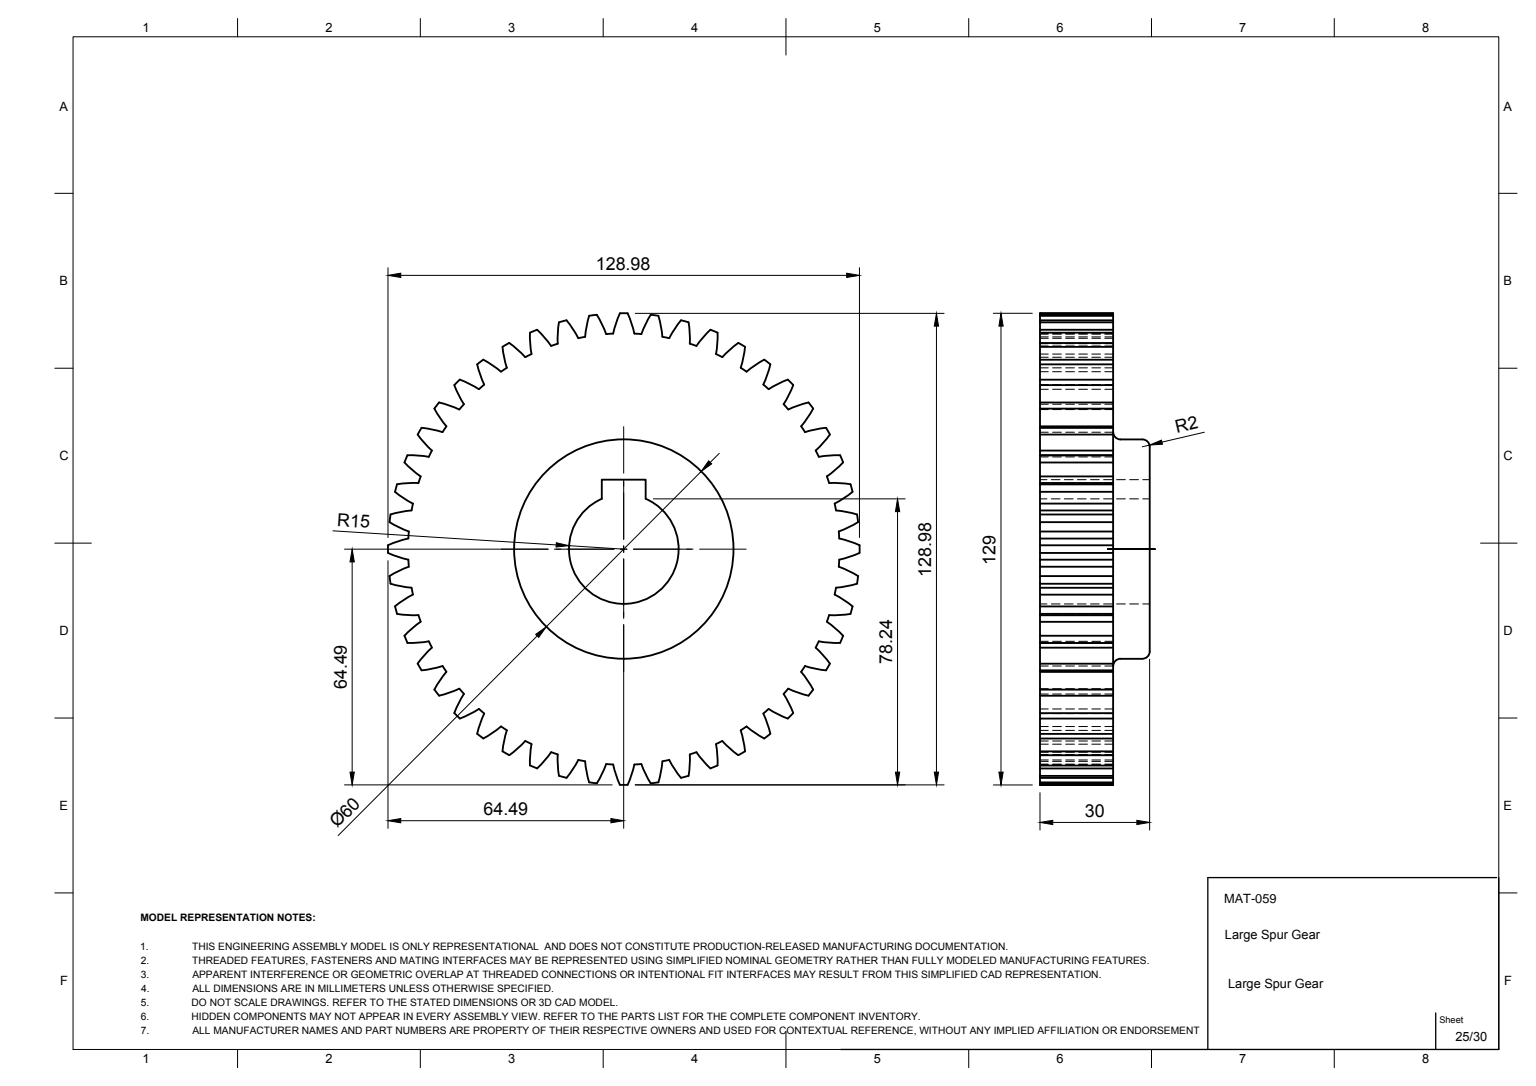
ISO-10303-21;
HEADER;
/* Generated by software containing ST-Developer
 * from STEP Tools, Inc. (www.steptools.com) 
 */

FILE_DESCRIPTION(
/* description */ ('', 'CAx-IF Rec.Pracs.---Representation and Presentation of Product Manufa
cturing Information (PMI)---4.0---2014-10-13'),
/* implementation_level */ '2;1');

FILE_NAME(
/* name */ 'Large Spur Gear.step',
/* time_stamp */ '2026-10-28T23:00:48+01:00',
/* author */ (''),
/* organization */ (''),
/* preprocessor_version */ 'ST-DEVELOPER v20.2',
/* originating_system */ 'Autodesk Translation Framework v15.17.0.0',
/* authorisation */ '');

FILE_SCHEMA (('AP242_MANAGED_MODEL_BASED_3D_ENGINEERING_MIM_LF { 1 0 10303 442 2 1 4 }'));
ENDSEC;

DATA;
#10=MECHANICAL_DESIGN_GEOMETRIC_PRESENTATION_REPRESENTATION('',(#996),#61811);
#906=TOROIDAL_SURFACE('',#36149,28.,2.);
#907=TOROIDAL_SURFACE('',#36158,32.,2.);
#932=SHAPE_REPRESENTATION_RELATIONSHIP('SRR','None',#61993,#957);
#957=ADVANCED_BREP_SHAPE_REPRESENTATION('',(#1035),#61806);
#996=STYLED_ITEM('',(#62149),#1035);
#1035=MANIFOLD_SOLID_BREP('Body1',#33826);
#1395=CYLINDRICAL_SURFACE('',#36154,30.);
#1396=CYLINDRICAL_SURFACE('',#36356,15.);
#1397=CYLINDRICAL_SURFACE('',#36359,59.00430282);
#1398=CYLINDRICAL_SURFACE('',#36361,28.3018268963564);
#1399=CYLINDRICAL_SURFACE('',#36363,28.3018268963564);
#1400=CYLINDRICAL_SURFACE('',#36365,59.00430282);
#1401=CYLINDRICAL_SURFACE('',#36367,28.3018268963564);
#1402=CYLINDRICAL_SURFACE('',#36369,28.3018268963564);
#1403=CYLINDRICAL_SURFACE('',#36371,59.00430282);
#1404=CYLINDRICAL_SURFACE('',#36373,28.3018268963564);
#1405=CYLINDRICAL_SURFACE('',#36375,28.3018268963564);
#1406=CYLINDRICAL_SURFACE('',#36377,59.00430282);
#1407=CYLINDRICAL_SURFACE('',#36379,28.3018268963564);
#1408=CYLINDRICAL_SURFACE('',#36381,28.3018268963564);
#1409=CYLINDRICAL_SURFACE('',#36383,59.00430282);
#1410=CYLINDRICAL_SURFACE('',#36385,28.3018268963564);
#1411=CYLINDRICAL_SURFACE('',#36387,28.3018268963564);
#1412=CYLINDRICAL_SURFACE('',#36389,59.00430282);
#1413=CYLINDRICAL_SURFACE('',#36391,28.3018268963564);
#1414=CYLINDRICAL_SURFACE('',#36393,28.3018268963564);
#1415=CYLINDRICAL_SURFACE('',#36395,59.00430282);
#1416=CYLINDRICAL_SURFACE('',#36397,28.3018268963564);
#1417=CYLINDRICAL_SURFACE('',#36399,28.3018268963564);
#1418=CYLINDRICAL_SURFACE('',#36401,59.00430282);
#1419=CYLINDRICAL_SURFACE('',#36403,28.3018268963564);
#1420=CYLINDRICAL_SURFACE('',#36405,28.3018268963564);
#1421=CYLINDRICAL_SURFACE('',#36407,59.00430282);
#1422=CYLINDRICAL_SURFACE('',#36409,28.3018268963564);
#1423=CYLINDRICAL_SURFACE('',#36411,28.3018268963564);
#1424=CYLINDRICAL_SURFACE('',#36413,59.00430282);
#1425=CYLINDRICAL_SURFACE('',#36415,28.3018268963564);
#1426=CYLINDRICAL_SURFACE('',#36417,28.3018268963564);
#1427=CYLINDRICAL_SURFACE('',#36419,59.00430282);
#1428=CYLINDRICAL_SURFACE('',#36421,28.3018268963564);
#1429=CYLINDRICAL_SURFACE('',#36423,28.3018268963564);
#1430=CYLINDRICAL_SURFACE('',#36425,59.00430282);
#1431=CYLINDRICAL_SURFACE('',#36427,28.3018268963564);
#1432=CYLINDRICAL_SURFACE('',#36429,28.3018268963564);
#1433=CYLINDRICAL_SURFACE('',#36431,59.00430282);
#1434=CYLINDRICAL_SURFACE('',#36433,28.3018268963564);
#1435=CYLINDRICAL_SURFACE('',#36435,28.3018268963564);
#1436=CYLINDRICAL_SURFACE('',#36437,59.00430282);
#1437=CYLINDRICAL_SURFACE('',#36439,28.3018268963564);
#1438=CYLINDRICAL_SURFACE('',#36441,28.3018268963564);
#1439=CYLINDRICAL_SURFACE('',#36443,59.00430282);
#1440=CYLINDRICAL_SURFACE('',#36445,28.3018268963564);
#1441=CYLINDRICAL_SURFACE('',#36447,28.3018268963564);
#1442=CYLINDRICAL_SURFACE('',#36449,59.00430282);
#1443=CYLINDRICAL_SURFACE('',#36451,28.3018268963564);
#1444=CYLINDRICAL_SURFACE('',#36453,28.3018268963564);
#1445=CYLINDRICAL_SURFACE('',#36455,59.00430282);
#1446=CYLINDRICAL_SURFACE('',#36457,28.3018268963564);
#1447=CYLINDRICAL_SURFACE('',#36459,28.3018268963564);
#1448=CYLINDRICAL_SURFACE('',#36461,59.00430282);
#1449=CYLINDRICAL_SURFACE('',#36463,28.3018268963564);
#1450=CYLINDRICAL_SURFACE('',#36465,28.3018268963564);
#1451=CYLINDRICAL_SURFACE('',#36467,59.00430282);
#1452=CYLINDRICAL_SURFACE('',#36469,28.3018268963564);
#1453=CYLINDRICAL_SURFACE('',#36471,28.3018268963564);
#1454=CYLINDRICAL_SURFACE('',#36473,59.00430282);
#1455=CYLINDRICAL_SURFACE('',#36475,28.3018268963564);
#1456=CYLINDRICAL_SURFACE('',#36477,28.3018268963564);
#1457=CYLINDRICAL_SURFACE('',#36479,59.00430282);
#1458=CYLINDRICAL_SURFACE('',#36481,28.3018268963564);
#1459=CYLINDRICAL_SURFACE('',#36483,28.3018268963564);
#1460=CYLINDRICAL_SURFACE('',#36485,59.00430282);
#1461=CYLINDRICAL_SURFACE('',#36487,28.3018268963564);
#1462=CYLINDRICAL_SURFACE('',#36489,28.3018268963564);
#1463=CYLINDRICAL_SURFACE('',#36491,59.00430282);
#1464=CYLINDRICAL_SURFACE('',#36493,28.3018268963564);
#1465=CYLINDRICAL_SURFACE('',#36495,28.3018268963564);
#1466=CYLINDRICAL_SURFACE('',#36497,59.00430282);
#1467=CYLINDRICAL_SURFACE('',#36499,28.3018268963564);
#1468=CYLINDRICAL_SURFACE('',#36501,28.3018268963564);
#1469=CYLINDRICAL_SURFACE('',#36503,59.00430282);
#1470=CYLINDRICAL_SURFACE('',#36505,28.3018268963564);
#1471=CYLINDRICAL_SURFACE('',#36507,28.3018268963564);
#1472=CYLINDRICAL_SURFACE('',#36509,59.00430282);
#1473=CYLINDRICAL_SURFACE('',#36511,28.3018268963564);
#1474=CYLINDRICAL_SURFACE('',#36513,28.3018268963564);
#1475=CYLINDRICAL_SURFACE('',#36515,59.00430282);
#1476=CYLINDRICAL_SURFACE('',#36517,28.3018268963564);
#1477=CYLINDRICAL_SURFACE('',#36519,28.3018268963564);
#1478=CYLINDRICAL_SURFACE('',#36521,59.00430282);
#1479=CYLINDRICAL_SURFACE('',#36523,28.3018268963564);
#1480=CYLINDRICAL_SURFACE('',#36525,28.3018268963564);
#1481=CYLINDRICAL_SURFACE('',#36527,59.00430282);
#1482=CYLINDRICAL_SURFACE('',#36529,28.3018268963564);
#1483=CYLINDRICAL_SURFACE('',#36531,28.3018268963564);
#1484=CYLINDRICAL_SURFACE('',#36533,59.00430282);
#1485=CYLINDRICAL_SURFACE('',#36535,28.3018268963564);
#1486=CYLINDRICAL_SURFACE('',#36537,28.3018268963564);
#1487=CYLINDRICAL_SURFACE('',#36539,59.00430282);
#1488=CYLINDRICAL_SURFACE('',#36541,28.3018268963564);
#1489=CYLINDRICAL_SURFACE('',#36543,28.3018268963564);
#1490=CYLINDRICAL_SURFACE('',#36545,59.00430282);
#1491=CYLINDRICAL_SURFACE('',#36547,28.3018268963564);
#1492=CYLINDRICAL_SURFACE('',#36549,28.3018268963564);
#1493=CYLINDRICAL_SURFACE('',#36551,59.00430282);
#1494=CYLINDRICAL_SURFACE('',#36553,28.3018268963564);
#1495=CYLINDRICAL_SURFACE('',#36555,28.3018268963564);
#1496=CYLINDRICAL_SURFACE('',#36557,59.00430282);
#1497=CYLINDRICAL_SURFACE('',#36559,28.3018268963564);
#1498=CYLINDRICAL_SURFACE('',#36561,28.3018268963564);
#1499=CYLINDRICAL_SURFACE('',#36563,59.00430282);
#1500=CYLINDRICAL_SURFACE('',#36565,28.3018268963564);
#1501=CYLINDRICAL_SURFACE('',#36567,28.3018268963564);
#1502=CYLINDRICAL_SURFACE('',#36569,59.00430282);
#1503=CYLINDRICAL_SURFACE('',#36571,28.3018268963564);
#1504=CYLINDRICAL_SURFACE('',#36573,28.3018268963564);
#1505=CYLINDRICAL_SURFACE('',#36575,59.00430282);
#1506=CYLINDRICAL_SURFACE('',#36577,28.3018268963564);
#1507=CYLINDRICAL_SURFACE('',#36579,28.3018268963564);
#1508=CYLINDRICAL_SURFACE('',#36581,59.00430282);
#1509=CYLINDRICAL_SURFACE('',#36583,28.3018268963564);
#1510=CYLINDRICAL_SURFACE('',#36585,28.3018268963564);
#1511=CYLINDRICAL_SURFACE('',#36587,59.00430282);
#1512=CYLINDRICAL_SURFACE('',#36589,28.3018268963564);
#1513=CYLINDRICAL_SURFACE('',#36591,28.3018268963564);
#1514=CYLINDRICAL_SURFACE('',#36593,59.00430282);
#1515=CYLINDRICAL_SURFACE('',#36595,28.3018268963564);
#1516=CYLINDRICAL_SURFACE('',#36597,28.3018268963564);
#1517=CYLINDRICAL_SURFACE('',#36599,59.00430282);
#1518=CYLINDRICAL_SURFACE('',#36601,28.3018268963564);
#1519=CYLINDRICAL_SURFACE('',#36603,28.3018268963564);
#1520=CYLINDRICAL_SURFACE('',#36605,59.00430282);
#1521=CYLINDRICAL_SURFACE('',#36607,28.3018268963564);
#1522=CYLINDRICAL_SURFACE('',#36609,28.3018268963564);
#1523=CYLINDRICAL_SURFACE('',#36611,59.00430282);
#1524=CYLINDRICAL_SURFACE('',#36613,28.3018268963564);
#1525=CYLINDRICAL_SURFACE('',#36615,28.3018268963564);
#1526=CYLINDRICAL_SURFACE('',#36617,59.00430282);
#1527=CYLINDRICAL_SURFACE('',#36619,28.3018268963564);
#1528=CYLINDRICAL_SURFACE('',#36621,28.3018268963564);
#1529=CYLINDRICAL_SURFACE('',#36623,59.00430282);
#1530=CYLINDRICAL_SURFACE('',#36625,28.3018268963564);
#1531=CYLINDRICAL_SURFACE('',#36627,28.3018268963564);
#1532=CYLINDRICAL_SURFACE('',#36629,59.00430282);
#1533=CYLINDRICAL_SURFACE('',#36631,28.3018268963564);
#1534=CYLINDRICAL_SURFACE('',#36633,28.3018268963564);
#1535=CYLINDRICAL_SURFACE('',#36635,59.00430282);
#1536=CYLINDRICAL_SURFACE('',#36637,28.3018268963564);
#1537=CYLINDRICAL_SURFACE('',#36639,28.3018268963564);
#1538=CYLINDRICAL_SURFACE('',#36641,64.5);
#1539=CYLINDRICAL_SURFACE('',#36643,64.5);
#1540=CYLINDRICAL_SURFACE('',#36645,64.5);
#1541=CYLINDRICAL_SURFACE('',#36647,64.5);
#1542=CYLINDRICAL_SURFACE('',#36649,64.5);
#1543=CYLINDRICAL_SURFACE('',#36651,64.5);
#1544=CYLINDRICAL_SURFACE('',#36653,64.5);
#1545=CYLINDRICAL_SURFACE('',#36655,64.5);
#1546=CYLINDRICAL_SURFACE('',#36657,64.5);
#1547=CYLINDRICAL_SURFACE('',#36659,64.5);
#1548=CYLINDRICAL_SURFACE('',#36661,64.5);
#1549=CYLINDRICAL_SURFACE('',#36663,64.5);
#1550=CYLINDRICAL_SURFACE('',#36665,64.5);
#1551=CYLINDRICAL_SURFACE('',#36667,64.5);
#1552=CYLINDRICAL_SURFACE('',#36669,64.5);
#1553=CYLINDRICAL_SURFACE('',#36671,64.5);
#1554=CYLINDRICAL_SURFACE('',#36673,64.5);
#1555=CYLINDRICAL_SURFACE('',#36675,64.5);
#1556=CYLINDRICAL_SURFACE('',#36677,64.5);
#1557=CYLINDRICAL_SURFACE('',#36679,64.5);
#1558=CYLINDRICAL_SURFACE('',#36681,64.5);
#1559=CYLINDRICAL_SURFACE('',#36683,64.5);
#1560=CYLINDRICAL_SURFACE('',#36685,64.5);
#1561=CYLINDRICAL_SURFACE('',#36687,64.5);
#1562=CYLINDRICAL_SURFACE('',#36689,64.5);
#1563=CYLINDRICAL_SURFACE('',#36691,64.5);
#1564=CYLINDRICAL_SURFACE('',#36693,64.5);
#1565=CYLINDRICAL_SURFACE('',#36695,64.5);
#1566=CYLINDRICAL_SURFACE('',#36697,64.5);
#1567=CYLINDRICAL_SURFACE('',#36699,64.5);
#1568=CYLINDRICAL_SURFACE('',#36701,64.5);
#1569=CYLINDRICAL_SURFACE('',#36703,64.5);
#1570=CYLINDRICAL_SURFACE('',#36705,64.5);
#1571=CYLINDRICAL_SURFACE('',#36707,64.5);
#1572=CYLINDRICAL_SURFACE('',#36709,64.5);
#1573=CYLINDRICAL_SURFACE('',#36711,64.5);
#1574=CYLINDRICAL_SURFACE('',#36713,64.5);
#1575=CYLINDRICAL_SURFACE('',#36715,64.5);
#1576=CYLINDRICAL_SURFACE('',#36717,64.5);
#1577=CYLINDRICAL_SURFACE('',#36719,64.5);
#1578=CYLINDRICAL_SURFACE('',#36721,64.5);
#1579=CYLINDRICAL_SURFACE('',#36723,64.5);
#1580=CYLINDRICAL_SURFACE('',#36725,64.5);
#1581=CYLINDRICAL_SURFACE('',#36727,64.5);
#1582=CYLINDRICAL_SURFACE('',#36729,64.5);
#1583=CYLINDRICAL_SURFACE('',#36731,64.5);
#1584=CYLINDRICAL_SURFACE('',#36733,64.5);
#1585=CYLINDRICAL_SURFACE('',#36735,59.00430282);
#1586=CYLINDRICAL_SURFACE('',#36737,28.3018268963564);
#1587=CYLINDRICAL_SURFACE('',#36739,28.3018268963564);
#1588=CYLINDRICAL_SURFACE('',#36741,64.5);
#2131=FACE_BOUND('',#7406,.T.);
#2132=FACE_BOUND('',#7409,.T.);
#2133=FACE_BOUND('',#7607,.T.);
#3125=CIRCLE('',#36150,28.);
#3126=CIRCLE('',#36151,2.);
#3127=CIRCLE('',#36152,30.);
#3128=CIRCLE('',#36153,30.);
#3129=CIRCLE('',#36155,30.);
#3130=CIRCLE('',#36157,15.);
#3131=CIRCLE('',#36159,32.);
#3132=CIRCLE('',#36160,2.);
#3133=CIRCLE('',#36162,28.3018268963564);
#3134=CIRCLE('',#36163,59.00430282);
#3135=CIRCLE('',#36164,28.3018268963564);
#3136=CIRCLE('',#36165,64.5);
#3137=CIRCLE('',#36166,28.3018268963564);
#3138=CIRCLE('',#36167,59.00430282);
#3139=CIRCLE('',#36168,28.3018268963564);
#3140=CIRCLE('',#36169,64.5);
#3141=CIRCLE('',#36170,28.3018268963564);
#3142=CIRCLE('',#36171,59.00430282);
#3143=CIRCLE('',#36172,28.3018268963564);
#3144=CIRCLE('',#36173,64.5);
#3145=CIRCLE('',#36174,28.3018268963564);
#3146=CIRCLE('',#36175,59.00430282);
#3147=CIRCLE('',#36176,28.3018268963564);
#3148=CIRCLE('',#36177,64.5);
#3149=CIRCLE('',#36178,28.3018268963564);
#3150=CIRCLE('',#36179,59.00430282);
#3151=CIRCLE('',#36180,28.3018268963564);
#3152=CIRCLE('',#36181,64.5);
#3153=CIRCLE('',#36182,28.3018268963564);
#3154=CIRCLE('',#36183,59.00430282);
#3155=CIRCLE('',#36184,28.3018268963564);
#3156=CIRCLE('',#36185,64.5);
#3157=CIRCLE('',#36186,28.3018268963564);
#3158=CIRCLE('',#36187,59.00430282);
#3159=CIRCLE('',#36188,28.3018268963564);
#3160=CIRCLE('',#36189,64.5);
#3161=CIRCLE('',#36190,28.3018268963564);
#3162=CIRCLE('',#36191,59.00430282);
#3163=CIRCLE('',#36192,28.3018268963564);
#3164=CIRCLE('',#36193,64.5);
#3165=CIRCLE('',#36194,28.3018268963564);
#3166=CIRCLE('',#36195,59.00430282);
#3167=CIRCLE('',#36196,28.3018268963564);
#3168=CIRCLE('',#36197,64.5);
#3169=CIRCLE('',#36198,28.3018268963564);
#3170=CIRCLE('',#36199,59.00430282);
#3171=CIRCLE('',#36200,28.3018268963564);
#3172=CIRCLE('',#36201,64.5);
#3173=CIRCLE('',#36202,28.3018268963564);
#3174=CIRCLE('',#36203,59.00430282);
#3175=CIRCLE('',#36204,28.3018268963564);
#3176=CIRCLE('',#36205,64.5);
#3177=CIRCLE('',#36206,28.3018268963564);
#3178=CIRCLE('',#36207,59.00430282);
#3179=CIRCLE('',#36208,28.3018268963564);
#3180=CIRCLE('',#36209,64.5);
#3181=CIRCLE('',#36210,28.3018268963564);
#3182=CIRCLE('',#36211,59.00430282);
#3183=CIRCLE('',#36212,28.3018268963564);
#3184=CIRCLE('',#36213,64.5);
#3185=CIRCLE('',#36214,28.3018268963564);
#3186=CIRCLE('',#36215,59.00430282);
#3187=CIRCLE('',#36216,28.3018268963564);
#3188=CIRCLE('',#36217,64.5);
#3189=CIRCLE('',#36218,28.3018268963564);
#3190=CIRCLE('',#36219,59.00430282);
#3191=CIRCLE('',#36220,28.3018268963564);
#3192=CIRCLE('',#36221,64.5);
#3193=CIRCLE('',#36222,28.3018268963564);
#3194=CIRCLE('',#36223,59.00430282);
#3195=CIRCLE('',#36224,28.3018268963564);
#3196=CIRCLE('',#36225,64.5);
#3197=CIRCLE('',#36226,28.3018268963564);
#3198=CIRCLE('',#36227,59.00430282);
#3199=CIRCLE('',#36228,28.3018268963564);
#3200=CIRCLE('',#36229,64.5);
#3201=CIRCLE('',#36230,28.3018268963564);
#3202=CIRCLE('',#36231,59.00430282);
#3203=CIRCLE('',#36232,28.3018268963564);
#3204=CIRCLE('',#36233,64.5);
#3205=CIRCLE('',#36234,28.3018268963564);
#3206=CIRCLE('',#36235,59.00430282);
#3207=CIRCLE('',#36236,28.3018268963564);
#3208=CIRCLE('',#36237,64.5);
#3209=CIRCLE('',#36238,28.3018268963564);
#3210=CIRCLE('',#36239,59.00430282);
#3211=CIRCLE('',#36240,28.3018268963564);
#3212=CIRCLE('',#36241,64.5);
#3213=CIRCLE('',#36242,28.3018268963564);
#3214=CIRCLE('',#36243,59.00430282);
#3215=CIRCLE('',#36244,28.3018268963564);
#3216=CIRCLE('',#36245,64.5);
#3217=CIRCLE('',#36246,28.3018268963564);
#3218=CIRCLE('',#36247,59.00430282);
#3219=CIRCLE('',#36248,28.3018268963564);
#3220=CIRCLE('',#36249,64.5);
#3221=CIRCLE('',#36250,28.3018268963564);
#3222=CIRCLE('',#36251,59.00430282);
#3223=CIRCLE('',#36252,28.3018268963564);
#3224=CIRCLE('',#36253,64.5);
#3225=CIRCLE('',#36254,28.3018268963564);
#3226=CIRCLE('',#36255,59.00430282);
#3227=CIRCLE('',#36256,28.3018268963564);
#3228=CIRCLE('',#36257,64.5);
#3229=CIRCLE('',#36258,28.3018268963564);
#3230=CIRCLE('',#36259,59.00430282);
#3231=CIRCLE('',#36260,28.3018268963564);
#3232=CIRCLE('',#36261,64.5);
#3233=CIRCLE('',#36262,28.3018268963564);
#3234=CIRCLE('',#36263,59.00430282);
#3235=CIRCLE('',#36264,28.3018268963564);
#3236=CIRCLE('',#36265,64.5);
#3237=CIRCLE('',#36266,28.3018268963564);
#3238=CIRCLE('',#36267,59.00430282);
#3239=CIRCLE('',#36268,28.3018268963564);
#3240=CIRCLE('',#36269,64.5);
#3241=CIRCLE('',#36270,28.3018268963564);
#3242=CIRCLE('',#36271,59.00430282);
#3243=CIRCLE('',#36272,28.3018268963564);
#3244=CIRCLE('',#36273,64.5);
#3245=CIRCLE('',#36274,28.3018268963564);
#3246=CIRCLE('',#36275,59.00430282);
#3247=CIRCLE('',#36276,28.3018268963564);
#3248=CIRCLE('',#36277,64.5);
#3249=CIRCLE('',#36278,28.3018268963564);
#3250=CIRCLE('',#36279,59.00430282);
#3251=CIRCLE('',#36280,28.3018268963564);
#3252=CIRCLE('',#36281,64.5);
#3253=CIRCLE('',#36282,28.3018268963564);
#3254=CIRCLE('',#36283,59.00430282);
#3255=CIRCLE('',#36284,28.3018268963564);
#3256=CIRCLE('',#36285,64.5);
#3257=CIRCLE('',#36286,28.3018268963564);
#3258=CIRCLE('',#36287,59.00430282);
#3259=CIRCLE('',#36288,28.3018268963564);
#3260=CIRCLE('',#36289,64.5);
#3261=CIRCLE('',#36290,28.3018268963564);
#3262=CIRCLE('',#36291,59.00430282);
#3263=CIRCLE('',#36292,28.3018268963564);
#3264=CIRCLE('',#36293,64.5);
#3265=CIRCLE('',#36294,28.3018268963564);
#3266=CIRCLE('',#36295,59.00430282);
#3267=CIRCLE('',#36296,28.3018268963564);
#3268=CIRCLE('',#36297,64.5);
#3269=CIRCLE('',#36298,28.3018268963564);
#3270=CIRCLE('',#36299,59.00430282);
#3271=CIRCLE('',#36300,28.3018268963564);
#3272=CIRCLE('',#36301,64.5);
#3273=CIRCLE('',#36302,28.3018268963564);
#3274=CIRCLE('',#36303,59.00430282);
#3275=CIRCLE('',#36304,28.3018268963564);
#3276=CIRCLE('',#36305,64.5);
#3277=CIRCLE('',#36306,28.3018268963564);
#3278=CIRCLE('',#36307,59.00430282);
#3279=CIRCLE('',#36308,28.3018268963564);
#3280=CIRCLE('',#36309,64.5);
#3281=CIRCLE('',#36310,28.3018268963564);
#3282=CIRCLE('',#36311,59.00430282);
#3283=CIRCLE('',#36312,28.3018268963564);
#3284=CIRCLE('',#36313,64.5);
#3285=CIRCLE('',#36314,28.3018268963564);
#3286=CIRCLE('',#36315,59.00430282);
#3287=CIRCLE('',#36316,28.3018268963564);
#3288=CIRCLE('',#36317,64.5);
#3289=CIRCLE('',#36318,28.3018268963564);
#3290=CIRCLE('',#36319,59.00430282);
#3291=CIRCLE('',#36320,28.3018268963564);
#3292=CIRCLE('',#36321,64.5);
#3293=CIRCLE('',#36322,28.3018268963564);
#3294=CIRCLE('',#36323,59.00430282);
#3295=CIRCLE('',#36324,28.3018268963564);
#3296=CIRCLE('',#36325,64.5);
#3297=CIRCLE('',#36326,28.3018268963564);
#3298=CIRCLE('',#36327,59.00430282);
#3299=CIRCLE('',#36328,28.3018268963564);
#3300=CIRCLE('',#36329,64.5);
#3301=CIRCLE('',#36330,28.3018268963564);
#3302=CIRCLE('',#36331,59.00430282);
#3303=CIRCLE('',#36332,28.3018268963564);
#3304=CIRCLE('',#36333,64.5);
#3305=CIRCLE('',#36334,28.3018268963564);
#3306=CIRCLE('',#36335,59.00430282);
#3307=CIRCLE('',#36336,28.3018268963564);
#3308=CIRCLE('',#36337,64.5);
#3309=CIRCLE('',#36338,28.3018268963564);
#3310=CIRCLE('',#36339,59.00430282);
#3311=CIRCLE('',#36340,28.3018268963564);
#3312=CIRCLE('',#36341,64.5);
#3313=CIRCLE('',#36342,28.3018268963564);
#3314=CIRCLE('',#36343,59.00430282);
#3315=CIRCLE('',#36344,28.3018268963564);
#3316=CIRCLE('',#36345,64.5);
#3317=CIRCLE('',#36346,28.3018268963564);
#3318=CIRCLE('',#36347,59.00430282);
#3319=CIRCLE('',#36348,28.3018268963564);
#3320=CIRCLE('',#36349,64.5);
#3321=CIRCLE('',#36350,28.3018268963564);
#3322=CIRCLE('',#36351,59.00430282);
#3323=CIRCLE('',#36352,28.3018268963564);
#3324=CIRCLE('',#36353,64.5);
#3325=CIRCLE('',#36357,15.);
#3326=CIRCLE('',#36360,59.00430282);
#3327=CIRCLE('',#36362,28.3018268963564);
#3328=CIRCLE('',#36364,28.3018268963564);
#3329=CIRCLE('',#36366,59.00430282);
#3330=CIRCLE('',#36368,28.3018268963564);
#3331=CIRCLE('',#36370,28.3018268963564);
#3332=CIRCLE('',#36372,59.00430282);
#3333=CIRCLE('',#36374,28.3018268963564);
#3334=CIRCLE('',#36376,28.3018268963564);
#3335=CIRCLE('',#36378,59.00430282);
#3336=CIRCLE('',#36380,28.3018268963564);
#3337=CIRCLE('',#36382,28.3018268963564);
#3338=CIRCLE('',#36384,59.00430282);
#3339=CIRCLE('',#36386,28.3018268963564);
#3340=CIRCLE('',#36388,28.3018268963564);
#3341=CIRCLE('',#36390,59.00430282);
#3342=CIRCLE('',#36392,28.3018268963564);
#3343=CIRCLE('',#36394,28.3018268963564);
#3344=CIRCLE('',#36396,59.00430282);
#3345=CIRCLE('',#36398,28.3018268963564);
#3346=CIRCLE('',#36400,28.3018268963564);
#3347=CIRCLE('',#36402,59.00430282);
#3348=CIRCLE('',#36404,28.3018268963564);
#3349=CIRCLE('',#36406,28.3018268963564);
#3350=CIRCLE('',#36408,59.00430282);
#3351=CIRCLE('',#36410,28.3018268963564);
#3352=CIRCLE('',#36412,28.3018268963564);
#3353=CIRCLE('',#36414,59.00430282);
#3354=CIRCLE('',#36416,28.3018268963564);
#3355=CIRCLE('',#36418,28.3018268963564);
#3356=CIRCLE('',#36420,59.00430282);
#3357=CIRCLE('',#36422,28.3018268963564);
#3358=CIRCLE('',#36424,28.3018268963564);
#3359=CIRCLE('',#36426,59.00430282);
#3360=CIRCLE('',#36428,28.3018268963564);
#3361=CIRCLE('',#36430,28.3018268963564);
#3362=CIRCLE('',#36432,59.00430282);
#3363=CIRCLE('',#36434,28.3018268963564);
#3364=CIRCLE('',#36436,28.3018268963564);
#3365=CIRCLE('',#36438,59.00430282);
#3366=CIRCLE('',#36440,28.3018268963564);
#3367=CIRCLE('',#36442,28.3018268963564);
#3368=CIRCLE('',#36444,59.00430282);
#3369=CIRCLE('',#36446,28.3018268963564);
#3370=CIRCLE('',#36448,28.3018268963564);
#3371=CIRCLE('',#36450,59.00430282);
#3372=CIRCLE('',#36452,28.3018268963564);
#3373=CIRCLE('',#36454,28.3018268963564);
#3374=CIRCLE('',#36456,59.00430282);
#3375=CIRCLE('',#36458,28.3018268963564);
#3376=CIRCLE('',#36460,28.3018268963564);
#3377=CIRCLE('',#36462,59.00430282);
#3378=CIRCLE('',#36464,28.3018268963564);
#3379=CIRCLE('',#36466,28.3018268963564);
#3380=CIRCLE('',#36468,59.00430282);
#3381=CIRCLE('',#36470,28.3018268963564);
#3382=CIRCLE('',#36472,28.3018268963564);
#3383=CIRCLE('',#36474,59.00430282);
#3384=CIRCLE('',#36476,28.3018268963564);
#3385=CIRCLE('',#36478,28.3018268963564);
#3386=CIRCLE('',#36480,59.00430282);
#3387=CIRCLE('',#36482,28.3018268963564);
#3388=CIRCLE('',#36484,28.3018268963564);
#3389=CIRCLE('',#36486,59.00430282);
#3390=CIRCLE('',#36488,28.3018268963564);
#3391=CIRCLE('',#36490,28.3018268963564);
#3392=CIRCLE('',#36492,59.00430282);
#3393=CIRCLE('',#36494,28.3018268963564);
#3394=CIRCLE('',#36496,28.3018268963564);
#3395=CIRCLE('',#36498,59.00430282);
#3396=CIRCLE('',#36500,28.3018268963564);
#3397=CIRCLE('',#36502,28.3018268963564);
#3398=CIRCLE('',#36504,59.00430282);
#3399=CIRCLE('',#36506,28.3018268963564);
#3400=CIRCLE('',#36508,28.3018268963564);
#3401=CIRCLE('',#36510,59.00430282);
#3402=CIRCLE('',#36512,28.3018268963564);
#3403=CIRCLE('',#36514,28.3018268963564);
#3404=CIRCLE('',#36516,59.00430282);
#3405=CIRCLE('',#36518,28.3018268963564);
#3406=CIRCLE('',#36520,28.3018268963564);
#3407=CIRCLE('',#36522,59.00430282);
#3408=CIRCLE('',#36524,28.3018268963564);
#3409=CIRCLE('',#36526,28.3018268963564);
#3410=CIRCLE('',#36528,59.00430282);
#3411=CIRCLE('',#36530,28.3018268963564);
#3412=CIRCLE('',#36532,28.3018268963564);
#3413=CIRCLE('',#36534,59.00430282);
#3414=CIRCLE('',#36536,28.3018268963564);
#3415=CIRCLE('',#36538,28.3018268963564);
#3416=CIRCLE('',#36540,59.00430282);
#3417=CIRCLE('',#36542,28.3018268963564);
#3418=CIRCLE('',#36544,28.3018268963564);
#3419=CIRCLE('',#36546,59.00430282);
#3420=CIRCLE('',#36548,28.3018268963564);
#3421=CIRCLE('',#36550,28.3018268963564);
#3422=CIRCLE('',#36552,59.00430282);
#3423=CIRCLE('',#36554,28.3018268963564);
#3424=CIRCLE('',#36556,28.3018268963564);
#3425=CIRCLE('',#36558,59.00430282);
#3426=CIRCLE('',#36560,28.3018268963564);
#3427=CIRCLE('',#36562,28.3018268963564);
#3428=CIRCLE('',#36564,59.00430282);
#3429=CIRCLE('',#36566,28.3018268963564);
#3430=CIRCLE('',#36568,28.3018268963564);
#3431=CIRCLE('',#36570,59.00430282);
#3432=CIRCLE('',#36572,28.3018268963564);
#3433=CIRCLE('',#36574,28.3018268963564);
#3434=CIRCLE('',#36576,59.00430282);
#3435=CIRCLE('',#36578,28.3018268963564);
#3436=CIRCLE('',#36580,28.3018268963564);
#3437=CIRCLE('',#36582,59.00430282);
#3438=CIRCLE('',#36584,28.3018268963564);
#3439=CIRCLE('',#36586,28.3018268963564);
#3440=CIRCLE('',#36588,59.00430282);
#3441=CIRCLE('',#36590,28.3018268963564);
#3442=CIRCLE('',#36592,28.3018268963564);
#3443=CIRCLE('',#36594,59.00430282);
#3444=CIRCLE('',#36596,28.3018268963564);
#3445=CIRCLE('',#36598,28.3018268963564);
#3446=CIRCLE('',#36600,59.00430282);
#3447=CIRCLE('',#36602,28.3018268963564);
#3448=CIRCLE('',#36604,28.3018268963564);
#3449=CIRCLE('',#36606,59.00430282);
#3450=CIRCLE('',#36608,28.3018268963564);
#3451=CIRCLE('',#36610,28.3018268963564);
#3452=CIRCLE('',#36612,59.00430282);
#3453=CIRCLE('',#36614,28.3018268963564);
#3454=CIRCLE('',#36616,28.3018268963564);
#3455=CIRCLE('',#36618,59.00430282);
#3456=CIRCLE('',#36620,28.3018268963564);
#3457=CIRCLE('',#36622,28.3018268963564);
#3458=CIRCLE('',#36624,59.00430282);
#3459=CIRCLE('',#36626,28.3018268963564);
#3460=CIRCLE('',#36628,28.3018268963564);
#3461=CIRCLE('',#36630,59.00430282);
#3462=CIRCLE('',#36632,28.3018268963564);
#3463=CIRCLE('',#36634,28.3018268963564);
#3464=CIRCLE('',#36636,59.00430282);
#3465=CIRCLE('',#36638,28.3018268963564);
#3466=CIRCLE('',#36640,28.3018268963564);
#3467=CIRCLE('',#36642,64.5);
#3468=CIRCLE('',#36644,64.5);
#3469=CIRCLE('',#36646,64.5);
#3470=CIRCLE('',#36648,64.5);
#3471=CIRCLE('',#36650,64.5);
#3472=CIRCLE('',#36652,64.5);
#3473=CIRCLE('',#36654,64.5);
#3474=CIRCLE('',#36656,64.5);
#3475=CIRCLE('',#36658,64.5);
#3476=CIRCLE('',#36660,64.5);
#3477=CIRCLE('',#36662,64.5);
#3478=CIRCLE('',#36664,64.5);
#3479=CIRCLE('',#36666,64.5);
#3480=CIRCLE('',#36668,64.5);
#3481=CIRCLE('',#36670,64.5);
#3482=CIRCLE('',#36672,64.5);
#3483=CIRCLE('',#36674,64.5);
#3484=CIRCLE('',#36676,64.5);
#3485=CIRCLE('',#36678,64.5);
#3486=CIRCLE('',#36680,64.5);
#3487=CIRCLE('',#36682,64.5);
#3488=CIRCLE('',#36684,64.5);
#3489=CIRCLE('',#36686,64.5);
#3490=CIRCLE('',#36688,64.5);
#3491=CIRCLE('',#36690,64.5);
#3492=CIRCLE('',#36692,64.5);
#3493=CIRCLE('',#36694,64.5);
#3494=CIRCLE('',#36696,64.5);
#3495=CIRCLE('',#36698,64.5);
#3496=CIRCLE('',#36700,64.5);
#3497=CIRCLE('',#36702,64.5);
#3498=CIRCLE('',#36704,64.5);
#3499=CIRCLE('',#36706,64.5);
#3500=CIRCLE('',#36708,64.5);
#3501=CIRCLE('',#36710,64.5);
#3502=CIRCLE('',#36712,64.5);
#3503=CIRCLE('',#36714,64.5);
#3504=CIRCLE('',#36716,64.5);
#3505=CIRCLE('',#36718,64.5);
#3506=CIRCLE('',#36720,64.5);
#3507=CIRCLE('',#36722,64.5);
#3508=CIRCLE('',#36724,64.5);
#3509=CIRCLE('',#36726,64.5);
#3510=CIRCLE('',#36728,64.5);
#3511=CIRCLE('',#36730,64.5);
#3512=CIRCLE('',#36732,64.5);
#3513=CIRCLE('',#36734,64.5);
#3514=CIRCLE('',#36736,59.00430282);
#3515=CIRCLE('',#36738,28.3018268963564);
#3516=CIRCLE('',#36740,28.3018268963564);
#3517=CIRCLE('',#36742,64.5);
#5272=FACE_OUTER_BOUND('',#7403,.T.);
#5273=FACE_OUTER_BOUND('',#7404,.T.);
#5274=FACE_OUTER_BOUND('',#7405,.T.);
#5275=FACE_OUTER_BOUND('',#7407,.T.);
#5276=FACE_OUTER_BOUND('',#7408,.T.);
#5277=FACE_OUTER_BOUND('',#7410,.T.);
#5278=FACE_OUTER_BOUND('',#7411,.T.);
#5279=FACE_OUTER_BOUND('',#7412,.T.);
#5280=FACE_OUTER_BOUND('',#7413,.T.);
#5281=FACE_OUTER_BOUND('',#7414,.T.);
#5282=FACE_OUTER_BOUND('',#7415,.T.);
#5283=FACE_OUTER_BOUND('',#7416,.T.);
#5284=FACE_OUTER_BOUND('',#7417,.T.);
#5285=FACE_OUTER_BOUND('',#7418,.T.);
#5286=FACE_OUTER_BOUND('',#7419,.T.);
#5287=FACE_OUTER_BOUND('',#7420,.T.);
#5288=FACE_OUTER_BOUND('',#7421,.T.);
#5289=FACE_OUTER_BOUND('',#7422,.T.);
#5290=FACE_OUTER_BOUND('',#7423,.T.);
#5291=FACE_OUTER_BOUND('',#7424,.T.);
#5292=FACE_OUTER_BOUND('',#7425,.T.);
#5293=FACE_OUTER_BOUND('',#7426,.T.);
#5294=FACE_OUTER_BOUND('',#7427,.T.);
#5295=FACE_OUTER_BOUND('',#7428,.T.);
#5296=FACE_OUTER_BOUND('',#7429,.T.);
#5297=FACE_OUTER_BOUND('',#7430,.T.);
#5298=FACE_OUTER_BOUND('',#7431,.T.);
#5299=FACE_OUTER_BOUND('',#7432,.T.);
#5300=FACE_OUTER_BOUND('',#7433,.T.);
#5301=FACE_OUTER_BOUND('',#7434,.T.);
#5302=FACE_OUTER_BOUND('',#7435,.T.);
#5303=FACE_OUTER_BOUND('',#7436,.T.);
#5304=FACE_OUTER_BOUND('',#7437,.T.);
#5305=FACE_OUTER_BOUND('',#7438,.T.);
#5306=FACE_OUTER_BOUND('',#7439,.T.);
#5307=FACE_OUTER_BOUND('',#7440,.T.);
#5308=FACE_OUTER_BOUND('',#7441,.T.);
#5309=FACE_OUTER_BOUND('',#7442,.T.);
#5310=FACE_OUTER_BOUND('',#7443,.T.);
#5311=FACE_OUTER_BOUND('',#7444,.T.);
#5312=FACE_OUTER_BOUND('',#7445,.T.);
#5313=FACE_OUTER_BOUND('',#7446,.T.);
#5314=FACE_OUTER_BOUND('',#7447,.T.);
#5315=FACE_OUTER_BOUND('',#7448,.T.);
#5316=FACE_OUTER_BOUND('',#7449,.T.);
#5317=FACE_OUTER_BOUND('',#7450,.T.);
#5318=FACE_OUTER_BOUND('',#7451,.T.);
#5319=FACE_OUTER_BOUND('',#7452,.T.);
#5320=FACE_OUTER_BOUND('',#7453,.T.);
#5321=FACE_OUTER_BOUND('',#7454,.T.);
#5322=FACE_OUTER_BOUND('',#7455,.T.);
#5323=FACE_OUTER_BOUND('',#7456,.T.);
#5324=FACE_OUTER_BOUND('',#7457,.T.);
#5325=FACE_OUTER_BOUND('',#7458,.T.);
#5326=FACE_OUTER_BOUND('',#7459,.T.);
#5327=FACE_OUTER_BOUND('',#7460,.T.);
#5328=FACE_OUTER_BOUND('',#7461,.T.);
#5329=FACE_OUTER_BOUND('',#7462,.T.);
#5330=FACE_OUTER_BOUND('',#7463,.T.);
#5331=FACE_OUTER_BOUND('',#7464,.T.);
#5332=FACE_OUTER_BOUND('',#7465,.T.);
#5333=FACE_OUTER_BOUND('',#7466,.T.);
#5334=FACE_OUTER_BOUND('',#7467,.T.);
#5335=FACE_OUTER_BOUND('',#7468,.T.);
#5336=FACE_OUTER_BOUND('',#7469,.T.);
#5337=FACE_OUTER_BOUND('',#7470,.T.);
#5338=FACE_OUTER_BOUND('',#7471,.T.);
#5339=FACE_OUTER_BOUND('',#7472,.T.);
#5340=FACE_OUTER_BOUND('',#7473,.T.);
#5341=FACE_OUTER_BOUND('',#7474,.T.);
#5342=FACE_OUTER_BOUND('',#7475,.T.);
#5343=FACE_OUTER_BOUND('',#7476,.T.);
#5344=FACE_OUTER_BOUND('',#7477,.T.);
#5345=FACE_OUTER_BOUND('',#7478,.T.);
#5346=FACE_OUTER_BOUND('',#7479,.T.);
#5347=FACE_OUTER_BOUND('',#7480,.T.);
#5348=FACE_OUTER_BOUND('',#7481,.T.);
#5349=FACE_OUTER_BOUND('',#7482,.T.);
#5350=FACE_OUTER_BOUND('',#7483,.T.);
#5351=FACE_OUTER_BOUND('',#7484,.T.);
#5352=FACE_OUTER_BOUND('',#7485,.T.);
#5353=FACE_OUTER_BOUND('',#7486,.T.);
#5354=FACE_OUTER_BOUND('',#7487,.T.);
#5355=FACE_OUTER_BOUND('',#7488,.T.);
#5356=FACE_OUTER_BOUND('',#7489,.T.);
#5357=FACE_OUTER_BOUND('',#7490,.T.);
#5358=FACE_OUTER_BOUND('',#7491,.T.);
#5359=FACE_OUTER_BOUND('',#7492,.T.);
#5360=FACE_OUTER_BOUND('',#7493,.T.);
#5361=FACE_OUTER_BOUND('',#7494,.T.);
#5362=FACE_OUTER_BOUND('',#7495,.T.);
#5363=FACE_OUTER_BOUND('',#7496,.T.);
#5364=FACE_OUTER_BOUND('',#7497,.T.);
#5365=FACE_OUTER_BOUND('',#7498,.T.);
#5366=FACE_OUTER_BOUND('',#7499,.T.);
#5367=FACE_OUTER_BOUND('',#7500,.T.);
#5368=FACE_OUTER_BOUND('',#7501,.T.);
#5369=FACE_OUTER_BOUND('',#7502,.T.);
#5370=FACE_OUTER_BOUND('',#7503,.T.);
#5371=FACE_OUTER_BOUND('',#7504,.T.);
#5372=FACE_OUTER_BOUND('',#7505,.T.);
#5373=FACE_OUTER_BOUND('',#7506,.T.);
#5374=FACE_OUTER_BOUND('',#7507,.T.);
#5375=FACE_OUTER_BOUND('',#7508,.T.);
#5376=FACE_OUTER_BOUND('',#7509,.T.);
#5377=FACE_OUTER_BOUND('',#7510,.T.);
#5378=FACE_OUTER_BOUND('',#7511,.T.);
#5379=FACE_OUTER_BOUND('',#7512,.T.);
#5380=FACE_OUTER_BOUND('',#7513,.T.);
#5381=FACE_OUTER_BOUND('',#7514,.T.);
#5382=FACE_OUTER_BOUND('',#7515,.T.);
#5383=FACE_OUTER_BOUND('',#7516,.T.);
#5384=FACE_OUTER_BOUND('',#7517,.T.);
#5385=FACE_OUTER_BOUND('',#7518,.T.);
#5386=FACE_OUTER_BOUND('',#7519,.T.);
#5387=FACE_OUTER_BOUND('',#7520,.T.);
#5388=FACE_OUTER_BOUND('',#7521,.T.);
#5389=FACE_OUTER_BOUND('',#7522,.T.);
#5390=FACE_OUTER_BOUND('',#7523,.T.);
#5391=FACE_OUTER_BOUND('',#7524,.T.);
#5392=FACE_OUTER_BOUND('',#7525,.T.);
#5393=FACE_OUTER_BOUND('',#7526,.T.);
#5394=FACE_OUTER_BOUND('',#7527,.T.);
#5395=FACE_OUTER_BOUND('',#7528,.T.);
#5396=FACE_OUTER_BOUND('',#7529,.T.);
#5397=FACE_OUTER_BOUND('',#7530,.T.);
#5398=FACE_OUTER_BOUND('',#7531,.T.);
#5399=FACE_OUTER_BOUND('',#7532,.T.);
#5400=FACE_OUTER_BOUND('',#7533,.T.);
#5401=FACE_OUTER_BOUND('',#7534,.T.);
#5402=FACE_OUTER_BOUND('',#7535,.T.);
#5403=FACE_OUTER_BOUND('',#7536,.T.);
#5404=FACE_OUTER_BOUND('',#7537,.T.);
#5405=FACE_OUTER_BOUND('',#7538,.T.);
#5406=FACE_OUTER_BOUND('',#7539,.T.);
#5407=FACE_OUTER_BOUND('',#7540,.T.);
#5408=FACE_OUTER_BOUND('',#7541,.T.);
#5409=FACE_OUTER_BOUND('',#7542,.T.);
#5410=FACE_OUTER_BOUND('',#7543,.T.);
#5411=FACE_OUTER_BOUND('',#7544,.T.);
#5412=FACE_OUTER_BOUND('',#7545,.T.);
#5413=FACE_OUTER_BOUND('',#7546,.T.);
#5414=FACE_OUTER_BOUND('',#7547,.T.);
#5415=FACE_OUTER_BOUND('',#7548,.T.);
#5416=FACE_OUTER_BOUND('',#7549,.T.);
#5417=FACE_OUTER_BOUND('',#7550,.T.);
#5418=FACE_OUTER_BOUND('',#7551,.T.);
#5419=FACE_OUTER_BOUND('',#7552,.T.);
#5420=FACE_OUTER_BOUND('',#7553,.T.);
#5421=FACE_OUTER_BOUND('',#7554,.T.);
#5422=FACE_OUTER_BOUND('',#7555,.T.);
#5423=FACE_OUTER_BOUND('',#7556,.T.);
#5424=FACE_OUTER_BOUND('',#7557,.T.);
#5425=FACE_OUTER_BOUND('',#7558,.T.);
#5426=FACE_OUTER_BOUND('',#7559,.T.);
#5427=FACE_OUTER_BOUND('',#7560,.T.);
#5428=FACE_OUTER_BOUND('',#7561,.T.);
#5429=FACE_OUTER_BOUND('',#7562,.T.);
#5430=FACE_OUTER_BOUND('',#7563,.T.);
#5431=FACE_OUTER_BOUND('',#7564,.T.);
#5432=FACE_OUTER_BOUND('',#7565,.T.);
#5433=FACE_OUTER_BOUND('',#7566,.T.);
#5434=FACE_OUTER_BOUND('',#7567,.T.);
#5435=FACE_OUTER_BOUND('',#7568,.T.);
#5436=FACE_OUTER_BOUND('',#7569,.T.);
#5437=FACE_OUTER_BOUND('',#7570,.T.);
#5438=FACE_OUTER_BOUND('',#7571,.T.);
#5439=FACE_OUTER_BOUND('',#7572,.T.);
#5440=FACE_OUTER_BOUND('',#7573,.T.);
#5441=FACE_OUTER_BOUND('',#7574,.T.);
#5442=FACE_OUTER_BOUND('',#7575,.T.);
#5443=FACE_OUTER_BOUND('',#7576,.T.);
#5444=FACE_OUTER_BOUND('',#7577,.T.);
#5445=FACE_OUTER_BOUND('',#7578,.T.);
#5446=FACE_OUTER_BOUND('',#7579,.T.);
#5447=FACE_OUTER_BOUND('',#7580,.T.);
#5448=FACE_OUTER_BOUND('',#7581,.T.);
#5449=FACE_OUTER_BOUND('',#7582,.T.);
#5450=FACE_OUTER_BOUND('',#7583,.T.);
#5451=FACE_OUTER_BOUND('',#7584,.T.);
#5452=FACE_OUTER_BOUND('',#7585,.T.);
#5453=FACE_OUTER_BOUND('',#7586,.T.);
#5454=FACE_OUTER_BOUND('',#7587,.T.);
#5455=FACE_OUTER_BOUND('',#7588,.T.);
#5456=FACE_OUTER_BOUND('',#7589,.T.);
#5457=FACE_OUTER_BOUND('',#7590,.T.);
#5458=FACE_OUTER_BOUND('',#7591,.T.);
#5459=FACE_OUTER_BOUND('',#7592,.T.);
#5460=FACE_OUTER_BOUND('',#7593,.T.);
#5461=FACE_OUTER_BOUND('',#7594,.T.);
#5462=FACE_OUTER_BOUND('',#7595,.T.);
#5463=FACE_OUTER_BOUND('',#7596,.T.);
#5464=FACE_OUTER_BOUND('',#7597,.T.);
#5465=FACE_OUTER_BOUND('',#7598,.T.);
#5466=FACE_OUTER_BOUND('',#7599,.T.);
#5467=FACE_OUTER_BOUND('',#7600,.T.);
#5468=FACE_OUTER_BOUND('',#7601,.T.);
#5469=FACE_OUTER_BOUND('',#7602,.T.);
#5470=FACE_OUTER_BOUND('',#7603,.T.);
#5471=FACE_OUTER_BOUND('',#7604,.T.);
#5472=FACE_OUTER_BOUND('',#7605,.T.);
#5473=FACE_OUTER_BOUND('',#7606,.T.);
#7403=EDGE_LOOP('',(#26578,#26579,#26580,#26581,#26582));
#7404=EDGE_LOOP('',(#26583,#26584,#26585,#26586,#26587));
#7405=EDGE_LOOP('',(#26588));
#7406=EDGE_LOOP('',(#26589,#26590,#26591,#26592));
#7407=EDGE_LOOP('',(#26593,#26594,#26595,#26596));
#7408=EDGE_LOOP('',(#26597,#26598,#26599,#26600,#26601,#26602,#26603,#26604,
#26605,#26606,#26607,#26608,#26609,#26610,#26611,#26612,#26613,#26614,#26615,
#26616,#26617,#26618,#26619,#26620,#26621,#26622,#26623,#26624,#26625,#26626,
#26627,#26628,#26629,#26630,#26631,#26632,#26633,#26634,#26635,#26636,#26637,
#26638,#26639,#26640,#26641,#26642,#26643,#26644,#26645,#26646,#26647,#26648,
#26649,#26650,#26651,#26652,#26653,#26654,#26655,#26656,#26657,#26658,#26659,
#26660,#26661,#26662,#26663,#26664,#26665,#26666,#26667,#26668,#26669,#26670,
#26671,#26672,#26673,#26674,#26675,#26676,#26677,#26678,#26679,#26680,#26681,
#26682,#26683,#26684,#26685,#26686,#26687,#26688,#26689,#26690,#26691,#26692,
#26693,#26694,#26695,#26696,#26697,#26698,#26699,#26700,#26701,#26702,#26703,
#26704,#26705,#26706,#26707,#26708,#26709,#26710,#26711,#26712,#26713,#26714,
#26715,#26716,#26717,#26718,#26719,#26720,#26721,#26722,#26723,#26724,#26725,
#26726,#26727,#26728,#26729,#26730,#26731,#26732,#26733,#26734,#26735,#26736,
#26737,#26738,#26739,#26740,#26741,#26742,#26743,#26744,#26745,#26746,#26747,
#26748,#26749,#26750,#26751,#26752,#26753,#26754,#26755,#26756,#26757,#26758,
#26759,#26760,#26761,#26762,#26763,#26764,#26765,#26766,#26767,#26768,#26769,
#26770,#26771,#26772,#26773,#26774,#26775,#26776,#26777,#26778,#26779,#26780,
#26781,#26782,#26783,#26784,#26785,#26786,#26787,#26788));
#7409=EDGE_LOOP('',(#26789));
#7410=EDGE_LOOP('',(#26790,#26791,#26792,#26793));
#7411=EDGE_LOOP('',(#26794,#26795,#26796,#26797));
#7412=EDGE_LOOP('',(#26798,#26799,#26800,#26801));
#7413=EDGE_LOOP('',(#26802,#26803,#26804,#26805));
#7414=EDGE_LOOP('',(#26806,#26807,#26808,#26809));
#7415=EDGE_LOOP('',(#26810,#26811,#26812,#26813));
#7416=EDGE_LOOP('',(#26814,#26815,#26816,#26817));
#7417=EDGE_LOOP('',(#26818,#26819,#26820,#26821));
#7418=EDGE_LOOP('',(#26822,#26823,#26824,#26825));
#7419=EDGE_LOOP('',(#26826,#26827,#26828,#26829));
#7420=EDGE_LOOP('',(#26830,#26831,#26832,#26833));
#7421=EDGE_LOOP('',(#26834,#26835,#26836,#26837));
#7422=EDGE_LOOP('',(#26838,#26839,#26840,#26841));
#7423=EDGE_LOOP('',(#26842,#26843,#26844,#26845));
#7424=EDGE_LOOP('',(#26846,#26847,#26848,#26849));
#7425=EDGE_LOOP('',(#26850,#26851,#26852,#26853));
#7426=EDGE_LOOP('',(#26854,#26855,#26856,#26857));
#7427=EDGE_LOOP('',(#26858,#26859,#26860,#26861));
#7428=EDGE_LOOP('',(#26862,#26863,#26864,#26865));
#7429=EDGE_LOOP('',(#26866,#26867,#26868,#26869));
#7430=EDGE_LOOP('',(#26870,#26871,#26872,#26873));
#7431=EDGE_LOOP('',(#26874,#26875,#26876,#26877));
#7432=EDGE_LOOP('',(#26878,#26879,#26880,#26881));
#7433=EDGE_LOOP('',(#26882,#26883,#26884,#26885));
#7434=EDGE_LOOP('',(#26886,#26887,#26888,#26889));
#7435=EDGE_LOOP('',(#26890,#26891,#26892,#26893));
#7436=EDGE_LOOP('',(#26894,#26895,#26896,#26897));
#7437=EDGE_LOOP('',(#26898,#26899,#26900,#26901));
#7438=EDGE_LOOP('',(#26902,#26903,#26904,#26905));
#7439=EDGE_LOOP('',(#26906,#26907,#26908,#26909));
#7440=EDGE_LOOP('',(#26910,#26911,#26912,#26913));
#7441=EDGE_LOOP('',(#26914,#26915,#26916,#26917));
#7442=EDGE_LOOP('',(#26918,#26919,#26920,#26921));
#7443=EDGE_LOOP('',(#26922,#26923,#26924,#26925));
#7444=EDGE_LOOP('',(#26926,#26927,#26928,#26929));
#7445=EDGE_LOOP('',(#26930,#26931,#26932,#26933));
#7446=EDGE_LOOP('',(#26934,#26935,#26936,#26937));
#7447=EDGE_LOOP('',(#26938,#26939,#26940,#26941));
#7448=EDGE_LOOP('',(#26942,#26943,#26944,#26945));
#7449=EDGE_LOOP('',(#26946,#26947,#26948,#26949));
#7450=EDGE_LOOP('',(#26950,#26951,#26952,#26953));
#7451=EDGE_LOOP('',(#26954,#26955,#26956,#26957));
#7452=EDGE_LOOP('',(#26958,#26959,#26960,#26961));
#7453=EDGE_LOOP('',(#26962,#26963,#26964,#26965));
#7454=EDGE_LOOP('',(#26966,#26967,#26968,#26969));
#7455=EDGE_LOOP('',(#26970,#26971,#26972,#26973));
#7456=EDGE_LOOP('',(#26974,#26975,#26976,#26977));
#7457=EDGE_LOOP('',(#26978,#26979,#26980,#26981));
#7458=EDGE_LOOP('',(#26982,#26983,#26984,#26985));
#7459=EDGE_LOOP('',(#26986,#26987,#26988,#26989));
#7460=EDGE_LOOP('',(#26990,#26991,#26992,#26993));
#7461=EDGE_LOOP('',(#26994,#26995,#26996,#26997));
#7462=EDGE_LOOP('',(#26998,#26999,#27000,#27001));
#7463=EDGE_LOOP('',(#27002,#27003,#27004,#27005));
#7464=EDGE_LOOP('',(#27006,#27007,#27008,#27009));
#7465=EDGE_LOOP('',(#27010,#27011,#27012,#27013));
#7466=EDGE_LOOP('',(#27014,#27015,#27016,#27017));
#7467=EDGE_LOOP('',(#27018,#27019,#27020,#27021));
#7468=EDGE_LOOP('',(#27022,#27023,#27024,#27025));
#7469=EDGE_LOOP('',(#27026,#27027,#27028,#27029));
#7470=EDGE_LOOP('',(#27030,#27031,#27032,#27033));
#7471=EDGE_LOOP('',(#27034,#27035,#27036,#27037));
#7472=EDGE_LOOP('',(#27038,#27039,#27040,#27041));
#7473=EDGE_LOOP('',(#27042,#27043,#27044,#27045));
#7474=EDGE_LOOP('',(#27046,#27047,#27048,#27049));
#7475=EDGE_LOOP('',(#27050,#27051,#27052,#27053));
#7476=EDGE_LOOP('',(#27054,#27055,#27056,#27057));
#7477=EDGE_LOOP('',(#27058,#27059,#27060,#27061));
#7478=EDGE_LOOP('',(#27062,#27063,#27064,#27065));
#7479=EDGE_LOOP('',(#27066,#27067,#27068,#27069));
#7480=EDGE_LOOP('',(#27070,#27071,#27072,#27073));
#7481=EDGE_LOOP('',(#27074,#27075,#27076,#27077));
#7482=EDGE_LOOP('',(#27078,#27079,#27080,#27081));
#7483=EDGE_LOOP('',(#27082,#27083,#27084,#27085));
#7484=EDGE_LOOP('',(#27086,#27087,#27088,#27089));
#7485=EDGE_LOOP('',(#27090,#27091,#27092,#27093));
#7486=EDGE_LOOP('',(#27094,#27095,#27096,#27097));
#7487=EDGE_LOOP('',(#27098,#27099,#27100,#27101));
#7488=EDGE_LOOP('',(#27102,#27103,#27104,#27105));
#7489=EDGE_LOOP('',(#27106,#27107,#27108,#27109));
#7490=EDGE_LOOP('',(#27110,#27111,#27112,#27113));
#7491=EDGE_LOOP('',(#27114,#27115,#27116,#27117));
#7492=EDGE_LOOP('',(#27118,#27119,#27120,#27121));
#7493=EDGE_LOOP('',(#27122,#27123,#27124,#27125));
#7494=EDGE_LOOP('',(#27126,#27127,#27128,#27129));
#7495=EDGE_LOOP('',(#27130,#27131,#27132,#27133));
#7496=EDGE_LOOP('',(#27134,#27135,#27136,#27137));
#7497=EDGE_LOOP('',(#27138,#27139,#27140,#27141));
#7498=EDGE_LOOP('',(#27142,#27143,#27144,#27145));
#7499=EDGE_LOOP('',(#27146,#27147,#27148,#27149));
#7500=EDGE_LOOP('',(#27150,#27151,#27152,#27153));
#7501=EDGE_LOOP('',(#27154,#27155,#27156,#27157));
#7502=EDGE_LOOP('',(#27158,#27159,#27160,#27161));
#7503=EDGE_LOOP('',(#27162,#27163,#27164,#27165));
#7504=EDGE_LOOP('',(#27166,#27167,#27168,#27169));
#7505=EDGE_LOOP('',(#27170,#27171,#27172,#27173));
#7506=EDGE_LOOP('',(#27174,#27175,#27176,#27177));
#7507=EDGE_LOOP('',(#27178,#27179,#27180,#27181));
#7508=EDGE_LOOP('',(#27182,#27183,#27184,#27185));
#7509=EDGE_LOOP('',(#27186,#27187,#27188,#27189));
#7510=EDGE_LOOP('',(#27190,#27191,#27192,#27193));
#7511=EDGE_LOOP('',(#27194,#27195,#27196,#27197));
#7512=EDGE_LOOP('',(#27198,#27199,#27200,#27201));
#7513=EDGE_LOOP('',(#27202,#27203,#27204,#27205));
#7514=EDGE_LOOP('',(#27206,#27207,#27208,#27209));
#7515=EDGE_LOOP('',(#27210,#27211,#27212,#27213));
#7516=EDGE_LOOP('',(#27214,#27215,#27216,#27217));
#7517=EDGE_LOOP('',(#27218,#27219,#27220,#27221));
#7518=EDGE_LOOP('',(#27222,#27223,#27224,#27225));
#7519=EDGE_LOOP('',(#27226,#27227,#27228,#27229));
#7520=EDGE_LOOP('',(#27230,#27231,#27232,#27233));
#7521=EDGE_LOOP('',(#27234,#27235,#27236,#27237));
#7522=EDGE_LOOP('',(#27238,#27239,#27240,#27241));
#7523=EDGE_LOOP('',(#27242,#27243,#27244,#27245));
#7524=EDGE_LOOP('',(#27246,#27247,#27248,#27249));
#7525=EDGE_LOOP('',(#27250,#27251,#27252,#27253));
#7526=EDGE_LOOP('',(#27254,#27255,#27256,#27257));
#7527=EDGE_LOOP('',(#27258,#27259,#27260,#27261));
#7528=EDGE_LOOP('',(#27262,#27263,#27264,#27265));
#7529=EDGE_LOOP('',(#27266,#27267,#27268,#27269));
#7530=EDGE_LOOP('',(#27270,#27271,#27272,#27273));
#7531=EDGE_LOOP('',(#27274,#27275,#27276,#27277));
#7532=EDGE_LOOP('',(#27278,#27279,#27280,#27281));
#7533=EDGE_LOOP('',(#27282,#27283,#27284,#27285));
#7534=EDGE_LOOP('',(#27286,#27287,#27288,#27289));
#7535=EDGE_LOOP('',(#27290,#27291,#27292,#27293));
#7536=EDGE_LOOP('',(#27294,#27295,#27296,#27297));
#7537=EDGE_LOOP('',(#27298,#27299,#27300,#27301));
#7538=EDGE_LOOP('',(#27302,#27303,#27304,#27305));
#7539=EDGE_LOOP('',(#27306,#27307,#27308,#27309));
#7540=EDGE_LOOP('',(#27310,#27311,#27312,#27313));
#7541=EDGE_LOOP('',(#27314,#27315,#27316,#27317));
#7542=EDGE_LOOP('',(#27318,#27319,#27320,#27321));
#7543=EDGE_LOOP('',(#27322,#27323,#27324,#27325));
#7544=EDGE_LOOP('',(#27326,#27327,#27328,#27329));
#7545=EDGE_LOOP('',(#27330,#27331,#27332,#27333));
#7546=EDGE_LOOP('',(#27334,#27335,#27336,#27337));
#7547=EDGE_LOOP('',(#27338,#27339,#27340,#27341));
#7548=EDGE_LOOP('',(#27342,#27343,#27344,#27345));
#7549=EDGE_LOOP('',(#27346,#27347,#27348,#27349));
#7550=EDGE_LOOP('',(#27350,#27351,#27352,#27353));
#7551=EDGE_LOOP('',(#27354,#27355,#27356,#27357));
#7552=EDGE_LOOP('',(#27358,#27359,#27360,#27361));
#7553=EDGE_LOOP('',(#27362,#27363,#27364,#27365));
#7554=EDGE_LOOP('',(#27366,#27367,#27368,#27369));
#7555=EDGE_LOOP('',(#27370,#27371,#27372,#27373));
#7556=EDGE_LOOP('',(#27374,#27375,#27376,#27377));
#7557=EDGE_LOOP('',(#27378,#27379,#27380,#27381));
#7558=EDGE_LOOP('',(#27382,#27383,#27384,#27385));
#7559=EDGE_LOOP('',(#27386,#27387,#27388,#27389));
#7560=EDGE_LOOP('',(#27390,#27391,#27392,#27393));
#7561=EDGE_LOOP('',(#27394,#27395,#27396,#27397));
#7562=EDGE_LOOP('',(#27398,#27399,#27400,#27401));
#7563=EDGE_LOOP('',(#27402,#27403,#27404,#27405));
#7564=EDGE_LOOP('',(#27406,#27407,#27408,#27409));
#7565=EDGE_LOOP('',(#27410,#27411,#27412,#27413));
#7566=EDGE_LOOP('',(#27414,#27415,#27416,#27417));
#7567=EDGE_LOOP('',(#27418,#27419,#27420,#27421));
#7568=EDGE_LOOP('',(#27422,#27423,#27424,#27425));
#7569=EDGE_LOOP('',(#27426,#27427,#27428,#27429));
#7570=EDGE_LOOP('',(#27430,#27431,#27432,#27433));
#7571=EDGE_LOOP('',(#27434,#27435,#27436,#27437));
#7572=EDGE_LOOP('',(#27438,#27439,#27440,#27441));
#7573=EDGE_LOOP('',(#27442,#27443,#27444,#27445));
#7574=EDGE_LOOP('',(#27446,#27447,#27448,#27449));
#7575=EDGE_LOOP('',(#27450,#27451,#27452,#27453));
#7576=EDGE_LOOP('',(#27454,#27455,#27456,#27457));
#7577=EDGE_LOOP('',(#27458,#27459,#27460,#27461));
#7578=EDGE_LOOP('',(#27462,#27463,#27464,#27465));
#7579=EDGE_LOOP('',(#27466,#27467,#27468,#27469));
#7580=EDGE_LOOP('',(#27470,#27471,#27472,#27473));
#7581=EDGE_LOOP('',(#27474,#27475,#27476,#27477));
#7582=EDGE_LOOP('',(#27478,#27479,#27480,#27481));
#7583=EDGE_LOOP('',(#27482,#27483,#27484,#27485));
#7584=EDGE_LOOP('',(#27486,#27487,#27488,#27489));
#7585=EDGE_LOOP('',(#27490,#27491,#27492,#27493));
#7586=EDGE_LOOP('',(#27494,#27495,#27496,#27497));
#7587=EDGE_LOOP('',(#27498,#27499,#27500,#27501));
#7588=EDGE_LOOP('',(#27502,#27503,#27504,#27505));
#7589=EDGE_LOOP('',(#27506,#27507,#27508,#27509));
#7590=EDGE_LOOP('',(#27510,#27511,#27512,#27513));
#7591=EDGE_LOOP('',(#27514,#27515,#27516,#27517));
#7592=EDGE_LOOP('',(#27518,#27519,#27520,#27521));
#7593=EDGE_LOOP('',(#27522,#27523,#27524,#27525));
#7594=EDGE_LOOP('',(#27526,#27527,#27528,#27529));
#7595=EDGE_LOOP('',(#27530,#27531,#27532,#27533));
#7596=EDGE_LOOP('',(#27534,#27535,#27536,#27537));
#7597=EDGE_LOOP('',(#27538,#27539,#27540,#27541));
#7598=EDGE_LOOP('',(#27542,#27543,#27544,#27545));
#7599=EDGE_LOOP('',(#27546,#27547,#27548,#27549));
#7600=EDGE_LOOP('',(#27550,#27551,#27552,#27553));
#7601=EDGE_LOOP('',(#27554,#27555,#27556,#27557));
#7602=EDGE_LOOP('',(#27558,#27559,#27560,#27561));
#7603=EDGE_LOOP('',(#27562,#27563,#27564,#27565));
#7604=EDGE_LOOP('',(#27566,#27567,#27568,#27569));
#7605=EDGE_LOOP('',(#27570,#27571,#27572,#27573));
#7606=EDGE_LOOP('',(#27574,#27575,#27576,#27577,#27578,#27579,#27580,#27581,
#27582,#27583,#27584,#27585,#27586,#27587,#27588,#27589,#27590,#27591,#27592,
#27593,#27594,#27595,#27596,#27597,#27598,#27599,#27600,#27601,#27602,#27603,
#27604,#27605,#27606,#27607,#27608,#27609,#27610,#27611,#27612,#27613,#27614,
#27615,#27616,#27617,#27618,#27619,#27620,#27621,#27622,#27623,#27624,#27625,
#27626,#27627,#27628,#27629,#27630,#27631,#27632,#27633,#27634,#27635,#27636,
#27637,#27638,#27639,#27640,#27641,#27642,#27643,#27644,#27645,#27646,#27647,
#27648,#27649,#27650,#27651,#27652,#27653,#27654,#27655,#27656,#27657,#27658,
#27659,#27660,#27661,#27662,#27663,#27664,#27665,#27666,#27667,#27668,#27669,
#27670,#27671,#27672,#27673,#27674,#27675,#27676,#27677,#27678,#27679,#27680,
#27681,#27682,#27683,#27684,#27685,#27686,#27687,#27688,#27689,#27690,#27691,
#27692,#27693,#27694,#27695,#27696,#27697,#27698,#27699,#27700,#27701,#27702,
#27703,#27704,#27705,#27706,#27707,#27708,#27709,#27710,#27711,#27712,#27713,
#27714,#27715,#27716,#27717,#27718,#27719,#27720,#27721,#27722,#27723,#27724,
#27725,#27726,#27727,#27728,#27729,#27730,#27731,#27732,#27733,#27734,#27735,
#27736,#27737,#27738,#27739,#27740,#27741,#27742,#27743,#27744,#27745,#27746,
#27747,#27748,#27749,#27750,#27751,#27752,#27753,#27754,#27755,#27756,#27757,
#27758,#27759,#27760,#27761,#27762,#27763,#27764,#27765));
#7607=EDGE_LOOP('',(#27766,#27767,#27768,#27769));
#9826=LINE('',#56415,#12373);
#9827=LINE('',#56420,#12374);
#9828=LINE('',#56422,#12375);
#9829=LINE('',#56424,#12376);
#9830=LINE('',#56818,#12377);
#9831=LINE('',#56819,#12378);
#9832=LINE('',#56820,#12379);
#9833=LINE('',#56823,#12380);
#9834=LINE('',#56824,#12381);
#9835=LINE('',#56828,#12382);
#9836=LINE('',#56830,#12383);
#9837=LINE('',#56833,#12384);
#9838=LINE('',#56836,#12385);
#9839=LINE('',#56840,#12386);
#9840=LINE('',#56843,#12387);
#9841=LINE('',#56847,#12388);
#9842=LINE('',#56850,#12389);
#9843=LINE('',#56854,#12390);
#9844=LINE('',#56857,#12391);
#9845=LINE('',#56861,#12392);
#9846=LINE('',#56864,#12393);
#9847=LINE('',#56868,#12394);
#9848=LINE('',#56871,#12395);
#9849=LINE('',#56875,#12396);
#9850=LINE('',#56878,#12397);
#9851=LINE('',#56882,#12398);
#9852=LINE('',#56885,#12399);
#9853=LINE('',#56889,#12400);
#9854=LINE('',#56892,#12401);
#9855=LINE('',#56896,#12402);
#9856=LINE('',#56899,#12403);
#9857=LINE('',#56903,#12404);
#9858=LINE('',#56906,#12405);
#9859=LINE('',#56910,#12406);
#9860=LINE('',#56913,#12407);
#9861=LINE('',#56917,#12408);
#9862=LINE('',#56920,#12409);
#9863=LINE('',#56924,#12410);
#9864=LINE('',#56927,#12411);
#9865=LINE('',#56931,#12412);
#9866=LINE('',#56934,#12413);
#9867=LINE('',#56938,#12414);
#9868=LINE('',#56941,#12415);
#9869=LINE('',#56945,#12416);
#9870=LINE('',#56948,#12417);
#9871=LINE('',#56952,#12418);
#9872=LINE('',#56955,#12419);
#9873=LINE('',#56959,#12420);
#9874=LINE('',#56962,#12421);
#9875=LINE('',#56966,#12422);
#9876=LINE('',#56969,#12423);
#9877=LINE('',#56973,#12424);
#9878=LINE('',#56976,#12425);
#9879=LINE('',#56980,#12426);
#9880=LINE('',#56983,#12427);
#9881=LINE('',#56987,#12428);
#9882=LINE('',#56990,#12429);
#9883=LINE('',#56994,#12430);
#9884=LINE('',#56997,#12431);
#9885=LINE('',#57001,#12432);
#9886=LINE('',#57004,#12433);
#9887=LINE('',#57008,#12434);
#9888=LINE('',#57011,#12435);
#9889=LINE('',#57015,#12436);
#9890=LINE('',#57018,#12437);
#9891=LINE('',#57022,#12438);
#9892=LINE('',#57025,#12439);
#9893=LINE('',#57029,#12440);
#9894=LINE('',#57032,#12441);
#9895=LINE('',#57036,#12442);
#9896=LINE('',#57039,#12443);
#9897=LINE('',#57043,#12444);
#9898=LINE('',#57046,#12445);
#9899=LINE('',#57050,#12446);
#9900=LINE('',#57053,#12447);
#9901=LINE('',#57057,#12448);
#9902=LINE('',#57060,#12449);
#9903=LINE('',#57064,#12450);
#9904=LINE('',#57067,#12451);
#9905=LINE('',#57071,#12452);
#9906=LINE('',#57074,#12453);
#9907=LINE('',#57078,#12454);
#9908=LINE('',#57081,#12455);
#9909=LINE('',#57085,#12456);
#9910=LINE('',#57088,#12457);
#9911=LINE('',#57092,#12458);
#9912=LINE('',#57095,#12459);
#9913=LINE('',#57099,#12460);
#9914=LINE('',#57102,#12461);
#9915=LINE('',#57106,#12462);
#9916=LINE('',#57109,#12463);
#9917=LINE('',#57113,#12464);
#9918=LINE('',#57116,#12465);
#9919=LINE('',#57120,#12466);
#9920=LINE('',#57123,#12467);
#9921=LINE('',#57127,#12468);
#9922=LINE('',#57130,#12469);
#9923=LINE('',#57134,#12470);
#9924=LINE('',#57137,#12471);
#9925=LINE('',#57141,#12472);
#9926=LINE('',#57144,#12473);
#9927=LINE('',#57148,#12474);
#9928=LINE('',#57151,#12475);
#9929=LINE('',#57155,#12476);
#9930=LINE('',#57158,#12477);
#9931=LINE('',#57162,#12478);
#9932=LINE('',#57165,#12479);
#9933=LINE('',#57169,#12480);
#9934=LINE('',#57172,#12481);
#9935=LINE('',#57176,#12482);
#9936=LINE('',#57179,#12483);
#9937=LINE('',#57183,#12484);
#9938=LINE('',#57186,#12485);
#9939=LINE('',#57190,#12486);
#9940=LINE('',#57193,#12487);
#9941=LINE('',#57197,#12488);
#9942=LINE('',#57200,#12489);
#9943=LINE('',#57204,#12490);
#9944=LINE('',#57207,#12491);
#9945=LINE('',#57211,#12492);
#9946=LINE('',#57214,#12493);
#9947=LINE('',#57218,#12494);
#9948=LINE('',#57221,#12495);
#9949=LINE('',#57225,#12496);
#9950=LINE('',#57228,#12497);
#9951=LINE('',#57232,#12498);
#9952=LINE('',#57235,#12499);
#9953=LINE('',#57239,#12500);
#9954=LINE('',#57242,#12501);
#9955=LINE('',#57246,#12502);
#9956=LINE('',#57249,#12503);
#9957=LINE('',#57253,#12504);
#9958=LINE('',#57256,#12505);
#9959=LINE('',#57260,#12506);
#9960=LINE('',#57263,#12507);
#9961=LINE('',#57267,#12508);
#9962=LINE('',#57270,#12509);
#9963=LINE('',#57274,#12510);
#9964=LINE('',#57277,#12511);
#9965=LINE('',#57281,#12512);
#9966=LINE('',#57284,#12513);
#9967=LINE('',#57288,#12514);
#9968=LINE('',#57291,#12515);
#9969=LINE('',#57295,#12516);
#9970=LINE('',#57298,#12517);
#9971=LINE('',#57302,#12518);
#9972=LINE('',#57305,#12519);
#9973=LINE('',#57309,#12520);
#9974=LINE('',#57312,#12521);
#9975=LINE('',#57316,#12522);
#9976=LINE('',#57319,#12523);
#9977=LINE('',#57323,#12524);
#9978=LINE('',#57326,#12525);
#9979=LINE('',#57330,#12526);
#9980=LINE('',#57333,#12527);
#9981=LINE('',#57337,#12528);
#9982=LINE('',#57340,#12529);
#9983=LINE('',#57344,#12530);
#9984=LINE('',#57347,#12531);
#9985=LINE('',#57351,#12532);
#9986=LINE('',#57354,#12533);
#9987=LINE('',#57358,#12534);
#9988=LINE('',#57361,#12535);
#9989=LINE('',#57365,#12536);
#9990=LINE('',#57368,#12537);
#9991=LINE('',#57372,#12538);
#9992=LINE('',#57375,#12539);
#9993=LINE('',#57379,#12540);
#9994=LINE('',#57382,#12541);
#9995=LINE('',#57386,#12542);
#9996=LINE('',#57389,#12543);
#9997=LINE('',#57393,#12544);
#9998=LINE('',#57396,#12545);
#9999=LINE('',#57400,#12546);
#10000=LINE('',#57403,#12547);
#10001=LINE('',#57407,#12548);
#10002=LINE('',#57410,#12549);
#10003=LINE('',#57414,#12550);
#10004=LINE('',#57417,#12551);
#10005=LINE('',#57421,#12552);
#10006=LINE('',#57424,#12553);
#10007=LINE('',#57428,#12554);
#10008=LINE('',#57431,#12555);
#10009=LINE('',#57435,#12556);
#10010=LINE('',#57438,#12557);
#10011=LINE('',#57442,#12558);
#10012=LINE('',#57445,#12559);
#10013=LINE('',#57449,#12560);
#10014=LINE('',#57452,#12561);
#10015=LINE('',#57456,#12562);
#10016=LINE('',#57459,#12563);
#10017=LINE('',#57463,#12564);
#10018=LINE('',#57466,#12565);
#10019=LINE('',#57470,#12566);
#10020=LINE('',#57473,#12567);
#10021=LINE('',#57477,#12568);
#10022=LINE('',#57480,#12569);
#10023=LINE('',#57484,#12570);
#10024=LINE('',#57487,#12571);
#10025=LINE('',#57492,#12572);
#10026=LINE('',#57587,#12573);
#10027=LINE('',#57590,#12574);
#10028=LINE('',#57594,#12575);
#12373=VECTOR('',#43732,30.);
#12374=VECTOR('',#43737,10.);
#12375=VECTOR('',#43738,10.);
#12376=VECTOR('',#43739,10.);
#12377=VECTOR('',#44136,10.);
#12378=VECTOR('',#44137,10.);
#12379=VECTOR('',#44138,10.);
#12380=VECTOR('',#44141,10.);
#12381=VECTOR('',#44142,10.);
#12382=VECTOR('',#44147,10.);
#12383=VECTOR('',#44150,10.);
#12384=VECTOR('',#44153,10.);
#12385=VECTOR('',#44156,10.);
#12386=VECTOR('',#44161,10.);
#12387=VECTOR('',#44164,10.);
#12388=VECTOR('',#44169,10.);
#12389=VECTOR('',#44172,10.);
#12390=VECTOR('',#44177,10.);
#12391=VECTOR('',#44180,10.);
#12392=VECTOR('',#44185,10.);
#12393=VECTOR('',#44188,10.);
#12394=VECTOR('',#44193,10.);
#12395=VECTOR('',#44196,10.);
#12396=VECTOR('',#44201,10.);
#12397=VECTOR('',#44204,10.);
#12398=VECTOR('',#44209,10.);
#12399=VECTOR('',#44212,10.);
#12400=VECTOR('',#44217,10.);
#12401=VECTOR('',#44220,10.);
#12402=VECTOR('',#44225,10.);
#12403=VECTOR('',#44228,10.);
#12404=VECTOR('',#44233,10.);
#12405=VECTOR('',#44236,10.);
#12406=VECTOR('',#44241,10.);
#12407=VECTOR('',#44244,10.);
#12408=VECTOR('',#44249,10.);
#12409=VECTOR('',#44252,10.);
#12410=VECTOR('',#44257,10.);
#12411=VECTOR('',#44260,10.);
#12412=VECTOR('',#44265,10.);
#12413=VECTOR('',#44268,10.);
#12414=VECTOR('',#44273,10.);
#12415=VECTOR('',#44276,10.);
#12416=VECTOR('',#44281,10.);
#12417=VECTOR('',#44284,10.);
#12418=VECTOR('',#44289,10.);
#12419=VECTOR('',#44292,10.);
#12420=VECTOR('',#44297,10.);
#12421=VECTOR('',#44300,10.);
#12422=VECTOR('',#44305,10.);
#12423=VECTOR('',#44308,10.);
#12424=VECTOR('',#44313,10.);
#12425=VECTOR('',#44316,10.);
#12426=VECTOR('',#44321,10.);
#12427=VECTOR('',#44324,10.);
#12428=VECTOR('',#44329,10.);
#12429=VECTOR('',#44332,10.);
#12430=VECTOR('',#44337,10.);
#12431=VECTOR('',#44340,10.);
#12432=VECTOR('',#44345,10.);
#12433=VECTOR('',#44348,10.);
#12434=VECTOR('',#44353,10.);
#12435=VECTOR('',#44356,10.);
#12436=VECTOR('',#44361,10.);
#12437=VECTOR('',#44364,10.);
#12438=VECTOR('',#44369,10.);
#12439=VECTOR('',#44372,10.);
#12440=VECTOR('',#44377,10.);
#12441=VECTOR('',#44380,10.);
#12442=VECTOR('',#44385,10.);
#12443=VECTOR('',#44388,10.);
#12444=VECTOR('',#44393,10.);
#12445=VECTOR('',#44396,10.);
#12446=VECTOR('',#44401,10.);
#12447=VECTOR('',#44404,10.);
#12448=VECTOR('',#44409,10.);
#12449=VECTOR('',#44412,10.);
#12450=VECTOR('',#44417,10.);
#12451=VECTOR('',#44420,10.);
#12452=VECTOR('',#44425,10.);
#12453=VECTOR('',#44428,10.);
#12454=VECTOR('',#44433,10.);
#12455=VECTOR('',#44436,10.);
#12456=VECTOR('',#44441,10.);
#12457=VECTOR('',#44444,10.);
#12458=VECTOR('',#44449,10.);
#12459=VECTOR('',#44452,10.);
#12460=VECTOR('',#44457,10.);
#12461=VECTOR('',#44460,10.);
#12462=VECTOR('',#44465,10.);
#12463=VECTOR('',#44468,10.);
#12464=VECTOR('',#44473,10.);
#12465=VECTOR('',#44476,10.);
#12466=VECTOR('',#44481,10.);
#12467=VECTOR('',#44484,10.);
#12468=VECTOR('',#44489,10.);
#12469=VECTOR('',#44492,10.);
#12470=VECTOR('',#44497,10.);
#12471=VECTOR('',#44500,10.);
#12472=VECTOR('',#44505,10.);
#12473=VECTOR('',#44508,10.);
#12474=VECTOR('',#44513,10.);
#12475=VECTOR('',#44516,10.);
#12476=VECTOR('',#44521,10.);
#12477=VECTOR('',#44524,10.);
#12478=VECTOR('',#44529,10.);
#12479=VECTOR('',#44532,10.);
#12480=VECTOR('',#44537,10.);
#12481=VECTOR('',#44540,10.);
#12482=VECTOR('',#44545,10.);
#12483=VECTOR('',#44548,10.);
#12484=VECTOR('',#44553,10.);
#12485=VECTOR('',#44556,10.);
#12486=VECTOR('',#44561,10.);
#12487=VECTOR('',#44564,10.);
#12488=VECTOR('',#44569,10.);
#12489=VECTOR('',#44572,10.);
#12490=VECTOR('',#44577,10.);
#12491=VECTOR('',#44580,10.);
#12492=VECTOR('',#44585,10.);
#12493=VECTOR('',#44588,10.);
#12494=VECTOR('',#44593,10.);
#12495=VECTOR('',#44596,10.);
#12496=VECTOR('',#44601,10.);
#12497=VECTOR('',#44604,10.);
#12498=VECTOR('',#44609,10.);
#12499=VECTOR('',#44612,10.);
#12500=VECTOR('',#44617,10.);
#12501=VECTOR('',#44620,10.);
#12502=VECTOR('',#44625,10.);
#12503=VECTOR('',#44628,10.);
#12504=VECTOR('',#44633,10.);
#12505=VECTOR('',#44636,10.);
#12506=VECTOR('',#44641,10.);
#12507=VECTOR('',#44644,10.);
#12508=VECTOR('',#44649,10.);
#12509=VECTOR('',#44652,10.);
#12510=VECTOR('',#44657,10.);
#12511=VECTOR('',#44660,10.);
#12512=VECTOR('',#44665,10.);
#12513=VECTOR('',#44668,10.);
#12514=VECTOR('',#44673,10.);
#12515=VECTOR('',#44676,10.);
#12516=VECTOR('',#44681,10.);
#12517=VECTOR('',#44684,10.);
#12518=VECTOR('',#44689,10.);
#12519=VECTOR('',#44692,10.);
#12520=VECTOR('',#44697,10.);
#12521=VECTOR('',#44700,10.);
#12522=VECTOR('',#44705,10.);
#12523=VECTOR('',#44708,10.);
#12524=VECTOR('',#44713,10.);
#12525=VECTOR('',#44716,10.);
#12526=VECTOR('',#44721,10.);
#12527=VECTOR('',#44724,10.);
#12528=VECTOR('',#44729,10.);
#12529=VECTOR('',#44732,10.);
#12530=VECTOR('',#44737,10.);
#12531=VECTOR('',#44740,10.);
#12532=VECTOR('',#44745,10.);
#12533=VECTOR('',#44748,10.);
#12534=VECTOR('',#44753,10.);
#12535=VECTOR('',#44756,10.);
#12536=VECTOR('',#44761,10.);
#12537=VECTOR('',#44764,10.);
#12538=VECTOR('',#44769,10.);
#12539=VECTOR('',#44772,10.);
#12540=VECTOR('',#44777,10.);
#12541=VECTOR('',#44780,10.);
#12542=VECTOR('',#44785,10.);
#12543=VECTOR('',#44788,10.);
#12544=VECTOR('',#44793,10.);
#12545=VECTOR('',#44796,10.);
#12546=VECTOR('',#44801,10.);
#12547=VECTOR('',#44804,10.);
#12548=VECTOR('',#44809,10.);
#12549=VECTOR('',#44812,10.);
#12550=VECTOR('',#44817,10.);
#12551=VECTOR('',#44820,10.);
#12552=VECTOR('',#44825,10.);
#12553=VECTOR('',#44828,10.);
#12554=VECTOR('',#44833,10.);
#12555=VECTOR('',#44836,10.);
#12556=VECTOR('',#44841,10.);
#12557=VECTOR('',#44844,10.);
#12558=VECTOR('',#44849,10.);
#12559=VECTOR('',#44852,10.);
#12560=VECTOR('',#44857,10.);
#12561=VECTOR('',#44860,10.);
#12562=VECTOR('',#44865,10.);
#12563=VECTOR('',#44868,10.);
#12564=VECTOR('',#44873,10.);
#12565=VECTOR('',#44876,10.);
#12566=VECTOR('',#44881,10.);
#12567=VECTOR('',#44884,10.);
#12568=VECTOR('',#44889,10.);
#12569=VECTOR('',#44892,10.);
#12570=VECTOR('',#44897,10.);
#12571=VECTOR('',#44900,10.);
#12572=VECTOR('',#44907,10.);
#12573=VECTOR('',#45094,10.);
#12574=VECTOR('',#45097,10.);
#12575=VECTOR('',#45102,10.);
#15111=VERTEX_POINT('',#56406);
#15112=VERTEX_POINT('',#56408);
#15113=VERTEX_POINT('',#56410);
#15114=VERTEX_POINT('',#56414);
#15115=VERTEX_POINT('',#56418);
#15116=VERTEX_POINT('',#56419);
#15117=VERTEX_POINT('',#56421);
#15118=VERTEX_POINT('',#56423);
#15119=VERTEX_POINT('',#56427);
#15120=VERTEX_POINT('',#56431);
#15121=VERTEX_POINT('',#56432);
#15122=VERTEX_POINT('',#56434);
#15123=VERTEX_POINT('',#56436);
#15124=VERTEX_POINT('',#56438);
#15125=VERTEX_POINT('',#56440);
#15126=VERTEX_POINT('',#56442);
#15127=VERTEX_POINT('',#56444);
#15128=VERTEX_POINT('',#56446);
#15129=VERTEX_POINT('',#56448);
#15130=VERTEX_POINT('',#56450);
#15131=VERTEX_POINT('',#56452);
#15132=VERTEX_POINT('',#56454);
#15133=VERTEX_POINT('',#56456);
#15134=VERTEX_POINT('',#56458);
#15135=VERTEX_POINT('',#56460);
#15136=VERTEX_POINT('',#56462);
#15137=VERTEX_POINT('',#56464);
#15138=VERTEX_POINT('',#56466);
#15139=VERTEX_POINT('',#56468);
#15140=VERTEX_POINT('',#56470);
#15141=VERTEX_POINT('',#56472);
#15142=VERTEX_POINT('',#56474);
#15143=VERTEX_POINT('',#56476);
#15144=VERTEX_POINT('',#56478);
#15145=VERTEX_POINT('',#56480);
#15146=VERTEX_POINT('',#56482);
#15147=VERTEX_POINT('',#56484);
#15148=VERTEX_POINT('',#56486);
#15149=VERTEX_POINT('',#56488);
#15150=VERTEX_POINT('',#56490);
#15151=VERTEX_POINT('',#56492);
#15152=VERTEX_POINT('',#56494);
#15153=VERTEX_POINT('',#56496);
#15154=VERTEX_POINT('',#56498);
#15155=VERTEX_POINT('',#56500);
#15156=VERTEX_POINT('',#56502);
#15157=VERTEX_POINT('',#56504);
#15158=VERTEX_POINT('',#56506);
#15159=VERTEX_POINT('',#56508);
#15160=VERTEX_POINT('',#56510);
#15161=VERTEX_POINT('',#56512);
#15162=VERTEX_POINT('',#56514);
#15163=VERTEX_POINT('',#56516);
#15164=VERTEX_POINT('',#56518);
#15165=VERTEX_POINT('',#56520);
#15166=VERTEX_POINT('',#56522);
#15167=VERTEX_POINT('',#56524);
#15168=VERTEX_POINT('',#56526);
#15169=VERTEX_POINT('',#56528);
#15170=VERTEX_POINT('',#56530);
#15171=VERTEX_POINT('',#56532);
#15172=VERTEX_POINT('',#56534);
#15173=VERTEX_POINT('',#56536);
#15174=VERTEX_POINT('',#56538);
#15175=VERTEX_POINT('',#56540);
#15176=VERTEX_POINT('',#56542);
#15177=VERTEX_POINT('',#56544);
#15178=VERTEX_POINT('',#56546);
#15179=VERTEX_POINT('',#56548);
#15180=VERTEX_POINT('',#56550);
#15181=VERTEX_POINT('',#56552);
#15182=VERTEX_POINT('',#56554);
#15183=VERTEX_POINT('',#56556);
#15184=VERTEX_POINT('',#56558);
#15185=VERTEX_POINT('',#56560);
#15186=VERTEX_POINT('',#56562);
#15187=VERTEX_POINT('',#56564);
#15188=VERTEX_POINT('',#56566);
#15189=VERTEX_POINT('',#56568);
#15190=VERTEX_POINT('',#56570);
#15191=VERTEX_POINT('',#56572);
#15192=VERTEX_POINT('',#56574);
#15193=VERTEX_POINT('',#56576);
#15194=VERTEX_POINT('',#56578);
#15195=VERTEX_POINT('',#56580);
#15196=VERTEX_POINT('',#56582);
#15197=VERTEX_POINT('',#56584);
#15198=VERTEX_POINT('',#56586);
#15199=VERTEX_POINT('',#56588);
#15200=VERTEX_POINT('',#56590);
#15201=VERTEX_POINT('',#56592);
#15202=VERTEX_POINT('',#56594);
#15203=VERTEX_POINT('',#56596);
#15204=VERTEX_POINT('',#56598);
#15205=VERTEX_POINT('',#56600);
#15206=VERTEX_POINT('',#56602);
#15207=VERTEX_POINT('',#56604);
#15208=VERTEX_POINT('',#56606);
#15209=VERTEX_POINT('',#56608);
#15210=VERTEX_POINT('',#56610);
#15211=VERTEX_POINT('',#56612);
#15212=VERTEX_POINT('',#56614);
#15213=VERTEX_POINT('',#56616);
#15214=VERTEX_POINT('',#56618);
#15215=VERTEX_POINT('',#56620);
#15216=VERTEX_POINT('',#56622);
#15217=VERTEX_POINT('',#56624);
#15218=VERTEX_POINT('',#56626);
#15219=VERTEX_POINT('',#56628);
#15220=VERTEX_POINT('',#56630);
#15221=VERTEX_POINT('',#56632);
#15222=VERTEX_POINT('',#56634);
#15223=VERTEX_POINT('',#56636);
#15224=VERTEX_POINT('',#56638);
#15225=VERTEX_POINT('',#56640);
#15226=VERTEX_POINT('',#56642);
#15227=VERTEX_POINT('',#56644);
#15228=VERTEX_POINT('',#56646);
#15229=VERTEX_POINT('',#56648);
#15230=VERTEX_POINT('',#56650);
#15231=VERTEX_POINT('',#56652);
#15232=VERTEX_POINT('',#56654);
#15233=VERTEX_POINT('',#56656);
#15234=VERTEX_POINT('',#56658);
#15235=VERTEX_POINT('',#56660);
#15236=VERTEX_POINT('',#56662);
#15237=VERTEX_POINT('',#56664);
#15238=VERTEX_POINT('',#56666);
#15239=VERTEX_POINT('',#56668);
#15240=VERTEX_POINT('',#56670);
#15241=VERTEX_POINT('',#56672);
#15242=VERTEX_POINT('',#56674);
#15243=VERTEX_POINT('',#56676);
#15244=VERTEX_POINT('',#56678);
#15245=VERTEX_POINT('',#56680);
#15246=VERTEX_POINT('',#56682);
#15247=VERTEX_POINT('',#56684);
#15248=VERTEX_POINT('',#56686);
#15249=VERTEX_POINT('',#56688);
#15250=VERTEX_POINT('',#56690);
#15251=VERTEX_POINT('',#56692);
#15252=VERTEX_POINT('',#56694);
#15253=VERTEX_POINT('',#56696);
#15254=VERTEX_POINT('',#56698);
#15255=VERTEX_POINT('',#56700);
#15256=VERTEX_POINT('',#56702);
#15257=VERTEX_POINT('',#56704);
#15258=VERTEX_POINT('',#56706);
#15259=VERTEX_POINT('',#56708);
#15260=VERTEX_POINT('',#56710);
#15261=VERTEX_POINT('',#56712);
#15262=VERTEX_POINT('',#56714);
#15263=VERTEX_POINT('',#56716);
#15264=VERTEX_POINT('',#56718);
#15265=VERTEX_POINT('',#56720);
#15266=VERTEX_POINT('',#56722);
#15267=VERTEX_POINT('',#56724);
#15268=VERTEX_POINT('',#56726);
#15269=VERTEX_POINT('',#56728);
#15270=VERTEX_POINT('',#56730);
#15271=VERTEX_POINT('',#56732);
#15272=VERTEX_POINT('',#56734);
#15273=VERTEX_POINT('',#56736);
#15274=VERTEX_POINT('',#56738);
#15275=VERTEX_POINT('',#56740);
#15276=VERTEX_POINT('',#56742);
#15277=VERTEX_POINT('',#56744);
#15278=VERTEX_POINT('',#56746);
#15279=VERTEX_POINT('',#56748);
#15280=VERTEX_POINT('',#56750);
#15281=VERTEX_POINT('',#56752);
#15282=VERTEX_POINT('',#56754);
#15283=VERTEX_POINT('',#56756);
#15284=VERTEX_POINT('',#56758);
#15285=VERTEX_POINT('',#56760);
#15286=VERTEX_POINT('',#56762);
#15287=VERTEX_POINT('',#56764);
#15288=VERTEX_POINT('',#56766);
#15289=VERTEX_POINT('',#56768);
#15290=VERTEX_POINT('',#56770);
#15291=VERTEX_POINT('',#56772);
#15292=VERTEX_POINT('',#56774);
#15293=VERTEX_POINT('',#56776);
#15294=VERTEX_POINT('',#56778);
#15295=VERTEX_POINT('',#56780);
#15296=VERTEX_POINT('',#56782);
#15297=VERTEX_POINT('',#56784);
#15298=VERTEX_POINT('',#56786);
#15299=VERTEX_POINT('',#56788);
#15300=VERTEX_POINT('',#56790);
#15301=VERTEX_POINT('',#56792);
#15302=VERTEX_POINT('',#56794);
#15303=VERTEX_POINT('',#56796);
#15304=VERTEX_POINT('',#56798);
#15305=VERTEX_POINT('',#56800);
#15306=VERTEX_POINT('',#56802);
#15307=VERTEX_POINT('',#56804);
#15308=VERTEX_POINT('',#56806);
#15309=VERTEX_POINT('',#56808);
#15310=VERTEX_POINT('',#56810);
#15311=VERTEX_POINT('',#56812);
#15312=VERTEX_POINT('',#56816);
#15313=VERTEX_POINT('',#56817);
#15314=VERTEX_POINT('',#56822);
#15315=VERTEX_POINT('',#56826);
#15316=VERTEX_POINT('',#56832);
#15317=VERTEX_POINT('',#56834);
#15318=VERTEX_POINT('',#56838);
#15319=VERTEX_POINT('',#56842);
#15320=VERTEX_POINT('',#56846);
#15321=VERTEX_POINT('',#56848);
#15322=VERTEX_POINT('',#56852);
#15323=VERTEX_POINT('',#56856);
#15324=VERTEX_POINT('',#56860);
#15325=VERTEX_POINT('',#56862);
#15326=VERTEX_POINT('',#56866);
#15327=VERTEX_POINT('',#56870);
#15328=VERTEX_POINT('',#56874);
#15329=VERTEX_POINT('',#56876);
#15330=VERTEX_POINT('',#56880);
#15331=VERTEX_POINT('',#56884);
#15332=VERTEX_POINT('',#56888);
#15333=VERTEX_POINT('',#56890);
#15334=VERTEX_POINT('',#56894);
#15335=VERTEX_POINT('',#56898);
#15336=VERTEX_POINT('',#56902);
#15337=VERTEX_POINT('',#56904);
#15338=VERTEX_POINT('',#56908);
#15339=VERTEX_POINT('',#56912);
#15340=VERTEX_POINT('',#56916);
#15341=VERTEX_POINT('',#56918);
#15342=VERTEX_POINT('',#56922);
#15343=VERTEX_POINT('',#56926);
#15344=VERTEX_POINT('',#56930);
#15345=VERTEX_POINT('',#56932);
#15346=VERTEX_POINT('',#56936);
#15347=VERTEX_POINT('',#56940);
#15348=VERTEX_POINT('',#56944);
#15349=VERTEX_POINT('',#56946);
#15350=VERTEX_POINT('',#56950);
#15351=VERTEX_POINT('',#56954);
#15352=VERTEX_POINT('',#56958);
#15353=VERTEX_POINT('',#56960);
#15354=VERTEX_POINT('',#56964);
#15355=VERTEX_POINT('',#56968);
#15356=VERTEX_POINT('',#56972);
#15357=VERTEX_POINT('',#56974);
#15358=VERTEX_POINT('',#56978);
#15359=VERTEX_POINT('',#56982);
#15360=VERTEX_POINT('',#56986);
#15361=VERTEX_POINT('',#56988);
#15362=VERTEX_POINT('',#56992);
#15363=VERTEX_POINT('',#56996);
#15364=VERTEX_POINT('',#57000);
#15365=VERTEX_POINT('',#57002);
#15366=VERTEX_POINT('',#57006);
#15367=VERTEX_POINT('',#57010);
#15368=VERTEX_POINT('',#57014);
#15369=VERTEX_POINT('',#57016);
#15370=VERTEX_POINT('',#57020);
#15371=VERTEX_POINT('',#57024);
#15372=VERTEX_POINT('',#57028);
#15373=VERTEX_POINT('',#57030);
#15374=VERTEX_POINT('',#57034);
#15375=VERTEX_POINT('',#57038);
#15376=VERTEX_POINT('',#57042);
#15377=VERTEX_POINT('',#57044);
#15378=VERTEX_POINT('',#57048);
#15379=VERTEX_POINT('',#57052);
#15380=VERTEX_POINT('',#57056);
#15381=VERTEX_POINT('',#57058);
#15382=VERTEX_POINT('',#57062);
#15383=VERTEX_POINT('',#57066);
#15384=VERTEX_POINT('',#57070);
#15385=VERTEX_POINT('',#57072);
#15386=VERTEX_POINT('',#57076);
#15387=VERTEX_POINT('',#57080);
#15388=VERTEX_POINT('',#57084);
#15389=VERTEX_POINT('',#57086);
#15390=VERTEX_POINT('',#57090);
#15391=VERTEX_POINT('',#57094);
#15392=VERTEX_POINT('',#57098);
#15393=VERTEX_POINT('',#57100);
#15394=VERTEX_POINT('',#57104);
#15395=VERTEX_POINT('',#57108);
#15396=VERTEX_POINT('',#57112);
#15397=VERTEX_POINT('',#57114);
#15398=VERTEX_POINT('',#57118);
#15399=VERTEX_POINT('',#57122);
#15400=VERTEX_POINT('',#57126);
#15401=VERTEX_POINT('',#57128);
#15402=VERTEX_POINT('',#57132);
#15403=VERTEX_POINT('',#57136);
#15404=VERTEX_POINT('',#57140);
#15405=VERTEX_POINT('',#57142);
#15406=VERTEX_POINT('',#57146);
#15407=VERTEX_POINT('',#57150);
#15408=VERTEX_POINT('',#57154);
#15409=VERTEX_POINT('',#57156);
#15410=VERTEX_POINT('',#57160);
#15411=VERTEX_POINT('',#57164);
#15412=VERTEX_POINT('',#57168);
#15413=VERTEX_POINT('',#57170);
#15414=VERTEX_POINT('',#57174);
#15415=VERTEX_POINT('',#57178);
#15416=VERTEX_POINT('',#57182);
#15417=VERTEX_POINT('',#57184);
#15418=VERTEX_POINT('',#57188);
#15419=VERTEX_POINT('',#57192);
#15420=VERTEX_POINT('',#57196);
#15421=VERTEX_POINT('',#57198);
#15422=VERTEX_POINT('',#57202);
#15423=VERTEX_POINT('',#57206);
#15424=VERTEX_POINT('',#57210);
#15425=VERTEX_POINT('',#57212);
#15426=VERTEX_POINT('',#57216);
#15427=VERTEX_POINT('',#57220);
#15428=VERTEX_POINT('',#57224);
#15429=VERTEX_POINT('',#57226);
#15430=VERTEX_POINT('',#57230);
#15431=VERTEX_POINT('',#57234);
#15432=VERTEX_POINT('',#57238);
#15433=VERTEX_POINT('',#57240);
#15434=VERTEX_POINT('',#57244);
#15435=VERTEX_POINT('',#57248);
#15436=VERTEX_POINT('',#57252);
#15437=VERTEX_POINT('',#57254);
#15438=VERTEX_POINT('',#57258);
#15439=VERTEX_POINT('',#57262);
#15440=VERTEX_POINT('',#57266);
#15441=VERTEX_POINT('',#57268);
#15442=VERTEX_POINT('',#57272);
#15443=VERTEX_POINT('',#57276);
#15444=VERTEX_POINT('',#57280);
#15445=VERTEX_POINT('',#57282);
#15446=VERTEX_POINT('',#57286);
#15447=VERTEX_POINT('',#57290);
#15448=VERTEX_POINT('',#57294);
#15449=VERTEX_POINT('',#57296);
#15450=VERTEX_POINT('',#57300);
#15451=VERTEX_POINT('',#57304);
#15452=VERTEX_POINT('',#57308);
#15453=VERTEX_POINT('',#57310);
#15454=VERTEX_POINT('',#57314);
#15455=VERTEX_POINT('',#57318);
#15456=VERTEX_POINT('',#57322);
#15457=VERTEX_POINT('',#57324);
#15458=VERTEX_POINT('',#57328);
#15459=VERTEX_POINT('',#57332);
#15460=VERTEX_POINT('',#57336);
#15461=VERTEX_POINT('',#57338);
#15462=VERTEX_POINT('',#57342);
#15463=VERTEX_POINT('',#57346);
#15464=VERTEX_POINT('',#57350);
#15465=VERTEX_POINT('',#57352);
#15466=VERTEX_POINT('',#57356);
#15467=VERTEX_POINT('',#57360);
#15468=VERTEX_POINT('',#57364);
#15469=VERTEX_POINT('',#57366);
#15470=VERTEX_POINT('',#57370);
#15471=VERTEX_POINT('',#57374);
#15472=VERTEX_POINT('',#57378);
#15473=VERTEX_POINT('',#57380);
#15474=VERTEX_POINT('',#57384);
#15475=VERTEX_POINT('',#57388);
#15476=VERTEX_POINT('',#57392);
#15477=VERTEX_POINT('',#57394);
#15478=VERTEX_POINT('',#57398);
#15479=VERTEX_POINT('',#57402);
#15480=VERTEX_POINT('',#57406);
#15481=VERTEX_POINT('',#57408);
#15482=VERTEX_POINT('',#57412);
#15483=VERTEX_POINT('',#57416);
#15484=VERTEX_POINT('',#57420);
#15485=VERTEX_POINT('',#57422);
#15486=VERTEX_POINT('',#57426);
#15487=VERTEX_POINT('',#57430);
#15488=VERTEX_POINT('',#57434);
#15489=VERTEX_POINT('',#57436);
#15490=VERTEX_POINT('',#57440);
#15491=VERTEX_POINT('',#57444);
#15492=VERTEX_POINT('',#57448);
#15493=VERTEX_POINT('',#57450);
#15494=VERTEX_POINT('',#57454);
#15495=VERTEX_POINT('',#57458);
#15496=VERTEX_POINT('',#57462);
#15497=VERTEX_POINT('',#57464);
#15498=VERTEX_POINT('',#57468);
#15499=VERTEX_POINT('',#57472);
#15500=VERTEX_POINT('',#57476);
#15501=VERTEX_POINT('',#57478);
#15502=VERTEX_POINT('',#57482);
#15503=VERTEX_POINT('',#57486);
#15504=VERTEX_POINT('',#57490);
#15505=VERTEX_POINT('',#57586);
#15506=VERTEX_POINT('',#57588);
#15507=VERTEX_POINT('',#57592);
#19191=EDGE_CURVE('',#15111,#15111,#3125,.T.);
#19192=EDGE_CURVE('',#15111,#15112,#3126,.T.);
#19193=EDGE_CURVE('',#15112,#15113,#3127,.T.);
#19194=EDGE_CURVE('',#15113,#15112,#3128,.T.);
#19195=EDGE_CURVE('',#15113,#15114,#9826,.T.);
#19196=EDGE_CURVE('',#15114,#15114,#3129,.T.);
#19197=EDGE_CURVE('',#15115,#15116,#9827,.T.);
#19198=EDGE_CURVE('',#15116,#15117,#9828,.T.);
#19199=EDGE_CURVE('',#15117,#15118,#9829,.T.);
#19200=EDGE_CURVE('',#15118,#15115,#3130,.T.);
#19201=EDGE_CURVE('',#15119,#15119,#3131,.T.);
#19202=EDGE_CURVE('',#15119,#15114,#3132,.T.);
#19203=EDGE_CURVE('',#15120,#15121,#3133,.T.);
#19204=EDGE_CURVE('',#15121,#15122,#3134,.T.);
#19205=EDGE_CURVE('',#15122,#15123,#3135,.T.);
#19206=EDGE_CURVE('',#15124,#15123,#3136,.T.);
#19207=EDGE_CURVE('',#15124,#15125,#3137,.T.);
#19208=EDGE_CURVE('',#15125,#15126,#3138,.T.);
#19209=EDGE_CURVE('',#15126,#15127,#3139,.T.);
#19210=EDGE_CURVE('',#15128,#15127,#3140,.T.);
#19211=EDGE_CURVE('',#15128,#15129,#3141,.T.);
#19212=EDGE_CURVE('',#15129,#15130,#3142,.T.);
#19213=EDGE_CURVE('',#15130,#15131,#3143,.T.);
#19214=EDGE_CURVE('',#15132,#15131,#3144,.T.);
#19215=EDGE_CURVE('',#15132,#15133,#3145,.T.);
#19216=EDGE_CURVE('',#15133,#15134,#3146,.T.);
#19217=EDGE_CURVE('',#15134,#15135,#3147,.T.);
#19218=EDGE_CURVE('',#15136,#15135,#3148,.T.);
#19219=EDGE_CURVE('',#15136,#15137,#3149,.T.);
#19220=EDGE_CURVE('',#15137,#15138,#3150,.T.);
#19221=EDGE_CURVE('',#15138,#15139,#3151,.T.);
#19222=EDGE_CURVE('',#15140,#15139,#3152,.T.);
#19223=EDGE_CURVE('',#15140,#15141,#3153,.T.);
#19224=EDGE_CURVE('',#15141,#15142,#3154,.T.);
#19225=EDGE_CURVE('',#15142,#15143,#3155,.T.);
#19226=EDGE_CURVE('',#15144,#15143,#3156,.T.);
#19227=EDGE_CURVE('',#15144,#15145,#3157,.T.);
#19228=EDGE_CURVE('',#15145,#15146,#3158,.T.);
#19229=EDGE_CURVE('',#15146,#15147,#3159,.T.);
#19230=EDGE_CURVE('',#15148,#15147,#3160,.T.);
#19231=EDGE_CURVE('',#15148,#15149,#3161,.T.);
#19232=EDGE_CURVE('',#15149,#15150,#3162,.T.);
#19233=EDGE_CURVE('',#15150,#15151,#3163,.T.);
#19234=EDGE_CURVE('',#15152,#15151,#3164,.T.);
#19235=EDGE_CURVE('',#15152,#15153,#3165,.T.);
#19236=EDGE_CURVE('',#15153,#15154,#3166,.T.);
#19237=EDGE_CURVE('',#15154,#15155,#3167,.T.);
#19238=EDGE_CURVE('',#15156,#15155,#3168,.T.);
#19239=EDGE_CURVE('',#15156,#15157,#3169,.T.);
#19240=EDGE_CURVE('',#15157,#15158,#3170,.T.);
#19241=EDGE_CURVE('',#15158,#15159,#3171,.T.);
#19242=EDGE_CURVE('',#15160,#15159,#3172,.T.);
#19243=EDGE_CURVE('',#15160,#15161,#3173,.T.);
#19244=EDGE_CURVE('',#15161,#15162,#3174,.T.);
#19245=EDGE_CURVE('',#15162,#15163,#3175,.T.);
#19246=EDGE_CURVE('',#15164,#15163,#3176,.T.);
#19247=EDGE_CURVE('',#15164,#15165,#3177,.T.);
#19248=EDGE_CURVE('',#15165,#15166,#3178,.T.);
#19249=EDGE_CURVE('',#15166,#15167,#3179,.T.);
#19250=EDGE_CURVE('',#15168,#15167,#3180,.T.);
#19251=EDGE_CURVE('',#15168,#15169,#3181,.T.);
#19252=EDGE_CURVE('',#15169,#15170,#3182,.T.);
#19253=EDGE_CURVE('',#15170,#15171,#3183,.T.);
#19254=EDGE_CURVE('',#15172,#15171,#3184,.T.);
#19255=EDGE_CURVE('',#15172,#15173,#3185,.T.);
#19256=EDGE_CURVE('',#15173,#15174,#3186,.T.);
#19257=EDGE_CURVE('',#15174,#15175,#3187,.T.);
#19258=EDGE_CURVE('',#15176,#15175,#3188,.T.);
#19259=EDGE_CURVE('',#15176,#15177,#3189,.T.);
#19260=EDGE_CURVE('',#15177,#15178,#3190,.T.);
#19261=EDGE_CURVE('',#15178,#15179,#3191,.T.);
#19262=EDGE_CURVE('',#15180,#15179,#3192,.T.);
#19263=EDGE_CURVE('',#15180,#15181,#3193,.T.);
#19264=EDGE_CURVE('',#15181,#15182,#3194,.T.);
#19265=EDGE_CURVE('',#15182,#15183,#3195,.T.);
#19266=EDGE_CURVE('',#15184,#15183,#3196,.T.);
#19267=EDGE_CURVE('',#15184,#15185,#3197,.T.);
#19268=EDGE_CURVE('',#15185,#15186,#3198,.T.);
#19269=EDGE_CURVE('',#15186,#15187,#3199,.T.);
#19270=EDGE_CURVE('',#15188,#15187,#3200,.T.);
#19271=EDGE_CURVE('',#15188,#15189,#3201,.T.);
#19272=EDGE_CURVE('',#15189,#15190,#3202,.T.);
#19273=EDGE_CURVE('',#15190,#15191,#3203,.T.);
#19274=EDGE_CURVE('',#15192,#15191,#3204,.T.);
#19275=EDGE_CURVE('',#15192,#15193,#3205,.T.);
#19276=EDGE_CURVE('',#15193,#15194,#3206,.T.);
#19277=EDGE_CURVE('',#15194,#15195,#3207,.T.);
#19278=EDGE_CURVE('',#15196,#15195,#3208,.T.);
#19279=EDGE_CURVE('',#15196,#15197,#3209,.T.);
#19280=EDGE_CURVE('',#15197,#15198,#3210,.T.);
#19281=EDGE_CURVE('',#15198,#15199,#3211,.T.);
#19282=EDGE_CURVE('',#15200,#15199,#3212,.T.);
#19283=EDGE_CURVE('',#15200,#15201,#3213,.T.);
#19284=EDGE_CURVE('',#15201,#15202,#3214,.T.);
#19285=EDGE_CURVE('',#15202,#15203,#3215,.T.);
#19286=EDGE_CURVE('',#15204,#15203,#3216,.T.);
#19287=EDGE_CURVE('',#15204,#15205,#3217,.T.);
#19288=EDGE_CURVE('',#15205,#15206,#3218,.T.);
#19289=EDGE_CURVE('',#15206,#15207,#3219,.T.);
#19290=EDGE_CURVE('',#15208,#15207,#3220,.T.);
#19291=EDGE_CURVE('',#15208,#15209,#3221,.T.);
#19292=EDGE_CURVE('',#15209,#15210,#3222,.T.);
#19293=EDGE_CURVE('',#15210,#15211,#3223,.T.);
#19294=EDGE_CURVE('',#15212,#15211,#3224,.T.);
#19295=EDGE_CURVE('',#15212,#15213,#3225,.T.);
#19296=EDGE_CURVE('',#15213,#15214,#3226,.T.);
#19297=EDGE_CURVE('',#15214,#15215,#3227,.T.);
#19298=EDGE_CURVE('',#15216,#15215,#3228,.T.);
#19299=EDGE_CURVE('',#15216,#15217,#3229,.T.);
#19300=EDGE_CURVE('',#15217,#15218,#3230,.T.);
#19301=EDGE_CURVE('',#15218,#15219,#3231,.T.);
#19302=EDGE_CURVE('',#15220,#15219,#3232,.T.);
#19303=EDGE_CURVE('',#15220,#15221,#3233,.T.);
#19304=EDGE_CURVE('',#15221,#15222,#3234,.T.);
#19305=EDGE_CURVE('',#15222,#15223,#3235,.T.);
#19306=EDGE_CURVE('',#15224,#15223,#3236,.T.);
#19307=EDGE_CURVE('',#15224,#15225,#3237,.T.);
#19308=EDGE_CURVE('',#15225,#15226,#3238,.T.);
#19309=EDGE_CURVE('',#15226,#15227,#3239,.T.);
#19310=EDGE_CURVE('',#15228,#15227,#3240,.T.);
#19311=EDGE_CURVE('',#15228,#15229,#3241,.T.);
#19312=EDGE_CURVE('',#15229,#15230,#3242,.T.);
#19313=EDGE_CURVE('',#15230,#15231,#3243,.T.);
#19314=EDGE_CURVE('',#15232,#15231,#3244,.T.);
#19315=EDGE_CURVE('',#15232,#15233,#3245,.T.);
#19316=EDGE_CURVE('',#15233,#15234,#3246,.T.);
#19317=EDGE_CURVE('',#15234,#15235,#3247,.T.);
#19318=EDGE_CURVE('',#15236,#15235,#3248,.T.);
#19319=EDGE_CURVE('',#15236,#15237,#3249,.T.);
#19320=EDGE_CURVE('',#15237,#15238,#3250,.T.);
#19321=EDGE_CURVE('',#15238,#15239,#3251,.T.);
#19322=EDGE_CURVE('',#15240,#15239,#3252,.T.);
#19323=EDGE_CURVE('',#15240,#15241,#3253,.T.);
#19324=EDGE_CURVE('',#15241,#15242,#3254,.T.);
#19325=EDGE_CURVE('',#15242,#15243,#3255,.T.);
#19326=EDGE_CURVE('',#15244,#15243,#3256,.T.);
#19327=EDGE_CURVE('',#15244,#15245,#3257,.T.);
#19328=EDGE_CURVE('',#15245,#15246,#3258,.T.);
#19329=EDGE_CURVE('',#15246,#15247,#3259,.T.);
#19330=EDGE_CURVE('',#15248,#15247,#3260,.T.);
#19331=EDGE_CURVE('',#15248,#15249,#3261,.T.);
#19332=EDGE_CURVE('',#15249,#15250,#3262,.T.);
#19333=EDGE_CURVE('',#15250,#15251,#3263,.T.);
#19334=EDGE_CURVE('',#15252,#15251,#3264,.T.);
#19335=EDGE_CURVE('',#15252,#15253,#3265,.T.);
#19336=EDGE_CURVE('',#15253,#15254,#3266,.T.);
#19337=EDGE_CURVE('',#15254,#15255,#3267,.T.);
#19338=EDGE_CURVE('',#15256,#15255,#3268,.T.);
#19339=EDGE_CURVE('',#15256,#15257,#3269,.T.);
#19340=EDGE_CURVE('',#15257,#15258,#3270,.T.);
#19341=EDGE_CURVE('',#15258,#15259,#3271,.T.);
#19342=EDGE_CURVE('',#15260,#15259,#3272,.T.);
#19343=EDGE_CURVE('',#15260,#15261,#3273,.T.);
#19344=EDGE_CURVE('',#15261,#15262,#3274,.T.);
#19345=EDGE_CURVE('',#15262,#15263,#3275,.T.);
#19346=EDGE_CURVE('',#15264,#15263,#3276,.T.);
#19347=EDGE_CURVE('',#15264,#15265,#3277,.T.);
#19348=EDGE_CURVE('',#15265,#15266,#3278,.T.);
#19349=EDGE_CURVE('',#15266,#15267,#3279,.T.);
#19350=EDGE_CURVE('',#15268,#15267,#3280,.T.);
#19351=EDGE_CURVE('',#15268,#15269,#3281,.T.);
#19352=EDGE_CURVE('',#15269,#15270,#3282,.T.);
#19353=EDGE_CURVE('',#15270,#15271,#3283,.T.);
#19354=EDGE_CURVE('',#15272,#15271,#3284,.T.);
#19355=EDGE_CURVE('',#15272,#15273,#3285,.T.);
#19356=EDGE_CURVE('',#15273,#15274,#3286,.T.);
#19357=EDGE_CURVE('',#15274,#15275,#3287,.T.);
#19358=EDGE_CURVE('',#15276,#15275,#3288,.T.);
#19359=EDGE_CURVE('',#15276,#15277,#3289,.T.);
#19360=EDGE_CURVE('',#15277,#15278,#3290,.T.);
#19361=EDGE_CURVE('',#15278,#15279,#3291,.T.);
#19362=EDGE_CURVE('',#15280,#15279,#3292,.T.);
#19363=EDGE_CURVE('',#15280,#15281,#3293,.T.);
#19364=EDGE_CURVE('',#15281,#15282,#3294,.T.);
#19365=EDGE_CURVE('',#15282,#15283,#3295,.T.);
#19366=EDGE_CURVE('',#15284,#15283,#3296,.T.);
#19367=EDGE_CURVE('',#15284,#15285,#3297,.T.);
#19368=EDGE_CURVE('',#15285,#15286,#3298,.T.);
#19369=EDGE_CURVE('',#15286,#15287,#3299,.T.);
#19370=EDGE_CURVE('',#15288,#15287,#3300,.T.);
#19371=EDGE_CURVE('',#15288,#15289,#3301,.T.);
#19372=EDGE_CURVE('',#15289,#15290,#3302,.T.);
#19373=EDGE_CURVE('',#15290,#15291,#3303,.T.);
#19374=EDGE_CURVE('',#15292,#15291,#3304,.T.);
#19375=EDGE_CURVE('',#15292,#15293,#3305,.T.);
#19376=EDGE_CURVE('',#15293,#15294,#3306,.T.);
#19377=EDGE_CURVE('',#15294,#15295,#3307,.T.);
#19378=EDGE_CURVE('',#15296,#15295,#3308,.T.);
#19379=EDGE_CURVE('',#15296,#15297,#3309,.T.);
#19380=EDGE_CURVE('',#15297,#15298,#3310,.T.);
#19381=EDGE_CURVE('',#15298,#15299,#3311,.T.);
#19382=EDGE_CURVE('',#15300,#15299,#3312,.T.);
#19383=EDGE_CURVE('',#15300,#15301,#3313,.T.);
#19384=EDGE_CURVE('',#15301,#15302,#3314,.T.);
#19385=EDGE_CURVE('',#15302,#15303,#3315,.T.);
#19386=EDGE_CURVE('',#15304,#15303,#3316,.T.);
#19387=EDGE_CURVE('',#15304,#15305,#3317,.T.);
#19388=EDGE_CURVE('',#15305,#15306,#3318,.T.);
#19389=EDGE_CURVE('',#15306,#15307,#3319,.T.);
#19390=EDGE_CURVE('',#15308,#15307,#3320,.T.);
#19391=EDGE_CURVE('',#15308,#15309,#3321,.T.);
#19392=EDGE_CURVE('',#15309,#15310,#3322,.T.);
#19393=EDGE_CURVE('',#15310,#15311,#3323,.T.);
#19394=EDGE_CURVE('',#15120,#15311,#3324,.T.);
#19395=EDGE_CURVE('',#15312,#15313,#9830,.T.);
#19396=EDGE_CURVE('',#15117,#15312,#9831,.T.);
#19397=EDGE_CURVE('',#15116,#15313,#9832,.T.);
#19398=EDGE_CURVE('',#15313,#15314,#9833,.T.);
#19399=EDGE_CURVE('',#15314,#15115,#9834,.T.);
#19400=EDGE_CURVE('',#15314,#15315,#3325,.T.);
#19401=EDGE_CURVE('',#15118,#15315,#9835,.T.);
#19402=EDGE_CURVE('',#15315,#15312,#9836,.T.);
#19403=EDGE_CURVE('',#15316,#15121,#9837,.T.);
#19404=EDGE_CURVE('',#15317,#15316,#3326,.T.);
#19405=EDGE_CURVE('',#15317,#15122,#9838,.T.);
#19406=EDGE_CURVE('',#15318,#15317,#3327,.T.);
#19407=EDGE_CURVE('',#15123,#15318,#9839,.T.);
#19408=EDGE_CURVE('',#15319,#15120,#9840,.T.);
#19409=EDGE_CURVE('',#15316,#15319,#3328,.T.);
#19410=EDGE_CURVE('',#15320,#15125,#9841,.T.);
#19411=EDGE_CURVE('',#15321,#15320,#3329,.T.);
#19412=EDGE_CURVE('',#15321,#15126,#9842,.T.);
#19413=EDGE_CURVE('',#15322,#15321,#3330,.T.);
#19414=EDGE_CURVE('',#15127,#15322,#9843,.T.);
#19415=EDGE_CURVE('',#15323,#15124,#9844,.T.);
#19416=EDGE_CURVE('',#15320,#15323,#3331,.T.);
#19417=EDGE_CURVE('',#15324,#15129,#9845,.T.);
#19418=EDGE_CURVE('',#15325,#15324,#3332,.T.);
#19419=EDGE_CURVE('',#15325,#15130,#9846,.T.);
#19420=EDGE_CURVE('',#15326,#15325,#3333,.T.);
#19421=EDGE_CURVE('',#15131,#15326,#9847,.T.);
#19422=EDGE_CURVE('',#15327,#15128,#9848,.T.);
#19423=EDGE_CURVE('',#15324,#15327,#3334,.T.);
#19424=EDGE_CURVE('',#15328,#15133,#9849,.T.);
#19425=EDGE_CURVE('',#15329,#15328,#3335,.T.);
#19426=EDGE_CURVE('',#15329,#15134,#9850,.T.);
#19427=EDGE_CURVE('',#15330,#15329,#3336,.T.);
#19428=EDGE_CURVE('',#15135,#15330,#9851,.T.);
#19429=EDGE_CURVE('',#15331,#15132,#9852,.T.);
#19430=EDGE_CURVE('',#15328,#15331,#3337,.T.);
#19431=EDGE_CURVE('',#15332,#15137,#9853,.T.);
#19432=EDGE_CURVE('',#15333,#15332,#3338,.T.);
#19433=EDGE_CURVE('',#15333,#15138,#9854,.T.);
#19434=EDGE_CURVE('',#15334,#15333,#3339,.T.);
#19435=EDGE_CURVE('',#15139,#15334,#9855,.T.);
#19436=EDGE_CURVE('',#15335,#15136,#9856,.T.);
#19437=EDGE_CURVE('',#15332,#15335,#3340,.T.);
#19438=EDGE_CURVE('',#15336,#15141,#9857,.T.);
#19439=EDGE_CURVE('',#15337,#15336,#3341,.T.);
#19440=EDGE_CURVE('',#15337,#15142,#9858,.T.);
#19441=EDGE_CURVE('',#15338,#15337,#3342,.T.);
#19442=EDGE_CURVE('',#15143,#15338,#9859,.T.);
#19443=EDGE_CURVE('',#15339,#15140,#9860,.T.);
#19444=EDGE_CURVE('',#15336,#15339,#3343,.T.);
#19445=EDGE_CURVE('',#15340,#15145,#9861,.T.);
#19446=EDGE_CURVE('',#15341,#15340,#3344,.T.);
#19447=EDGE_CURVE('',#15341,#15146,#9862,.T.);
#19448=EDGE_CURVE('',#15342,#15341,#3345,.T.);
#19449=EDGE_CURVE('',#15147,#15342,#9863,.T.);
#19450=EDGE_CURVE('',#15343,#15144,#9864,.T.);
#19451=EDGE_CURVE('',#15340,#15343,#3346,.T.);
#19452=EDGE_CURVE('',#15344,#15149,#9865,.T.);
#19453=EDGE_CURVE('',#15345,#15344,#3347,.T.);
#19454=EDGE_CURVE('',#15345,#15150,#9866,.T.);
#19455=EDGE_CURVE('',#15346,#15345,#3348,.T.);
#19456=EDGE_CURVE('',#15151,#15346,#9867,.T.);
#19457=EDGE_CURVE('',#15347,#15148,#9868,.T.);
#19458=EDGE_CURVE('',#15344,#15347,#3349,.T.);
#19459=EDGE_CURVE('',#15348,#15153,#9869,.T.);
#19460=EDGE_CURVE('',#15349,#15348,#3350,.T.);
#19461=EDGE_CURVE('',#15349,#15154,#9870,.T.);
#19462=EDGE_CURVE('',#15350,#15349,#3351,.T.);
#19463=EDGE_CURVE('',#15155,#15350,#9871,.T.);
#19464=EDGE_CURVE('',#15351,#15152,#9872,.T.);
#19465=EDGE_CURVE('',#15348,#15351,#3352,.T.);
#19466=EDGE_CURVE('',#15352,#15157,#9873,.T.);
#19467=EDGE_CURVE('',#15353,#15352,#3353,.T.);
#19468=EDGE_CURVE('',#15353,#15158,#9874,.T.);
#19469=EDGE_CURVE('',#15354,#15353,#3354,.T.);
#19470=EDGE_CURVE('',#15159,#15354,#9875,.T.);
#19471=EDGE_CURVE('',#15355,#15156,#9876,.T.);
#19472=EDGE_CURVE('',#15352,#15355,#3355,.T.);
#19473=EDGE_CURVE('',#15356,#15161,#9877,.T.);
#19474=EDGE_CURVE('',#15357,#15356,#3356,.T.);
#19475=EDGE_CURVE('',#15357,#15162,#9878,.T.);
#19476=EDGE_CURVE('',#15358,#15357,#3357,.T.);
#19477=EDGE_CURVE('',#15163,#15358,#9879,.T.);
#19478=EDGE_CURVE('',#15359,#15160,#9880,.T.);
#19479=EDGE_CURVE('',#15356,#15359,#3358,.T.);
#19480=EDGE_CURVE('',#15360,#15165,#9881,.T.);
#19481=EDGE_CURVE('',#15361,#15360,#3359,.T.);
#19482=EDGE_CURVE('',#15361,#15166,#9882,.T.);
#19483=EDGE_CURVE('',#15362,#15361,#3360,.T.);
#19484=EDGE_CURVE('',#15167,#15362,#9883,.T.);
#19485=EDGE_CURVE('',#15363,#15164,#9884,.T.);
#19486=EDGE_CURVE('',#15360,#15363,#3361,.T.);
#19487=EDGE_CURVE('',#15364,#15169,#9885,.T.);
#19488=EDGE_CURVE('',#15365,#15364,#3362,.T.);
#19489=EDGE_CURVE('',#15365,#15170,#9886,.T.);
#19490=EDGE_CURVE('',#15366,#15365,#3363,.T.);
#19491=EDGE_CURVE('',#15171,#15366,#9887,.T.);
#19492=EDGE_CURVE('',#15367,#15168,#9888,.T.);
#19493=EDGE_CURVE('',#15364,#15367,#3364,.T.);
#19494=EDGE_CURVE('',#15368,#15173,#9889,.T.);
#19495=EDGE_CURVE('',#15369,#15368,#3365,.T.);
#19496=EDGE_CURVE('',#15369,#15174,#9890,.T.);
#19497=EDGE_CURVE('',#15370,#15369,#3366,.T.);
#19498=EDGE_CURVE('',#15175,#15370,#9891,.T.);
#19499=EDGE_CURVE('',#15371,#15172,#9892,.T.);
#19500=EDGE_CURVE('',#15368,#15371,#3367,.T.);
#19501=EDGE_CURVE('',#15372,#15177,#9893,.T.);
#19502=EDGE_CURVE('',#15373,#15372,#3368,.T.);
#19503=EDGE_CURVE('',#15373,#15178,#9894,.T.);
#19504=EDGE_CURVE('',#15374,#15373,#3369,.T.);
#19505=EDGE_CURVE('',#15179,#15374,#9895,.T.);
#19506=EDGE_CURVE('',#15375,#15176,#9896,.T.);
#19507=EDGE_CURVE('',#15372,#15375,#3370,.T.);
#19508=EDGE_CURVE('',#15376,#15181,#9897,.T.);
#19509=EDGE_CURVE('',#15377,#15376,#3371,.T.);
#19510=EDGE_CURVE('',#15377,#15182,#9898,.T.);
#19511=EDGE_CURVE('',#15378,#15377,#3372,.T.);
#19512=EDGE_CURVE('',#15183,#15378,#9899,.T.);
#19513=EDGE_CURVE('',#15379,#15180,#9900,.T.);
#19514=EDGE_CURVE('',#15376,#15379,#3373,.T.);
#19515=EDGE_CURVE('',#15380,#15185,#9901,.T.);
#19516=EDGE_CURVE('',#15381,#15380,#3374,.T.);
#19517=EDGE_CURVE('',#15381,#15186,#9902,.T.);
#19518=EDGE_CURVE('',#15382,#15381,#3375,.T.);
#19519=EDGE_CURVE('',#15187,#15382,#9903,.T.);
#19520=EDGE_CURVE('',#15383,#15184,#9904,.T.);
#19521=EDGE_CURVE('',#15380,#15383,#3376,.T.);
#19522=EDGE_CURVE('',#15384,#15189,#9905,.T.);
#19523=EDGE_CURVE('',#15385,#15384,#3377,.T.);
#19524=EDGE_CURVE('',#15385,#15190,#9906,.T.);
#19525=EDGE_CURVE('',#15386,#15385,#3378,.T.);
#19526=EDGE_CURVE('',#15191,#15386,#9907,.T.);
#19527=EDGE_CURVE('',#15387,#15188,#9908,.T.);
#19528=EDGE_CURVE('',#15384,#15387,#3379,.T.);
#19529=EDGE_CURVE('',#15388,#15193,#9909,.T.);
#19530=EDGE_CURVE('',#15389,#15388,#3380,.T.);
#19531=EDGE_CURVE('',#15389,#15194,#9910,.T.);
#19532=EDGE_CURVE('',#15390,#15389,#3381,.T.);
#19533=EDGE_CURVE('',#15195,#15390,#9911,.T.);
#19534=EDGE_CURVE('',#15391,#15192,#9912,.T.);
#19535=EDGE_CURVE('',#15388,#15391,#3382,.T.);
#19536=EDGE_CURVE('',#15392,#15197,#9913,.T.);
#19537=EDGE_CURVE('',#15393,#15392,#3383,.T.);
#19538=EDGE_CURVE('',#15393,#15198,#9914,.T.);
#19539=EDGE_CURVE('',#15394,#15393,#3384,.T.);
#19540=EDGE_CURVE('',#15199,#15394,#9915,.T.);
#19541=EDGE_CURVE('',#15395,#15196,#9916,.T.);
#19542=EDGE_CURVE('',#15392,#15395,#3385,.T.);
#19543=EDGE_CURVE('',#15396,#15201,#9917,.T.);
#19544=EDGE_CURVE('',#15397,#15396,#3386,.T.);
#19545=EDGE_CURVE('',#15397,#15202,#9918,.T.);
#19546=EDGE_CURVE('',#15398,#15397,#3387,.T.);
#19547=EDGE_CURVE('',#15203,#15398,#9919,.T.);
#19548=EDGE_CURVE('',#15399,#15200,#9920,.T.);
#19549=EDGE_CURVE('',#15396,#15399,#3388,.T.);
#19550=EDGE_CURVE('',#15400,#15205,#9921,.T.);
#19551=EDGE_CURVE('',#15401,#15400,#3389,.T.);
#19552=EDGE_CURVE('',#15401,#15206,#9922,.T.);
#19553=EDGE_CURVE('',#15402,#15401,#3390,.T.);
#19554=EDGE_CURVE('',#15207,#15402,#9923,.T.);
#19555=EDGE_CURVE('',#15403,#15204,#9924,.T.);
#19556=EDGE_CURVE('',#15400,#15403,#3391,.T.);
#19557=EDGE_CURVE('',#15404,#15209,#9925,.T.);
#19558=EDGE_CURVE('',#15405,#15404,#3392,.T.);
#19559=EDGE_CURVE('',#15405,#15210,#9926,.T.);
#19560=EDGE_CURVE('',#15406,#15405,#3393,.T.);
#19561=EDGE_CURVE('',#15211,#15406,#9927,.T.);
#19562=EDGE_CURVE('',#15407,#15208,#9928,.T.);
#19563=EDGE_CURVE('',#15404,#15407,#3394,.T.);
#19564=EDGE_CURVE('',#15408,#15213,#9929,.T.);
#19565=EDGE_CURVE('',#15409,#15408,#3395,.T.);
#19566=EDGE_CURVE('',#15409,#15214,#9930,.T.);
#19567=EDGE_CURVE('',#15410,#15409,#3396,.T.);
#19568=EDGE_CURVE('',#15215,#15410,#9931,.T.);
#19569=EDGE_CURVE('',#15411,#15212,#9932,.T.);
#19570=EDGE_CURVE('',#15408,#15411,#3397,.T.);
#19571=EDGE_CURVE('',#15412,#15217,#9933,.T.);
#19572=EDGE_CURVE('',#15413,#15412,#3398,.T.);
#19573=EDGE_CURVE('',#15413,#15218,#9934,.T.);
#19574=EDGE_CURVE('',#15414,#15413,#3399,.T.);
#19575=EDGE_CURVE('',#15219,#15414,#9935,.T.);
#19576=EDGE_CURVE('',#15415,#15216,#9936,.T.);
#19577=EDGE_CURVE('',#15412,#15415,#3400,.T.);
#19578=EDGE_CURVE('',#15416,#15221,#9937,.T.);
#19579=EDGE_CURVE('',#15417,#15416,#3401,.T.);
#19580=EDGE_CURVE('',#15417,#15222,#9938,.T.);
#19581=EDGE_CURVE('',#15418,#15417,#3402,.T.);
#19582=EDGE_CURVE('',#15223,#15418,#9939,.T.);
#19583=EDGE_CURVE('',#15419,#15220,#9940,.T.);
#19584=EDGE_CURVE('',#15416,#15419,#3403,.T.);
#19585=EDGE_CURVE('',#15420,#15225,#9941,.T.);
#19586=EDGE_CURVE('',#15421,#15420,#3404,.T.);
#19587=EDGE_CURVE('',#15421,#15226,#9942,.T.);
#19588=EDGE_CURVE('',#15422,#15421,#3405,.T.);
#19589=EDGE_CURVE('',#15227,#15422,#9943,.T.);
#19590=EDGE_CURVE('',#15423,#15224,#9944,.T.);
#19591=EDGE_CURVE('',#15420,#15423,#3406,.T.);
#19592=EDGE_CURVE('',#15424,#15229,#9945,.T.);
#19593=EDGE_CURVE('',#15425,#15424,#3407,.T.);
#19594=EDGE_CURVE('',#15425,#15230,#9946,.T.);
#19595=EDGE_CURVE('',#15426,#15425,#3408,.T.);
#19596=EDGE_CURVE('',#15231,#15426,#9947,.T.);
#19597=EDGE_CURVE('',#15427,#15228,#9948,.T.);
#19598=EDGE_CURVE('',#15424,#15427,#3409,.T.);
#19599=EDGE_CURVE('',#15428,#15233,#9949,.T.);
#19600=EDGE_CURVE('',#15429,#15428,#3410,.T.);
#19601=EDGE_CURVE('',#15429,#15234,#9950,.T.);
#19602=EDGE_CURVE('',#15430,#15429,#3411,.T.);
#19603=EDGE_CURVE('',#15235,#15430,#9951,.T.);
#19604=EDGE_CURVE('',#15431,#15232,#9952,.T.);
#19605=EDGE_CURVE('',#15428,#15431,#3412,.T.);
#19606=EDGE_CURVE('',#15432,#15237,#9953,.T.);
#19607=EDGE_CURVE('',#15433,#15432,#3413,.T.);
#19608=EDGE_CURVE('',#15433,#15238,#9954,.T.);
#19609=EDGE_CURVE('',#15434,#15433,#3414,.T.);
#19610=EDGE_CURVE('',#15239,#15434,#9955,.T.);
#19611=EDGE_CURVE('',#15435,#15236,#9956,.T.);
#19612=EDGE_CURVE('',#15432,#15435,#3415,.T.);
#19613=EDGE_CURVE('',#15436,#15241,#9957,.T.);
#19614=EDGE_CURVE('',#15437,#15436,#3416,.T.);
#19615=EDGE_CURVE('',#15437,#15242,#9958,.T.);
#19616=EDGE_CURVE('',#15438,#15437,#3417,.T.);
#19617=EDGE_CURVE('',#15243,#15438,#9959,.T.);
#19618=EDGE_CURVE('',#15439,#15240,#9960,.T.);
#19619=EDGE_CURVE('',#15436,#15439,#3418,.T.);
#19620=EDGE_CURVE('',#15440,#15245,#9961,.T.);
#19621=EDGE_CURVE('',#15441,#15440,#3419,.T.);
#19622=EDGE_CURVE('',#15441,#15246,#9962,.T.);
#19623=EDGE_CURVE('',#15442,#15441,#3420,.T.);
#19624=EDGE_CURVE('',#15247,#15442,#9963,.T.);
#19625=EDGE_CURVE('',#15443,#15244,#9964,.T.);
#19626=EDGE_CURVE('',#15440,#15443,#3421,.T.);
#19627=EDGE_CURVE('',#15444,#15249,#9965,.T.);
#19628=EDGE_CURVE('',#15445,#15444,#3422,.T.);
#19629=EDGE_CURVE('',#15445,#15250,#9966,.T.);
#19630=EDGE_CURVE('',#15446,#15445,#3423,.T.);
#19631=EDGE_CURVE('',#15251,#15446,#9967,.T.);
#19632=EDGE_CURVE('',#15447,#15248,#9968,.T.);
#19633=EDGE_CURVE('',#15444,#15447,#3424,.T.);
#19634=EDGE_CURVE('',#15448,#15253,#9969,.T.);
#19635=EDGE_CURVE('',#15449,#15448,#3425,.T.);
#19636=EDGE_CURVE('',#15449,#15254,#9970,.T.);
#19637=EDGE_CURVE('',#15450,#15449,#3426,.T.);
#19638=EDGE_CURVE('',#15255,#15450,#9971,.T.);
#19639=EDGE_CURVE('',#15451,#15252,#9972,.T.);
#19640=EDGE_CURVE('',#15448,#15451,#3427,.T.);
#19641=EDGE_CURVE('',#15452,#15257,#9973,.T.);
#19642=EDGE_CURVE('',#15453,#15452,#3428,.T.);
#19643=EDGE_CURVE('',#15453,#15258,#9974,.T.);
#19644=EDGE_CURVE('',#15454,#15453,#3429,.T.);
#19645=EDGE_CURVE('',#15259,#15454,#9975,.T.);
#19646=EDGE_CURVE('',#15455,#15256,#9976,.T.);
#19647=EDGE_CURVE('',#15452,#15455,#3430,.T.);
#19648=EDGE_CURVE('',#15456,#15261,#9977,.T.);
#19649=EDGE_CURVE('',#15457,#15456,#3431,.T.);
#19650=EDGE_CURVE('',#15457,#15262,#9978,.T.);
#19651=EDGE_CURVE('',#15458,#15457,#3432,.T.);
#19652=EDGE_CURVE('',#15263,#15458,#9979,.T.);
#19653=EDGE_CURVE('',#15459,#15260,#9980,.T.);
#19654=EDGE_CURVE('',#15456,#15459,#3433,.T.);
#19655=EDGE_CURVE('',#15460,#15265,#9981,.T.);
#19656=EDGE_CURVE('',#15461,#15460,#3434,.T.);
#19657=EDGE_CURVE('',#15461,#15266,#9982,.T.);
#19658=EDGE_CURVE('',#15462,#15461,#3435,.T.);
#19659=EDGE_CURVE('',#15267,#15462,#9983,.T.);
#19660=EDGE_CURVE('',#15463,#15264,#9984,.T.);
#19661=EDGE_CURVE('',#15460,#15463,#3436,.T.);
#19662=EDGE_CURVE('',#15464,#15269,#9985,.T.);
#19663=EDGE_CURVE('',#15465,#15464,#3437,.T.);
#19664=EDGE_CURVE('',#15465,#15270,#9986,.T.);
#19665=EDGE_CURVE('',#15466,#15465,#3438,.T.);
#19666=EDGE_CURVE('',#15271,#15466,#9987,.T.);
#19667=EDGE_CURVE('',#15467,#15268,#9988,.T.);
#19668=EDGE_CURVE('',#15464,#15467,#3439,.T.);
#19669=EDGE_CURVE('',#15468,#15273,#9989,.T.);
#19670=EDGE_CURVE('',#15469,#15468,#3440,.T.);
#19671=EDGE_CURVE('',#15469,#15274,#9990,.T.);
#19672=EDGE_CURVE('',#15470,#15469,#3441,.T.);
#19673=EDGE_CURVE('',#15275,#15470,#9991,.T.);
#19674=EDGE_CURVE('',#15471,#15272,#9992,.T.);
#19675=EDGE_CURVE('',#15468,#15471,#3442,.T.);
#19676=EDGE_CURVE('',#15472,#15277,#9993,.T.);
#19677=EDGE_CURVE('',#15473,#15472,#3443,.T.);
#19678=EDGE_CURVE('',#15473,#15278,#9994,.T.);
#19679=EDGE_CURVE('',#15474,#15473,#3444,.T.);
#19680=EDGE_CURVE('',#15279,#15474,#9995,.T.);
#19681=EDGE_CURVE('',#15475,#15276,#9996,.T.);
#19682=EDGE_CURVE('',#15472,#15475,#3445,.T.);
#19683=EDGE_CURVE('',#15476,#15281,#9997,.T.);
#19684=EDGE_CURVE('',#15477,#15476,#3446,.T.);
#19685=EDGE_CURVE('',#15477,#15282,#9998,.T.);
#19686=EDGE_CURVE('',#15478,#15477,#3447,.T.);
#19687=EDGE_CURVE('',#15283,#15478,#9999,.T.);
#19688=EDGE_CURVE('',#15479,#15280,#10000,.T.);
#19689=EDGE_CURVE('',#15476,#15479,#3448,.T.);
#19690=EDGE_CURVE('',#15480,#15285,#10001,.T.);
#19691=EDGE_CURVE('',#15481,#15480,#3449,.T.);
#19692=EDGE_CURVE('',#15481,#15286,#10002,.T.);
#19693=EDGE_CURVE('',#15482,#15481,#3450,.T.);
#19694=EDGE_CURVE('',#15287,#15482,#10003,.T.);
#19695=EDGE_CURVE('',#15483,#15284,#10004,.T.);
#19696=EDGE_CURVE('',#15480,#15483,#3451,.T.);
#19697=EDGE_CURVE('',#15484,#15289,#10005,.T.);
#19698=EDGE_CURVE('',#15485,#15484,#3452,.T.);
#19699=EDGE_CURVE('',#15485,#15290,#10006,.T.);
#19700=EDGE_CURVE('',#15486,#15485,#3453,.T.);
#19701=EDGE_CURVE('',#15291,#15486,#10007,.T.);
#19702=EDGE_CURVE('',#15487,#15288,#10008,.T.);
#19703=EDGE_CURVE('',#15484,#15487,#3454,.T.);
#19704=EDGE_CURVE('',#15488,#15293,#10009,.T.);
#19705=EDGE_CURVE('',#15489,#15488,#3455,.T.);
#19706=EDGE_CURVE('',#15489,#15294,#10010,.T.);
#19707=EDGE_CURVE('',#15490,#15489,#3456,.T.);
#19708=EDGE_CURVE('',#15295,#15490,#10011,.T.);
#19709=EDGE_CURVE('',#15491,#15292,#10012,.T.);
#19710=EDGE_CURVE('',#15488,#15491,#3457,.T.);
#19711=EDGE_CURVE('',#15492,#15297,#10013,.T.);
#19712=EDGE_CURVE('',#15493,#15492,#3458,.T.);
#19713=EDGE_CURVE('',#15493,#15298,#10014,.T.);
#19714=EDGE_CURVE('',#15494,#15493,#3459,.T.);
#19715=EDGE_CURVE('',#15299,#15494,#10015,.T.);
#19716=EDGE_CURVE('',#15495,#15296,#10016,.T.);
#19717=EDGE_CURVE('',#15492,#15495,#3460,.T.);
#19718=EDGE_CURVE('',#15496,#15301,#10017,.T.);
#19719=EDGE_CURVE('',#15497,#15496,#3461,.T.);
#19720=EDGE_CURVE('',#15497,#15302,#10018,.T.);
#19721=EDGE_CURVE('',#15498,#15497,#3462,.T.);
#19722=EDGE_CURVE('',#15303,#15498,#10019,.T.);
#19723=EDGE_CURVE('',#15499,#15300,#10020,.T.);
#19724=EDGE_CURVE('',#15496,#15499,#3463,.T.);
#19725=EDGE_CURVE('',#15500,#15305,#10021,.T.);
#19726=EDGE_CURVE('',#15501,#15500,#3464,.T.);
#19727=EDGE_CURVE('',#15501,#15306,#10022,.T.);
#19728=EDGE_CURVE('',#15502,#15501,#3465,.T.);
#19729=EDGE_CURVE('',#15307,#15502,#10023,.T.);
#19730=EDGE_CURVE('',#15503,#15304,#10024,.T.);
#19731=EDGE_CURVE('',#15500,#15503,#3466,.T.);
#19732=EDGE_CURVE('',#15504,#15502,#3467,.T.);
#19733=EDGE_CURVE('',#15504,#15308,#10025,.T.);
#19734=EDGE_CURVE('',#15503,#15498,#3468,.T.);
#19735=EDGE_CURVE('',#15499,#15494,#3469,.T.);
#19736=EDGE_CURVE('',#15495,#15490,#3470,.T.);
#19737=EDGE_CURVE('',#15491,#15486,#3471,.T.);
#19738=EDGE_CURVE('',#15487,#15482,#3472,.T.);
#19739=EDGE_CURVE('',#15483,#15478,#3473,.T.);
#19740=EDGE_CURVE('',#15479,#15474,#3474,.T.);
#19741=EDGE_CURVE('',#15475,#15470,#3475,.T.);
#19742=EDGE_CURVE('',#15471,#15466,#3476,.T.);
#19743=EDGE_CURVE('',#15467,#15462,#3477,.T.);
#19744=EDGE_CURVE('',#15463,#15458,#3478,.T.);
#19745=EDGE_CURVE('',#15459,#15454,#3479,.T.);
#19746=EDGE_CURVE('',#15455,#15450,#3480,.T.);
#19747=EDGE_CURVE('',#15451,#15446,#3481,.T.);
#19748=EDGE_CURVE('',#15447,#15442,#3482,.T.);
#19749=EDGE_CURVE('',#15443,#15438,#3483,.T.);
#19750=EDGE_CURVE('',#15439,#15434,#3484,.T.);
#19751=EDGE_CURVE('',#15435,#15430,#3485,.T.);
#19752=EDGE_CURVE('',#15431,#15426,#3486,.T.);
#19753=EDGE_CURVE('',#15427,#15422,#3487,.T.);
#19754=EDGE_CURVE('',#15423,#15418,#3488,.T.);
#19755=EDGE_CURVE('',#15419,#15414,#3489,.T.);
#19756=EDGE_CURVE('',#15415,#15410,#3490,.T.);
#19757=EDGE_CURVE('',#15411,#15406,#3491,.T.);
#19758=EDGE_CURVE('',#15407,#15402,#3492,.T.);
#19759=EDGE_CURVE('',#15403,#15398,#3493,.T.);
#19760=EDGE_CURVE('',#15399,#15394,#3494,.T.);
#19761=EDGE_CURVE('',#15395,#15390,#3495,.T.);
#19762=EDGE_CURVE('',#15391,#15386,#3496,.T.);
#19763=EDGE_CURVE('',#15387,#15382,#3497,.T.);
#19764=EDGE_CURVE('',#15383,#15378,#3498,.T.);
#19765=EDGE_CURVE('',#15379,#15374,#3499,.T.);
#19766=EDGE_CURVE('',#15375,#15370,#3500,.T.);
#19767=EDGE_CURVE('',#15371,#15366,#3501,.T.);
#19768=EDGE_CURVE('',#15367,#15362,#3502,.T.);
#19769=EDGE_CURVE('',#15363,#15358,#3503,.T.);
#19770=EDGE_CURVE('',#15359,#15354,#3504,.T.);
#19771=EDGE_CURVE('',#15355,#15350,#3505,.T.);
#19772=EDGE_CURVE('',#15351,#15346,#3506,.T.);
#19773=EDGE_CURVE('',#15347,#15342,#3507,.T.);
#19774=EDGE_CURVE('',#15343,#15338,#3508,.T.);
#19775=EDGE_CURVE('',#15339,#15334,#3509,.T.);
#19776=EDGE_CURVE('',#15335,#15330,#3510,.T.);
#19777=EDGE_CURVE('',#15331,#15326,#3511,.T.);
#19778=EDGE_CURVE('',#15327,#15322,#3512,.T.);
#19779=EDGE_CURVE('',#15323,#15318,#3513,.T.);
#19780=EDGE_CURVE('',#15505,#15309,#10026,.T.);
#19781=EDGE_CURVE('',#15506,#15505,#3514,.T.);
#19782=EDGE_CURVE('',#15506,#15310,#10027,.T.);
#19783=EDGE_CURVE('',#15507,#15506,#3515,.T.);
#19784=EDGE_CURVE('',#15311,#15507,#10028,.T.);
#19785=EDGE_CURVE('',#15505,#15504,#3516,.T.);
#19786=EDGE_CURVE('',#15319,#15507,#3517,.T.);
#26578=ORIENTED_EDGE('',*,*,#19191,.T.);
#26579=ORIENTED_EDGE('',*,*,#19192,.T.);
#26580=ORIENTED_EDGE('',*,*,#19193,.T.);
#26581=ORIENTED_EDGE('',*,*,#19194,.T.);
#26582=ORIENTED_EDGE('',*,*,#19192,.F.);
#26583=ORIENTED_EDGE('',*,*,#19194,.F.);
#26584=ORIENTED_EDGE('',*,*,#19195,.T.);
#26585=ORIENTED_EDGE('',*,*,#19196,.F.);
#26586=ORIENTED_EDGE('',*,*,#19195,.F.);
#26587=ORIENTED_EDGE('',*,*,#19193,.F.);
#26588=ORIENTED_EDGE('',*,*,#19191,.F.);
#26589=ORIENTED_EDGE('',*,*,#19197,.T.);
#26590=ORIENTED_EDGE('',*,*,#19198,.T.);
#26591=ORIENTED_EDGE('',*,*,#19199,.T.);
#26592=ORIENTED_EDGE('',*,*,#19200,.T.);
#26593=ORIENTED_EDGE('',*,*,#19201,.T.);
#26594=ORIENTED_EDGE('',*,*,#19202,.T.);
#26595=ORIENTED_EDGE('',*,*,#19196,.T.);
#26596=ORIENTED_EDGE('',*,*,#19202,.F.);
#26597=ORIENTED_EDGE('',*,*,#19203,.T.);
#26598=ORIENTED_EDGE('',*,*,#19204,.T.);
#26599=ORIENTED_EDGE('',*,*,#19205,.T.);
#26600=ORIENTED_EDGE('',*,*,#19206,.F.);
#26601=ORIENTED_EDGE('',*,*,#19207,.T.);
#26602=ORIENTED_EDGE('',*,*,#19208,.T.);
#26603=ORIENTED_EDGE('',*,*,#19209,.T.);
#26604=ORIENTED_EDGE('',*,*,#19210,.F.);
#26605=ORIENTED_EDGE('',*,*,#19211,.T.);
#26606=ORIENTED_EDGE('',*,*,#19212,.T.);
#26607=ORIENTED_EDGE('',*,*,#19213,.T.);
#26608=ORIENTED_EDGE('',*,*,#19214,.F.);
#26609=ORIENTED_EDGE('',*,*,#19215,.T.);
#26610=ORIENTED_EDGE('',*,*,#19216,.T.);
#26611=ORIENTED_EDGE('',*,*,#19217,.T.);
#26612=ORIENTED_EDGE('',*,*,#19218,.F.);
#26613=ORIENTED_EDGE('',*,*,#19219,.T.);
#26614=ORIENTED_EDGE('',*,*,#19220,.T.);
#26615=ORIENTED_EDGE('',*,*,#19221,.T.);
#26616=ORIENTED_EDGE('',*,*,#19222,.F.);
#26617=ORIENTED_EDGE('',*,*,#19223,.T.);
#26618=ORIENTED_EDGE('',*,*,#19224,.T.);
#26619=ORIENTED_EDGE('',*,*,#19225,.T.);
#26620=ORIENTED_EDGE('',*,*,#19226,.F.);
#26621=ORIENTED_EDGE('',*,*,#19227,.T.);
#26622=ORIENTED_EDGE('',*,*,#19228,.T.);
#26623=ORIENTED_EDGE('',*,*,#19229,.T.);
#26624=ORIENTED_EDGE('',*,*,#19230,.F.);
#26625=ORIENTED_EDGE('',*,*,#19231,.T.);
#26626=ORIENTED_EDGE('',*,*,#19232,.T.);
#26627=ORIENTED_EDGE('',*,*,#19233,.T.);
#26628=ORIENTED_EDGE('',*,*,#19234,.F.);
#26629=ORIENTED_EDGE('',*,*,#19235,.T.);
#26630=ORIENTED_EDGE('',*,*,#19236,.T.);
#26631=ORIENTED_EDGE('',*,*,#19237,.T.);
#26632=ORIENTED_EDGE('',*,*,#19238,.F.);
#26633=ORIENTED_EDGE('',*,*,#19239,.T.);
#26634=ORIENTED_EDGE('',*,*,#19240,.T.);
#26635=ORIENTED_EDGE('',*,*,#19241,.T.);
#26636=ORIENTED_EDGE('',*,*,#19242,.F.);
#26637=ORIENTED_EDGE('',*,*,#19243,.T.);
#26638=ORIENTED_EDGE('',*,*,#19244,.T.);
#26639=ORIENTED_EDGE('',*,*,#19245,.T.);
#26640=ORIENTED_EDGE('',*,*,#19246,.F.);
#26641=ORIENTED_EDGE('',*,*,#19247,.T.);
#26642=ORIENTED_EDGE('',*,*,#19248,.T.);
#26643=ORIENTED_EDGE('',*,*,#19249,.T.);
#26644=ORIENTED_EDGE('',*,*,#19250,.F.);
#26645=ORIENTED_EDGE('',*,*,#19251,.T.);
#26646=ORIENTED_EDGE('',*,*,#19252,.T.);
#26647=ORIENTED_EDGE('',*,*,#19253,.T.);
#26648=ORIENTED_EDGE('',*,*,#19254,.F.);
#26649=ORIENTED_EDGE('',*,*,#19255,.T.);
#26650=ORIENTED_EDGE('',*,*,#19256,.T.);
#26651=ORIENTED_EDGE('',*,*,#19257,.T.);
#26652=ORIENTED_EDGE('',*,*,#19258,.F.);
#26653=ORIENTED_EDGE('',*,*,#19259,.T.);
#26654=ORIENTED_EDGE('',*,*,#19260,.T.);
#26655=ORIENTED_EDGE('',*,*,#19261,.T.);
#26656=ORIENTED_EDGE('',*,*,#19262,.F.);
#26657=ORIENTED_EDGE('',*,*,#19263,.T.);
#26658=ORIENTED_EDGE('',*,*,#19264,.T.);
#26659=ORIENTED_EDGE('',*,*,#19265,.T.);
#26660=ORIENTED_EDGE('',*,*,#19266,.F.);
#26661=ORIENTED_EDGE('',*,*,#19267,.T.);
#26662=ORIENTED_EDGE('',*,*,#19268,.T.);
#26663=ORIENTED_EDGE('',*,*,#19269,.T.);
#26664=ORIENTED_EDGE('',*,*,#19270,.F.);
#26665=ORIENTED_EDGE('',*,*,#19271,.T.);
#26666=ORIENTED_EDGE('',*,*,#19272,.T.);
#26667=ORIENTED_EDGE('',*,*,#19273,.T.);
#26668=ORIENTED_EDGE('',*,*,#19274,.F.);
#26669=ORIENTED_EDGE('',*,*,#19275,.T.);
#26670=ORIENTED_EDGE('',*,*,#19276,.T.);
#26671=ORIENTED_EDGE('',*,*,#19277,.T.);
#26672=ORIENTED_EDGE('',*,*,#19278,.F.);
#26673=ORIENTED_EDGE('',*,*,#19279,.T.);
#26674=ORIENTED_EDGE('',*,*,#19280,.T.);
#26675=ORIENTED_EDGE('',*,*,#19281,.T.);
#26676=ORIENTED_EDGE('',*,*,#19282,.F.);
#26677=ORIENTED_EDGE('',*,*,#19283,.T.);
#26678=ORIENTED_EDGE('',*,*,#19284,.T.);
#26679=ORIENTED_EDGE('',*,*,#19285,.T.);
#26680=ORIENTED_EDGE('',*,*,#19286,.F.);
#26681=ORIENTED_EDGE('',*,*,#19287,.T.);
#26682=ORIENTED_EDGE('',*,*,#19288,.T.);
#26683=ORIENTED_EDGE('',*,*,#19289,.T.);
#26684=ORIENTED_EDGE('',*,*,#19290,.F.);
#26685=ORIENTED_EDGE('',*,*,#19291,.T.);
#26686=ORIENTED_EDGE('',*,*,#19292,.T.);
#26687=ORIENTED_EDGE('',*,*,#19293,.T.);
#26688=ORIENTED_EDGE('',*,*,#19294,.F.);
#26689=ORIENTED_EDGE('',*,*,#19295,.T.);
#26690=ORIENTED_EDGE('',*,*,#19296,.T.);
#26691=ORIENTED_EDGE('',*,*,#19297,.T.);
#26692=ORIENTED_EDGE('',*,*,#19298,.F.);
#26693=ORIENTED_EDGE('',*,*,#19299,.T.);
#26694=ORIENTED_EDGE('',*,*,#19300,.T.);
#26695=ORIENTED_EDGE('',*,*,#19301,.T.);
#26696=ORIENTED_EDGE('',*,*,#19302,.F.);
#26697=ORIENTED_EDGE('',*,*,#19303,.T.);
#26698=ORIENTED_EDGE('',*,*,#19304,.T.);
#26699=ORIENTED_EDGE('',*,*,#19305,.T.);
#26700=ORIENTED_EDGE('',*,*,#19306,.F.);
#26701=ORIENTED_EDGE('',*,*,#19307,.T.);
#26702=ORIENTED_EDGE('',*,*,#19308,.T.);
#26703=ORIENTED_EDGE('',*,*,#19309,.T.);
#26704=ORIENTED_EDGE('',*,*,#19310,.F.);
#26705=ORIENTED_EDGE('',*,*,#19311,.T.);
#26706=ORIENTED_EDGE('',*,*,#19312,.T.);
#26707=ORIENTED_EDGE('',*,*,#19313,.T.);
#26708=ORIENTED_EDGE('',*,*,#19314,.F.);
#26709=ORIENTED_EDGE('',*,*,#19315,.T.);
#26710=ORIENTED_EDGE('',*,*,#19316,.T.);
#26711=ORIENTED_EDGE('',*,*,#19317,.T.);
#26712=ORIENTED_EDGE('',*,*,#19318,.F.);
#26713=ORIENTED_EDGE('',*,*,#19319,.T.);
#26714=ORIENTED_EDGE('',*,*,#19320,.T.);
#26715=ORIENTED_EDGE('',*,*,#19321,.T.);
#26716=ORIENTED_EDGE('',*,*,#19322,.F.);
#26717=ORIENTED_EDGE('',*,*,#19323,.T.);
#26718=ORIENTED_EDGE('',*,*,#19324,.T.);
#26719=ORIENTED_EDGE('',*,*,#19325,.T.);
#26720=ORIENTED_EDGE('',*,*,#19326,.F.);
#26721=ORIENTED_EDGE('',*,*,#19327,.T.);
#26722=ORIENTED_EDGE('',*,*,#19328,.T.);
#26723=ORIENTED_EDGE('',*,*,#19329,.T.);
#26724=ORIENTED_EDGE('',*,*,#19330,.F.);
#26725=ORIENTED_EDGE('',*,*,#19331,.T.);
#26726=ORIENTED_EDGE('',*,*,#19332,.T.);
#26727=ORIENTED_EDGE('',*,*,#19333,.T.);
#26728=ORIENTED_EDGE('',*,*,#19334,.F.);
#26729=ORIENTED_EDGE('',*,*,#19335,.T.);
#26730=ORIENTED_EDGE('',*,*,#19336,.T.);
#26731=ORIENTED_EDGE('',*,*,#19337,.T.);
#26732=ORIENTED_EDGE('',*,*,#19338,.F.);
#26733=ORIENTED_EDGE('',*,*,#19339,.T.);
#26734=ORIENTED_EDGE('',*,*,#19340,.T.);
#26735=ORIENTED_EDGE('',*,*,#19341,.T.);
#26736=ORIENTED_EDGE('',*,*,#19342,.F.);
#26737=ORIENTED_EDGE('',*,*,#19343,.T.);
#26738=ORIENTED_EDGE('',*,*,#19344,.T.);
#26739=ORIENTED_EDGE('',*,*,#19345,.T.);
#26740=ORIENTED_EDGE('',*,*,#19346,.F.);
#26741=ORIENTED_EDGE('',*,*,#19347,.T.);
#26742=ORIENTED_EDGE('',*,*,#19348,.T.);
#26743=ORIENTED_EDGE('',*,*,#19349,.T.);
#26744=ORIENTED_EDGE('',*,*,#19350,.F.);
#26745=ORIENTED_EDGE('',*,*,#19351,.T.);
#26746=ORIENTED_EDGE('',*,*,#19352,.T.);
#26747=ORIENTED_EDGE('',*,*,#19353,.T.);
#26748=ORIENTED_EDGE('',*,*,#19354,.F.);
#26749=ORIENTED_EDGE('',*,*,#19355,.T.);
#26750=ORIENTED_EDGE('',*,*,#19356,.T.);
#26751=ORIENTED_EDGE('',*,*,#19357,.T.);
#26752=ORIENTED_EDGE('',*,*,#19358,.F.);
#26753=ORIENTED_EDGE('',*,*,#19359,.T.);
#26754=ORIENTED_EDGE('',*,*,#19360,.T.);
#26755=ORIENTED_EDGE('',*,*,#19361,.T.);
#26756=ORIENTED_EDGE('',*,*,#19362,.F.);
#26757=ORIENTED_EDGE('',*,*,#19363,.T.);
#26758=ORIENTED_EDGE('',*,*,#19364,.T.);
#26759=ORIENTED_EDGE('',*,*,#19365,.T.);
#26760=ORIENTED_EDGE('',*,*,#19366,.F.);
#26761=ORIENTED_EDGE('',*,*,#19367,.T.);
#26762=ORIENTED_EDGE('',*,*,#19368,.T.);
#26763=ORIENTED_EDGE('',*,*,#19369,.T.);
#26764=ORIENTED_EDGE('',*,*,#19370,.F.);
#26765=ORIENTED_EDGE('',*,*,#19371,.T.);
#26766=ORIENTED_EDGE('',*,*,#19372,.T.);
#26767=ORIENTED_EDGE('',*,*,#19373,.T.);
#26768=ORIENTED_EDGE('',*,*,#19374,.F.);
#26769=ORIENTED_EDGE('',*,*,#19375,.T.);
#26770=ORIENTED_EDGE('',*,*,#19376,.T.);
#26771=ORIENTED_EDGE('',*,*,#19377,.T.);
#26772=ORIENTED_EDGE('',*,*,#19378,.F.);
#26773=ORIENTED_EDGE('',*,*,#19379,.T.);
#26774=ORIENTED_EDGE('',*,*,#19380,.T.);
#26775=ORIENTED_EDGE('',*,*,#19381,.T.);
#26776=ORIENTED_EDGE('',*,*,#19382,.F.);
#26777=ORIENTED_EDGE('',*,*,#19383,.T.);
#26778=ORIENTED_EDGE('',*,*,#19384,.T.);
#26779=ORIENTED_EDGE('',*,*,#19385,.T.);
#26780=ORIENTED_EDGE('',*,*,#19386,.F.);
#26781=ORIENTED_EDGE('',*,*,#19387,.T.);
#26782=ORIENTED_EDGE('',*,*,#19388,.T.);
#26783=ORIENTED_EDGE('',*,*,#19389,.T.);
#26784=ORIENTED_EDGE('',*,*,#19390,.F.);
#26785=ORIENTED_EDGE('',*,*,#19391,.T.);
#26786=ORIENTED_EDGE('',*,*,#19392,.T.);
#26787=ORIENTED_EDGE('',*,*,#19393,.T.);
#26788=ORIENTED_EDGE('',*,*,#19394,.F.);
#26789=ORIENTED_EDGE('',*,*,#19201,.F.);
#26790=ORIENTED_EDGE('',*,*,#19395,.F.);
#26791=ORIENTED_EDGE('',*,*,#19396,.F.);
#26792=ORIENTED_EDGE('',*,*,#19198,.F.);
#26793=ORIENTED_EDGE('',*,*,#19397,.T.);
#26794=ORIENTED_EDGE('',*,*,#19398,.F.);
#26795=ORIENTED_EDGE('',*,*,#19397,.F.);
#26796=ORIENTED_EDGE('',*,*,#19197,.F.);
#26797=ORIENTED_EDGE('',*,*,#19399,.F.);
#26798=ORIENTED_EDGE('',*,*,#19400,.F.);
#26799=ORIENTED_EDGE('',*,*,#19399,.T.);
#26800=ORIENTED_EDGE('',*,*,#19200,.F.);
#26801=ORIENTED_EDGE('',*,*,#19401,.T.);
#26802=ORIENTED_EDGE('',*,*,#19402,.F.);
#26803=ORIENTED_EDGE('',*,*,#19401,.F.);
#26804=ORIENTED_EDGE('',*,*,#19199,.F.);
#26805=ORIENTED_EDGE('',*,*,#19396,.T.);
#26806=ORIENTED_EDGE('',*,*,#19204,.F.);
#26807=ORIENTED_EDGE('',*,*,#19403,.F.);
#26808=ORIENTED_EDGE('',*,*,#19404,.F.);
#26809=ORIENTED_EDGE('',*,*,#19405,.T.);
#26810=ORIENTED_EDGE('',*,*,#19205,.F.);
#26811=ORIENTED_EDGE('',*,*,#19405,.F.);
#26812=ORIENTED_EDGE('',*,*,#19406,.F.);
#26813=ORIENTED_EDGE('',*,*,#19407,.F.);
#26814=ORIENTED_EDGE('',*,*,#19203,.F.);
#26815=ORIENTED_EDGE('',*,*,#19408,.F.);
#26816=ORIENTED_EDGE('',*,*,#19409,.F.);
#26817=ORIENTED_EDGE('',*,*,#19403,.T.);
#26818=ORIENTED_EDGE('',*,*,#19208,.F.);
#26819=ORIENTED_EDGE('',*,*,#19410,.F.);
#26820=ORIENTED_EDGE('',*,*,#19411,.F.);
#26821=ORIENTED_EDGE('',*,*,#19412,.T.);
#26822=ORIENTED_EDGE('',*,*,#19209,.F.);
#26823=ORIENTED_EDGE('',*,*,#19412,.F.);
#26824=ORIENTED_EDGE('',*,*,#19413,.F.);
#26825=ORIENTED_EDGE('',*,*,#19414,.F.);
#26826=ORIENTED_EDGE('',*,*,#19207,.F.);
#26827=ORIENTED_EDGE('',*,*,#19415,.F.);
#26828=ORIENTED_EDGE('',*,*,#19416,.F.);
#26829=ORIENTED_EDGE('',*,*,#19410,.T.);
#26830=ORIENTED_EDGE('',*,*,#19212,.F.);
#26831=ORIENTED_EDGE('',*,*,#19417,.F.);
#26832=ORIENTED_EDGE('',*,*,#19418,.F.);
#26833=ORIENTED_EDGE('',*,*,#19419,.T.);
#26834=ORIENTED_EDGE('',*,*,#19213,.F.);
#26835=ORIENTED_EDGE('',*,*,#19419,.F.);
#26836=ORIENTED_EDGE('',*,*,#19420,.F.);
#26837=ORIENTED_EDGE('',*,*,#19421,.F.);
#26838=ORIENTED_EDGE('',*,*,#19211,.F.);
#26839=ORIENTED_EDGE('',*,*,#19422,.F.);
#26840=ORIENTED_EDGE('',*,*,#19423,.F.);
#26841=ORIENTED_EDGE('',*,*,#19417,.T.);
#26842=ORIENTED_EDGE('',*,*,#19216,.F.);
#26843=ORIENTED_EDGE('',*,*,#19424,.F.);
#26844=ORIENTED_EDGE('',*,*,#19425,.F.);
#26845=ORIENTED_EDGE('',*,*,#19426,.T.);
#26846=ORIENTED_EDGE('',*,*,#19217,.F.);
#26847=ORIENTED_EDGE('',*,*,#19426,.F.);
#26848=ORIENTED_EDGE('',*,*,#19427,.F.);
#26849=ORIENTED_EDGE('',*,*,#19428,.F.);
#26850=ORIENTED_EDGE('',*,*,#19215,.F.);
#26851=ORIENTED_EDGE('',*,*,#19429,.F.);
#26852=ORIENTED_EDGE('',*,*,#19430,.F.);
#26853=ORIENTED_EDGE('',*,*,#19424,.T.);
#26854=ORIENTED_EDGE('',*,*,#19220,.F.);
#26855=ORIENTED_EDGE('',*,*,#19431,.F.);
#26856=ORIENTED_EDGE('',*,*,#19432,.F.);
#26857=ORIENTED_EDGE('',*,*,#19433,.T.);
#26858=ORIENTED_EDGE('',*,*,#19221,.F.);
#26859=ORIENTED_EDGE('',*,*,#19433,.F.);
#26860=ORIENTED_EDGE('',*,*,#19434,.F.);
#26861=ORIENTED_EDGE('',*,*,#19435,.F.);
#26862=ORIENTED_EDGE('',*,*,#19219,.F.);
#26863=ORIENTED_EDGE('',*,*,#19436,.F.);
#26864=ORIENTED_EDGE('',*,*,#19437,.F.);
#26865=ORIENTED_EDGE('',*,*,#19431,.T.);
#26866=ORIENTED_EDGE('',*,*,#19224,.F.);
#26867=ORIENTED_EDGE('',*,*,#19438,.F.);
#26868=ORIENTED_EDGE('',*,*,#19439,.F.);
#26869=ORIENTED_EDGE('',*,*,#19440,.T.);
#26870=ORIENTED_EDGE('',*,*,#19225,.F.);
#26871=ORIENTED_EDGE('',*,*,#19440,.F.);
#26872=ORIENTED_EDGE('',*,*,#19441,.F.);
#26873=ORIENTED_EDGE('',*,*,#19442,.F.);
#26874=ORIENTED_EDGE('',*,*,#19223,.F.);
#26875=ORIENTED_EDGE('',*,*,#19443,.F.);
#26876=ORIENTED_EDGE('',*,*,#19444,.F.);
#26877=ORIENTED_EDGE('',*,*,#19438,.T.);
#26878=ORIENTED_EDGE('',*,*,#19228,.F.);
#26879=ORIENTED_EDGE('',*,*,#19445,.F.);
#26880=ORIENTED_EDGE('',*,*,#19446,.F.);
#26881=ORIENTED_EDGE('',*,*,#19447,.T.);
#26882=ORIENTED_EDGE('',*,*,#19229,.F.);
#26883=ORIENTED_EDGE('',*,*,#19447,.F.);
#26884=ORIENTED_EDGE('',*,*,#19448,.F.);
#26885=ORIENTED_EDGE('',*,*,#19449,.F.);
#26886=ORIENTED_EDGE('',*,*,#19227,.F.);
#26887=ORIENTED_EDGE('',*,*,#19450,.F.);
#26888=ORIENTED_EDGE('',*,*,#19451,.F.);
#26889=ORIENTED_EDGE('',*,*,#19445,.T.);
#26890=ORIENTED_EDGE('',*,*,#19232,.F.);
#26891=ORIENTED_EDGE('',*,*,#19452,.F.);
#26892=ORIENTED_EDGE('',*,*,#19453,.F.);
#26893=ORIENTED_EDGE('',*,*,#19454,.T.);
#26894=ORIENTED_EDGE('',*,*,#19233,.F.);
#26895=ORIENTED_EDGE('',*,*,#19454,.F.);
#26896=ORIENTED_EDGE('',*,*,#19455,.F.);
#26897=ORIENTED_EDGE('',*,*,#19456,.F.);
#26898=ORIENTED_EDGE('',*,*,#19231,.F.);
#26899=ORIENTED_EDGE('',*,*,#19457,.F.);
#26900=ORIENTED_EDGE('',*,*,#19458,.F.);
#26901=ORIENTED_EDGE('',*,*,#19452,.T.);
#26902=ORIENTED_EDGE('',*,*,#19236,.F.);
#26903=ORIENTED_EDGE('',*,*,#19459,.F.);
#26904=ORIENTED_EDGE('',*,*,#19460,.F.);
#26905=ORIENTED_EDGE('',*,*,#19461,.T.);
#26906=ORIENTED_EDGE('',*,*,#19237,.F.);
#26907=ORIENTED_EDGE('',*,*,#19461,.F.);
#26908=ORIENTED_EDGE('',*,*,#19462,.F.);
#26909=ORIENTED_EDGE('',*,*,#19463,.F.);
#26910=ORIENTED_EDGE('',*,*,#19235,.F.);
#26911=ORIENTED_EDGE('',*,*,#19464,.F.);
#26912=ORIENTED_EDGE('',*,*,#19465,.F.);
#26913=ORIENTED_EDGE('',*,*,#19459,.T.);
#26914=ORIENTED_EDGE('',*,*,#19240,.F.);
#26915=ORIENTED_EDGE('',*,*,#19466,.F.);
#26916=ORIENTED_EDGE('',*,*,#19467,.F.);
#26917=ORIENTED_EDGE('',*,*,#19468,.T.);
#26918=ORIENTED_EDGE('',*,*,#19241,.F.);
#26919=ORIENTED_EDGE('',*,*,#19468,.F.);
#26920=ORIENTED_EDGE('',*,*,#19469,.F.);
#26921=ORIENTED_EDGE('',*,*,#19470,.F.);
#26922=ORIENTED_EDGE('',*,*,#19239,.F.);
#26923=ORIENTED_EDGE('',*,*,#19471,.F.);
#26924=ORIENTED_EDGE('',*,*,#19472,.F.);
#26925=ORIENTED_EDGE('',*,*,#19466,.T.);
#26926=ORIENTED_EDGE('',*,*,#19244,.F.);
#26927=ORIENTED_EDGE('',*,*,#19473,.F.);
#26928=ORIENTED_EDGE('',*,*,#19474,.F.);
#26929=ORIENTED_EDGE('',*,*,#19475,.T.);
#26930=ORIENTED_EDGE('',*,*,#19245,.F.);
#26931=ORIENTED_EDGE('',*,*,#19475,.F.);
#26932=ORIENTED_EDGE('',*,*,#19476,.F.);
#26933=ORIENTED_EDGE('',*,*,#19477,.F.);
#26934=ORIENTED_EDGE('',*,*,#19243,.F.);
#26935=ORIENTED_EDGE('',*,*,#19478,.F.);
#26936=ORIENTED_EDGE('',*,*,#19479,.F.);
#26937=ORIENTED_EDGE('',*,*,#19473,.T.);
#26938=ORIENTED_EDGE('',*,*,#19248,.F.);
#26939=ORIENTED_EDGE('',*,*,#19480,.F.);
#26940=ORIENTED_EDGE('',*,*,#19481,.F.);
#26941=ORIENTED_EDGE('',*,*,#19482,.T.);
#26942=ORIENTED_EDGE('',*,*,#19249,.F.);
#26943=ORIENTED_EDGE('',*,*,#19482,.F.);
#26944=ORIENTED_EDGE('',*,*,#19483,.F.);
#26945=ORIENTED_EDGE('',*,*,#19484,.F.);
#26946=ORIENTED_EDGE('',*,*,#19247,.F.);
#26947=ORIENTED_EDGE('',*,*,#19485,.F.);
#26948=ORIENTED_EDGE('',*,*,#19486,.F.);
#26949=ORIENTED_EDGE('',*,*,#19480,.T.);
#26950=ORIENTED_EDGE('',*,*,#19252,.F.);
#26951=ORIENTED_EDGE('',*,*,#19487,.F.);
#26952=ORIENTED_EDGE('',*,*,#19488,.F.);
#26953=ORIENTED_EDGE('',*,*,#19489,.T.);
#26954=ORIENTED_EDGE('',*,*,#19253,.F.);
#26955=ORIENTED_EDGE('',*,*,#19489,.F.);
#26956=ORIENTED_EDGE('',*,*,#19490,.F.);
#26957=ORIENTED_EDGE('',*,*,#19491,.F.);
#26958=ORIENTED_EDGE('',*,*,#19251,.F.);
#26959=ORIENTED_EDGE('',*,*,#19492,.F.);
#26960=ORIENTED_EDGE('',*,*,#19493,.F.);
#26961=ORIENTED_EDGE('',*,*,#19487,.T.);
#26962=ORIENTED_EDGE('',*,*,#19256,.F.);
#26963=ORIENTED_EDGE('',*,*,#19494,.F.);
#26964=ORIENTED_EDGE('',*,*,#19495,.F.);
#26965=ORIENTED_EDGE('',*,*,#19496,.T.);
#26966=ORIENTED_EDGE('',*,*,#19257,.F.);
#26967=ORIENTED_EDGE('',*,*,#19496,.F.);
#26968=ORIENTED_EDGE('',*,*,#19497,.F.);
#26969=ORIENTED_EDGE('',*,*,#19498,.F.);
#26970=ORIENTED_EDGE('',*,*,#19255,.F.);
#26971=ORIENTED_EDGE('',*,*,#19499,.F.);
#26972=ORIENTED_EDGE('',*,*,#19500,.F.);
#26973=ORIENTED_EDGE('',*,*,#19494,.T.);
#26974=ORIENTED_EDGE('',*,*,#19260,.F.);
#26975=ORIENTED_EDGE('',*,*,#19501,.F.);
#26976=ORIENTED_EDGE('',*,*,#19502,.F.);
#26977=ORIENTED_EDGE('',*,*,#19503,.T.);
#26978=ORIENTED_EDGE('',*,*,#19261,.F.);
#26979=ORIENTED_EDGE('',*,*,#19503,.F.);
#26980=ORIENTED_EDGE('',*,*,#19504,.F.);
#26981=ORIENTED_EDGE('',*,*,#19505,.F.);
#26982=ORIENTED_EDGE('',*,*,#19259,.F.);
#26983=ORIENTED_EDGE('',*,*,#19506,.F.);
#26984=ORIENTED_EDGE('',*,*,#19507,.F.);
#26985=ORIENTED_EDGE('',*,*,#19501,.T.);
#26986=ORIENTED_EDGE('',*,*,#19264,.F.);
#26987=ORIENTED_EDGE('',*,*,#19508,.F.);
#26988=ORIENTED_EDGE('',*,*,#19509,.F.);
#26989=ORIENTED_EDGE('',*,*,#19510,.T.);
#26990=ORIENTED_EDGE('',*,*,#19265,.F.);
#26991=ORIENTED_EDGE('',*,*,#19510,.F.);
#26992=ORIENTED_EDGE('',*,*,#19511,.F.);
#26993=ORIENTED_EDGE('',*,*,#19512,.F.);
#26994=ORIENTED_EDGE('',*,*,#19263,.F.);
#26995=ORIENTED_EDGE('',*,*,#19513,.F.);
#26996=ORIENTED_EDGE('',*,*,#19514,.F.);
#26997=ORIENTED_EDGE('',*,*,#19508,.T.);
#26998=ORIENTED_EDGE('',*,*,#19268,.F.);
#26999=ORIENTED_EDGE('',*,*,#19515,.F.);
#27000=ORIENTED_EDGE('',*,*,#19516,.F.);
#27001=ORIENTED_EDGE('',*,*,#19517,.T.);
#27002=ORIENTED_EDGE('',*,*,#19269,.F.);
#27003=ORIENTED_EDGE('',*,*,#19517,.F.);
#27004=ORIENTED_EDGE('',*,*,#19518,.F.);
#27005=ORIENTED_EDGE('',*,*,#19519,.F.);
#27006=ORIENTED_EDGE('',*,*,#19267,.F.);
#27007=ORIENTED_EDGE('',*,*,#19520,.F.);
#27008=ORIENTED_EDGE('',*,*,#19521,.F.);
#27009=ORIENTED_EDGE('',*,*,#19515,.T.);
#27010=ORIENTED_EDGE('',*,*,#19272,.F.);
#27011=ORIENTED_EDGE('',*,*,#19522,.F.);
#27012=ORIENTED_EDGE('',*,*,#19523,.F.);
#27013=ORIENTED_EDGE('',*,*,#19524,.T.);
#27014=ORIENTED_EDGE('',*,*,#19273,.F.);
#27015=ORIENTED_EDGE('',*,*,#19524,.F.);
#27016=ORIENTED_EDGE('',*,*,#19525,.F.);
#27017=ORIENTED_EDGE('',*,*,#19526,.F.);
#27018=ORIENTED_EDGE('',*,*,#19271,.F.);
#27019=ORIENTED_EDGE('',*,*,#19527,.F.);
#27020=ORIENTED_EDGE('',*,*,#19528,.F.);
#27021=ORIENTED_EDGE('',*,*,#19522,.T.);
#27022=ORIENTED_EDGE('',*,*,#19276,.F.);
#27023=ORIENTED_EDGE('',*,*,#19529,.F.);
#27024=ORIENTED_EDGE('',*,*,#19530,.F.);
#27025=ORIENTED_EDGE('',*,*,#19531,.T.);
#27026=ORIENTED_EDGE('',*,*,#19277,.F.);
#27027=ORIENTED_EDGE('',*,*,#19531,.F.);
#27028=ORIENTED_EDGE('',*,*,#19532,.F.);
#27029=ORIENTED_EDGE('',*,*,#19533,.F.);
#27030=ORIENTED_EDGE('',*,*,#19275,.F.);
#27031=ORIENTED_EDGE('',*,*,#19534,.F.);
#27032=ORIENTED_EDGE('',*,*,#19535,.F.);
#27033=ORIENTED_EDGE('',*,*,#19529,.T.);
#27034=ORIENTED_EDGE('',*,*,#19280,.F.);
#27035=ORIENTED_EDGE('',*,*,#19536,.F.);
#27036=ORIENTED_EDGE('',*,*,#19537,.F.);
#27037=ORIENTED_EDGE('',*,*,#19538,.T.);
#27038=ORIENTED_EDGE('',*,*,#19281,.F.);
#27039=ORIENTED_EDGE('',*,*,#19538,.F.);
#27040=ORIENTED_EDGE('',*,*,#19539,.F.);
#27041=ORIENTED_EDGE('',*,*,#19540,.F.);
#27042=ORIENTED_EDGE('',*,*,#19279,.F.);
#27043=ORIENTED_EDGE('',*,*,#19541,.F.);
#27044=ORIENTED_EDGE('',*,*,#19542,.F.);
#27045=ORIENTED_EDGE('',*,*,#19536,.T.);
#27046=ORIENTED_EDGE('',*,*,#19284,.F.);
#27047=ORIENTED_EDGE('',*,*,#19543,.F.);
#27048=ORIENTED_EDGE('',*,*,#19544,.F.);
#27049=ORIENTED_EDGE('',*,*,#19545,.T.);
#27050=ORIENTED_EDGE('',*,*,#19285,.F.);
#27051=ORIENTED_EDGE('',*,*,#19545,.F.);
#27052=ORIENTED_EDGE('',*,*,#19546,.F.);
#27053=ORIENTED_EDGE('',*,*,#19547,.F.);
#27054=ORIENTED_EDGE('',*,*,#19283,.F.);
#27055=ORIENTED_EDGE('',*,*,#19548,.F.);
#27056=ORIENTED_EDGE('',*,*,#19549,.F.);
#27057=ORIENTED_EDGE('',*,*,#19543,.T.);
#27058=ORIENTED_EDGE('',*,*,#19288,.F.);
#27059=ORIENTED_EDGE('',*,*,#19550,.F.);
#27060=ORIENTED_EDGE('',*,*,#19551,.F.);
#27061=ORIENTED_EDGE('',*,*,#19552,.T.);
#27062=ORIENTED_EDGE('',*,*,#19289,.F.);
#27063=ORIENTED_EDGE('',*,*,#19552,.F.);
#27064=ORIENTED_EDGE('',*,*,#19553,.F.);
#27065=ORIENTED_EDGE('',*,*,#19554,.F.);
#27066=ORIENTED_EDGE('',*,*,#19287,.F.);
#27067=ORIENTED_EDGE('',*,*,#19555,.F.);
#27068=ORIENTED_EDGE('',*,*,#19556,.F.);
#27069=ORIENTED_EDGE('',*,*,#19550,.T.);
#27070=ORIENTED_EDGE('',*,*,#19292,.F.);
#27071=ORIENTED_EDGE('',*,*,#19557,.F.);
#27072=ORIENTED_EDGE('',*,*,#19558,.F.);
#27073=ORIENTED_EDGE('',*,*,#19559,.T.);
#27074=ORIENTED_EDGE('',*,*,#19293,.F.);
#27075=ORIENTED_EDGE('',*,*,#19559,.F.);
#27076=ORIENTED_EDGE('',*,*,#19560,.F.);
#27077=ORIENTED_EDGE('',*,*,#19561,.F.);
#27078=ORIENTED_EDGE('',*,*,#19291,.F.);
#27079=ORIENTED_EDGE('',*,*,#19562,.F.);
#27080=ORIENTED_EDGE('',*,*,#19563,.F.);
#27081=ORIENTED_EDGE('',*,*,#19557,.T.);
#27082=ORIENTED_EDGE('',*,*,#19296,.F.);
#27083=ORIENTED_EDGE('',*,*,#19564,.F.);
#27084=ORIENTED_EDGE('',*,*,#19565,.F.);
#27085=ORIENTED_EDGE('',*,*,#19566,.T.);
#27086=ORIENTED_EDGE('',*,*,#19297,.F.);
#27087=ORIENTED_EDGE('',*,*,#19566,.F.);
#27088=ORIENTED_EDGE('',*,*,#19567,.F.);
#27089=ORIENTED_EDGE('',*,*,#19568,.F.);
#27090=ORIENTED_EDGE('',*,*,#19295,.F.);
#27091=ORIENTED_EDGE('',*,*,#19569,.F.);
#27092=ORIENTED_EDGE('',*,*,#19570,.F.);
#27093=ORIENTED_EDGE('',*,*,#19564,.T.);
#27094=ORIENTED_EDGE('',*,*,#19300,.F.);
#27095=ORIENTED_EDGE('',*,*,#19571,.F.);
#27096=ORIENTED_EDGE('',*,*,#19572,.F.);
#27097=ORIENTED_EDGE('',*,*,#19573,.T.);
#27098=ORIENTED_EDGE('',*,*,#19301,.F.);
#27099=ORIENTED_EDGE('',*,*,#19573,.F.);
#27100=ORIENTED_EDGE('',*,*,#19574,.F.);
#27101=ORIENTED_EDGE('',*,*,#19575,.F.);
#27102=ORIENTED_EDGE('',*,*,#19299,.F.);
#27103=ORIENTED_EDGE('',*,*,#19576,.F.);
#27104=ORIENTED_EDGE('',*,*,#19577,.F.);
#27105=ORIENTED_EDGE('',*,*,#19571,.T.);
#27106=ORIENTED_EDGE('',*,*,#19304,.F.);
#27107=ORIENTED_EDGE('',*,*,#19578,.F.);
#27108=ORIENTED_EDGE('',*,*,#19579,.F.);
#27109=ORIENTED_EDGE('',*,*,#19580,.T.);
#27110=ORIENTED_EDGE('',*,*,#19305,.F.);
#27111=ORIENTED_EDGE('',*,*,#19580,.F.);
#27112=ORIENTED_EDGE('',*,*,#19581,.F.);
#27113=ORIENTED_EDGE('',*,*,#19582,.F.);
#27114=ORIENTED_EDGE('',*,*,#19303,.F.);
#27115=ORIENTED_EDGE('',*,*,#19583,.F.);
#27116=ORIENTED_EDGE('',*,*,#19584,.F.);
#27117=ORIENTED_EDGE('',*,*,#19578,.T.);
#27118=ORIENTED_EDGE('',*,*,#19308,.F.);
#27119=ORIENTED_EDGE('',*,*,#19585,.F.);
#27120=ORIENTED_EDGE('',*,*,#19586,.F.);
#27121=ORIENTED_EDGE('',*,*,#19587,.T.);
#27122=ORIENTED_EDGE('',*,*,#19309,.F.);
#27123=ORIENTED_EDGE('',*,*,#19587,.F.);
#27124=ORIENTED_EDGE('',*,*,#19588,.F.);
#27125=ORIENTED_EDGE('',*,*,#19589,.F.);
#27126=ORIENTED_EDGE('',*,*,#19307,.F.);
#27127=ORIENTED_EDGE('',*,*,#19590,.F.);
#27128=ORIENTED_EDGE('',*,*,#19591,.F.);
#27129=ORIENTED_EDGE('',*,*,#19585,.T.);
#27130=ORIENTED_EDGE('',*,*,#19312,.F.);
#27131=ORIENTED_EDGE('',*,*,#19592,.F.);
#27132=ORIENTED_EDGE('',*,*,#19593,.F.);
#27133=ORIENTED_EDGE('',*,*,#19594,.T.);
#27134=ORIENTED_EDGE('',*,*,#19313,.F.);
#27135=ORIENTED_EDGE('',*,*,#19594,.F.);
#27136=ORIENTED_EDGE('',*,*,#19595,.F.);
#27137=ORIENTED_EDGE('',*,*,#19596,.F.);
#27138=ORIENTED_EDGE('',*,*,#19311,.F.);
#27139=ORIENTED_EDGE('',*,*,#19597,.F.);
#27140=ORIENTED_EDGE('',*,*,#19598,.F.);
#27141=ORIENTED_EDGE('',*,*,#19592,.T.);
#27142=ORIENTED_EDGE('',*,*,#19316,.F.);
#27143=ORIENTED_EDGE('',*,*,#19599,.F.);
#27144=ORIENTED_EDGE('',*,*,#19600,.F.);
#27145=ORIENTED_EDGE('',*,*,#19601,.T.);
#27146=ORIENTED_EDGE('',*,*,#19317,.F.);
#27147=ORIENTED_EDGE('',*,*,#19601,.F.);
#27148=ORIENTED_EDGE('',*,*,#19602,.F.);
#27149=ORIENTED_EDGE('',*,*,#19603,.F.);
#27150=ORIENTED_EDGE('',*,*,#19315,.F.);
#27151=ORIENTED_EDGE('',*,*,#19604,.F.);
#27152=ORIENTED_EDGE('',*,*,#19605,.F.);
#27153=ORIENTED_EDGE('',*,*,#19599,.T.);
#27154=ORIENTED_EDGE('',*,*,#19320,.F.);
#27155=ORIENTED_EDGE('',*,*,#19606,.F.);
#27156=ORIENTED_EDGE('',*,*,#19607,.F.);
#27157=ORIENTED_EDGE('',*,*,#19608,.T.);
#27158=ORIENTED_EDGE('',*,*,#19321,.F.);
#27159=ORIENTED_EDGE('',*,*,#19608,.F.);
#27160=ORIENTED_EDGE('',*,*,#19609,.F.);
#27161=ORIENTED_EDGE('',*,*,#19610,.F.);
#27162=ORIENTED_EDGE('',*,*,#19319,.F.);
#27163=ORIENTED_EDGE('',*,*,#19611,.F.);
#27164=ORIENTED_EDGE('',*,*,#19612,.F.);
#27165=ORIENTED_EDGE('',*,*,#19606,.T.);
#27166=ORIENTED_EDGE('',*,*,#19324,.F.);
#27167=ORIENTED_EDGE('',*,*,#19613,.F.);
#27168=ORIENTED_EDGE('',*,*,#19614,.F.);
#27169=ORIENTED_EDGE('',*,*,#19615,.T.);
#27170=ORIENTED_EDGE('',*,*,#19325,.F.);
#27171=ORIENTED_EDGE('',*,*,#19615,.F.);
#27172=ORIENTED_EDGE('',*,*,#19616,.F.);
#27173=ORIENTED_EDGE('',*,*,#19617,.F.);
#27174=ORIENTED_EDGE('',*,*,#19323,.F.);
#27175=ORIENTED_EDGE('',*,*,#19618,.F.);
#27176=ORIENTED_EDGE('',*,*,#19619,.F.);
#27177=ORIENTED_EDGE('',*,*,#19613,.T.);
#27178=ORIENTED_EDGE('',*,*,#19328,.F.);
#27179=ORIENTED_EDGE('',*,*,#19620,.F.);
#27180=ORIENTED_EDGE('',*,*,#19621,.F.);
#27181=ORIENTED_EDGE('',*,*,#19622,.T.);
#27182=ORIENTED_EDGE('',*,*,#19329,.F.);
#27183=ORIENTED_EDGE('',*,*,#19622,.F.);
#27184=ORIENTED_EDGE('',*,*,#19623,.F.);
#27185=ORIENTED_EDGE('',*,*,#19624,.F.);
#27186=ORIENTED_EDGE('',*,*,#19327,.F.);
#27187=ORIENTED_EDGE('',*,*,#19625,.F.);
#27188=ORIENTED_EDGE('',*,*,#19626,.F.);
#27189=ORIENTED_EDGE('',*,*,#19620,.T.);
#27190=ORIENTED_EDGE('',*,*,#19332,.F.);
#27191=ORIENTED_EDGE('',*,*,#19627,.F.);
#27192=ORIENTED_EDGE('',*,*,#19628,.F.);
#27193=ORIENTED_EDGE('',*,*,#19629,.T.);
#27194=ORIENTED_EDGE('',*,*,#19333,.F.);
#27195=ORIENTED_EDGE('',*,*,#19629,.F.);
#27196=ORIENTED_EDGE('',*,*,#19630,.F.);
#27197=ORIENTED_EDGE('',*,*,#19631,.F.);
#27198=ORIENTED_EDGE('',*,*,#19331,.F.);
#27199=ORIENTED_EDGE('',*,*,#19632,.F.);
#27200=ORIENTED_EDGE('',*,*,#19633,.F.);
#27201=ORIENTED_EDGE('',*,*,#19627,.T.);
#27202=ORIENTED_EDGE('',*,*,#19336,.F.);
#27203=ORIENTED_EDGE('',*,*,#19634,.F.);
#27204=ORIENTED_EDGE('',*,*,#19635,.F.);
#27205=ORIENTED_EDGE('',*,*,#19636,.T.);
#27206=ORIENTED_EDGE('',*,*,#19337,.F.);
#27207=ORIENTED_EDGE('',*,*,#19636,.F.);
#27208=ORIENTED_EDGE('',*,*,#19637,.F.);
#27209=ORIENTED_EDGE('',*,*,#19638,.F.);
#27210=ORIENTED_EDGE('',*,*,#19335,.F.);
#27211=ORIENTED_EDGE('',*,*,#19639,.F.);
#27212=ORIENTED_EDGE('',*,*,#19640,.F.);
#27213=ORIENTED_EDGE('',*,*,#19634,.T.);
#27214=ORIENTED_EDGE('',*,*,#19340,.F.);
#27215=ORIENTED_EDGE('',*,*,#19641,.F.);
#27216=ORIENTED_EDGE('',*,*,#19642,.F.);
#27217=ORIENTED_EDGE('',*,*,#19643,.T.);
#27218=ORIENTED_EDGE('',*,*,#19341,.F.);
#27219=ORIENTED_EDGE('',*,*,#19643,.F.);
#27220=ORIENTED_EDGE('',*,*,#19644,.F.);
#27221=ORIENTED_EDGE('',*,*,#19645,.F.);
#27222=ORIENTED_EDGE('',*,*,#19339,.F.);
#27223=ORIENTED_EDGE('',*,*,#19646,.F.);
#27224=ORIENTED_EDGE('',*,*,#19647,.F.);
#27225=ORIENTED_EDGE('',*,*,#19641,.T.);
#27226=ORIENTED_EDGE('',*,*,#19344,.F.);
#27227=ORIENTED_EDGE('',*,*,#19648,.F.);
#27228=ORIENTED_EDGE('',*,*,#19649,.F.);
#27229=ORIENTED_EDGE('',*,*,#19650,.T.);
#27230=ORIENTED_EDGE('',*,*,#19345,.F.);
#27231=ORIENTED_EDGE('',*,*,#19650,.F.);
#27232=ORIENTED_EDGE('',*,*,#19651,.F.);
#27233=ORIENTED_EDGE('',*,*,#19652,.F.);
#27234=ORIENTED_EDGE('',*,*,#19343,.F.);
#27235=ORIENTED_EDGE('',*,*,#19653,.F.);
#27236=ORIENTED_EDGE('',*,*,#19654,.F.);
#27237=ORIENTED_EDGE('',*,*,#19648,.T.);
#27238=ORIENTED_EDGE('',*,*,#19348,.F.);
#27239=ORIENTED_EDGE('',*,*,#19655,.F.);
#27240=ORIENTED_EDGE('',*,*,#19656,.F.);
#27241=ORIENTED_EDGE('',*,*,#19657,.T.);
#27242=ORIENTED_EDGE('',*,*,#19349,.F.);
#27243=ORIENTED_EDGE('',*,*,#19657,.F.);
#27244=ORIENTED_EDGE('',*,*,#19658,.F.);
#27245=ORIENTED_EDGE('',*,*,#19659,.F.);
#27246=ORIENTED_EDGE('',*,*,#19347,.F.);
#27247=ORIENTED_EDGE('',*,*,#19660,.F.);
#27248=ORIENTED_EDGE('',*,*,#19661,.F.);
#27249=ORIENTED_EDGE('',*,*,#19655,.T.);
#27250=ORIENTED_EDGE('',*,*,#19352,.F.);
#27251=ORIENTED_EDGE('',*,*,#19662,.F.);
#27252=ORIENTED_EDGE('',*,*,#19663,.F.);
#27253=ORIENTED_EDGE('',*,*,#19664,.T.);
#27254=ORIENTED_EDGE('',*,*,#19353,.F.);
#27255=ORIENTED_EDGE('',*,*,#19664,.F.);
#27256=ORIENTED_EDGE('',*,*,#19665,.F.);
#27257=ORIENTED_EDGE('',*,*,#19666,.F.);
#27258=ORIENTED_EDGE('',*,*,#19351,.F.);
#27259=ORIENTED_EDGE('',*,*,#19667,.F.);
#27260=ORIENTED_EDGE('',*,*,#19668,.F.);
#27261=ORIENTED_EDGE('',*,*,#19662,.T.);
#27262=ORIENTED_EDGE('',*,*,#19356,.F.);
#27263=ORIENTED_EDGE('',*,*,#19669,.F.);
#27264=ORIENTED_EDGE('',*,*,#19670,.F.);
#27265=ORIENTED_EDGE('',*,*,#19671,.T.);
#27266=ORIENTED_EDGE('',*,*,#19357,.F.);
#27267=ORIENTED_EDGE('',*,*,#19671,.F.);
#27268=ORIENTED_EDGE('',*,*,#19672,.F.);
#27269=ORIENTED_EDGE('',*,*,#19673,.F.);
#27270=ORIENTED_EDGE('',*,*,#19355,.F.);
#27271=ORIENTED_EDGE('',*,*,#19674,.F.);
#27272=ORIENTED_EDGE('',*,*,#19675,.F.);
#27273=ORIENTED_EDGE('',*,*,#19669,.T.);
#27274=ORIENTED_EDGE('',*,*,#19360,.F.);
#27275=ORIENTED_EDGE('',*,*,#19676,.F.);
#27276=ORIENTED_EDGE('',*,*,#19677,.F.);
#27277=ORIENTED_EDGE('',*,*,#19678,.T.);
#27278=ORIENTED_EDGE('',*,*,#19361,.F.);
#27279=ORIENTED_EDGE('',*,*,#19678,.F.);
#27280=ORIENTED_EDGE('',*,*,#19679,.F.);
#27281=ORIENTED_EDGE('',*,*,#19680,.F.);
#27282=ORIENTED_EDGE('',*,*,#19359,.F.);
#27283=ORIENTED_EDGE('',*,*,#19681,.F.);
#27284=ORIENTED_EDGE('',*,*,#19682,.F.);
#27285=ORIENTED_EDGE('',*,*,#19676,.T.);
#27286=ORIENTED_EDGE('',*,*,#19364,.F.);
#27287=ORIENTED_EDGE('',*,*,#19683,.F.);
#27288=ORIENTED_EDGE('',*,*,#19684,.F.);
#27289=ORIENTED_EDGE('',*,*,#19685,.T.);
#27290=ORIENTED_EDGE('',*,*,#19365,.F.);
#27291=ORIENTED_EDGE('',*,*,#19685,.F.);
#27292=ORIENTED_EDGE('',*,*,#19686,.F.);
#27293=ORIENTED_EDGE('',*,*,#19687,.F.);
#27294=ORIENTED_EDGE('',*,*,#19363,.F.);
#27295=ORIENTED_EDGE('',*,*,#19688,.F.);
#27296=ORIENTED_EDGE('',*,*,#19689,.F.);
#27297=ORIENTED_EDGE('',*,*,#19683,.T.);
#27298=ORIENTED_EDGE('',*,*,#19368,.F.);
#27299=ORIENTED_EDGE('',*,*,#19690,.F.);
#27300=ORIENTED_EDGE('',*,*,#19691,.F.);
#27301=ORIENTED_EDGE('',*,*,#19692,.T.);
#27302=ORIENTED_EDGE('',*,*,#19369,.F.);
#27303=ORIENTED_EDGE('',*,*,#19692,.F.);
#27304=ORIENTED_EDGE('',*,*,#19693,.F.);
#27305=ORIENTED_EDGE('',*,*,#19694,.F.);
#27306=ORIENTED_EDGE('',*,*,#19367,.F.);
#27307=ORIENTED_EDGE('',*,*,#19695,.F.);
#27308=ORIENTED_EDGE('',*,*,#19696,.F.);
#27309=ORIENTED_EDGE('',*,*,#19690,.T.);
#27310=ORIENTED_EDGE('',*,*,#19372,.F.);
#27311=ORIENTED_EDGE('',*,*,#19697,.F.);
#27312=ORIENTED_EDGE('',*,*,#19698,.F.);
#27313=ORIENTED_EDGE('',*,*,#19699,.T.);
#27314=ORIENTED_EDGE('',*,*,#19373,.F.);
#27315=ORIENTED_EDGE('',*,*,#19699,.F.);
#27316=ORIENTED_EDGE('',*,*,#19700,.F.);
#27317=ORIENTED_EDGE('',*,*,#19701,.F.);
#27318=ORIENTED_EDGE('',*,*,#19371,.F.);
#27319=ORIENTED_EDGE('',*,*,#19702,.F.);
#27320=ORIENTED_EDGE('',*,*,#19703,.F.);
#27321=ORIENTED_EDGE('',*,*,#19697,.T.);
#27322=ORIENTED_EDGE('',*,*,#19376,.F.);
#27323=ORIENTED_EDGE('',*,*,#19704,.F.);
#27324=ORIENTED_EDGE('',*,*,#19705,.F.);
#27325=ORIENTED_EDGE('',*,*,#19706,.T.);
#27326=ORIENTED_EDGE('',*,*,#19377,.F.);
#27327=ORIENTED_EDGE('',*,*,#19706,.F.);
#27328=ORIENTED_EDGE('',*,*,#19707,.F.);
#27329=ORIENTED_EDGE('',*,*,#19708,.F.);
#27330=ORIENTED_EDGE('',*,*,#19375,.F.);
#27331=ORIENTED_EDGE('',*,*,#19709,.F.);
#27332=ORIENTED_EDGE('',*,*,#19710,.F.);
#27333=ORIENTED_EDGE('',*,*,#19704,.T.);
#27334=ORIENTED_EDGE('',*,*,#19380,.F.);
#27335=ORIENTED_EDGE('',*,*,#19711,.F.);
#27336=ORIENTED_EDGE('',*,*,#19712,.F.);
#27337=ORIENTED_EDGE('',*,*,#19713,.T.);
#27338=ORIENTED_EDGE('',*,*,#19381,.F.);
#27339=ORIENTED_EDGE('',*,*,#19713,.F.);
#27340=ORIENTED_EDGE('',*,*,#19714,.F.);
#27341=ORIENTED_EDGE('',*,*,#19715,.F.);
#27342=ORIENTED_EDGE('',*,*,#19379,.F.);
#27343=ORIENTED_EDGE('',*,*,#19716,.F.);
#27344=ORIENTED_EDGE('',*,*,#19717,.F.);
#27345=ORIENTED_EDGE('',*,*,#19711,.T.);
#27346=ORIENTED_EDGE('',*,*,#19384,.F.);
#27347=ORIENTED_EDGE('',*,*,#19718,.F.);
#27348=ORIENTED_EDGE('',*,*,#19719,.F.);
#27349=ORIENTED_EDGE('',*,*,#19720,.T.);
#27350=ORIENTED_EDGE('',*,*,#19385,.F.);
#27351=ORIENTED_EDGE('',*,*,#19720,.F.);
#27352=ORIENTED_EDGE('',*,*,#19721,.F.);
#27353=ORIENTED_EDGE('',*,*,#19722,.F.);
#27354=ORIENTED_EDGE('',*,*,#19383,.F.);
#27355=ORIENTED_EDGE('',*,*,#19723,.F.);
#27356=ORIENTED_EDGE('',*,*,#19724,.F.);
#27357=ORIENTED_EDGE('',*,*,#19718,.T.);
#27358=ORIENTED_EDGE('',*,*,#19388,.F.);
#27359=ORIENTED_EDGE('',*,*,#19725,.F.);
#27360=ORIENTED_EDGE('',*,*,#19726,.F.);
#27361=ORIENTED_EDGE('',*,*,#19727,.T.);
#27362=ORIENTED_EDGE('',*,*,#19389,.F.);
#27363=ORIENTED_EDGE('',*,*,#19727,.F.);
#27364=ORIENTED_EDGE('',*,*,#19728,.F.);
#27365=ORIENTED_EDGE('',*,*,#19729,.F.);
#27366=ORIENTED_EDGE('',*,*,#19387,.F.);
#27367=ORIENTED_EDGE('',*,*,#19730,.F.);
#27368=ORIENTED_EDGE('',*,*,#19731,.F.);
#27369=ORIENTED_EDGE('',*,*,#19725,.T.);
#27370=ORIENTED_EDGE('',*,*,#19729,.T.);
#27371=ORIENTED_EDGE('',*,*,#19732,.F.);
#27372=ORIENTED_EDGE('',*,*,#19733,.T.);
#27373=ORIENTED_EDGE('',*,*,#19390,.T.);
#27374=ORIENTED_EDGE('',*,*,#19722,.T.);
#27375=ORIENTED_EDGE('',*,*,#19734,.F.);
#27376=ORIENTED_EDGE('',*,*,#19730,.T.);
#27377=ORIENTED_EDGE('',*,*,#19386,.T.);
#27378=ORIENTED_EDGE('',*,*,#19715,.T.);
#27379=ORIENTED_EDGE('',*,*,#19735,.F.);
#27380=ORIENTED_EDGE('',*,*,#19723,.T.);
#27381=ORIENTED_EDGE('',*,*,#19382,.T.);
#27382=ORIENTED_EDGE('',*,*,#19708,.T.);
#27383=ORIENTED_EDGE('',*,*,#19736,.F.);
#27384=ORIENTED_EDGE('',*,*,#19716,.T.);
#27385=ORIENTED_EDGE('',*,*,#19378,.T.);
#27386=ORIENTED_EDGE('',*,*,#19701,.T.);
#27387=ORIENTED_EDGE('',*,*,#19737,.F.);
#27388=ORIENTED_EDGE('',*,*,#19709,.T.);
#27389=ORIENTED_EDGE('',*,*,#19374,.T.);
#27390=ORIENTED_EDGE('',*,*,#19694,.T.);
#27391=ORIENTED_EDGE('',*,*,#19738,.F.);
#27392=ORIENTED_EDGE('',*,*,#19702,.T.);
#27393=ORIENTED_EDGE('',*,*,#19370,.T.);
#27394=ORIENTED_EDGE('',*,*,#19687,.T.);
#27395=ORIENTED_EDGE('',*,*,#19739,.F.);
#27396=ORIENTED_EDGE('',*,*,#19695,.T.);
#27397=ORIENTED_EDGE('',*,*,#19366,.T.);
#27398=ORIENTED_EDGE('',*,*,#19680,.T.);
#27399=ORIENTED_EDGE('',*,*,#19740,.F.);
#27400=ORIENTED_EDGE('',*,*,#19688,.T.);
#27401=ORIENTED_EDGE('',*,*,#19362,.T.);
#27402=ORIENTED_EDGE('',*,*,#19673,.T.);
#27403=ORIENTED_EDGE('',*,*,#19741,.F.);
#27404=ORIENTED_EDGE('',*,*,#19681,.T.);
#27405=ORIENTED_EDGE('',*,*,#19358,.T.);
#27406=ORIENTED_EDGE('',*,*,#19666,.T.);
#27407=ORIENTED_EDGE('',*,*,#19742,.F.);
#27408=ORIENTED_EDGE('',*,*,#19674,.T.);
#27409=ORIENTED_EDGE('',*,*,#19354,.T.);
#27410=ORIENTED_EDGE('',*,*,#19659,.T.);
#27411=ORIENTED_EDGE('',*,*,#19743,.F.);
#27412=ORIENTED_EDGE('',*,*,#19667,.T.);
#27413=ORIENTED_EDGE('',*,*,#19350,.T.);
#27414=ORIENTED_EDGE('',*,*,#19652,.T.);
#27415=ORIENTED_EDGE('',*,*,#19744,.F.);
#27416=ORIENTED_EDGE('',*,*,#19660,.T.);
#27417=ORIENTED_EDGE('',*,*,#19346,.T.);
#27418=ORIENTED_EDGE('',*,*,#19645,.T.);
#27419=ORIENTED_EDGE('',*,*,#19745,.F.);
#27420=ORIENTED_EDGE('',*,*,#19653,.T.);
#27421=ORIENTED_EDGE('',*,*,#19342,.T.);
#27422=ORIENTED_EDGE('',*,*,#19638,.T.);
#27423=ORIENTED_EDGE('',*,*,#19746,.F.);
#27424=ORIENTED_EDGE('',*,*,#19646,.T.);
#27425=ORIENTED_EDGE('',*,*,#19338,.T.);
#27426=ORIENTED_EDGE('',*,*,#19631,.T.);
#27427=ORIENTED_EDGE('',*,*,#19747,.F.);
#27428=ORIENTED_EDGE('',*,*,#19639,.T.);
#27429=ORIENTED_EDGE('',*,*,#19334,.T.);
#27430=ORIENTED_EDGE('',*,*,#19624,.T.);
#27431=ORIENTED_EDGE('',*,*,#19748,.F.);
#27432=ORIENTED_EDGE('',*,*,#19632,.T.);
#27433=ORIENTED_EDGE('',*,*,#19330,.T.);
#27434=ORIENTED_EDGE('',*,*,#19617,.T.);
#27435=ORIENTED_EDGE('',*,*,#19749,.F.);
#27436=ORIENTED_EDGE('',*,*,#19625,.T.);
#27437=ORIENTED_EDGE('',*,*,#19326,.T.);
#27438=ORIENTED_EDGE('',*,*,#19610,.T.);
#27439=ORIENTED_EDGE('',*,*,#19750,.F.);
#27440=ORIENTED_EDGE('',*,*,#19618,.T.);
#27441=ORIENTED_EDGE('',*,*,#19322,.T.);
#27442=ORIENTED_EDGE('',*,*,#19603,.T.);
#27443=ORIENTED_EDGE('',*,*,#19751,.F.);
#27444=ORIENTED_EDGE('',*,*,#19611,.T.);
#27445=ORIENTED_EDGE('',*,*,#19318,.T.);
#27446=ORIENTED_EDGE('',*,*,#19596,.T.);
#27447=ORIENTED_EDGE('',*,*,#19752,.F.);
#27448=ORIENTED_EDGE('',*,*,#19604,.T.);
#27449=ORIENTED_EDGE('',*,*,#19314,.T.);
#27450=ORIENTED_EDGE('',*,*,#19589,.T.);
#27451=ORIENTED_EDGE('',*,*,#19753,.F.);
#27452=ORIENTED_EDGE('',*,*,#19597,.T.);
#27453=ORIENTED_EDGE('',*,*,#19310,.T.);
#27454=ORIENTED_EDGE('',*,*,#19582,.T.);
#27455=ORIENTED_EDGE('',*,*,#19754,.F.);
#27456=ORIENTED_EDGE('',*,*,#19590,.T.);
#27457=ORIENTED_EDGE('',*,*,#19306,.T.);
#27458=ORIENTED_EDGE('',*,*,#19575,.T.);
#27459=ORIENTED_EDGE('',*,*,#19755,.F.);
#27460=ORIENTED_EDGE('',*,*,#19583,.T.);
#27461=ORIENTED_EDGE('',*,*,#19302,.T.);
#27462=ORIENTED_EDGE('',*,*,#19568,.T.);
#27463=ORIENTED_EDGE('',*,*,#19756,.F.);
#27464=ORIENTED_EDGE('',*,*,#19576,.T.);
#27465=ORIENTED_EDGE('',*,*,#19298,.T.);
#27466=ORIENTED_EDGE('',*,*,#19561,.T.);
#27467=ORIENTED_EDGE('',*,*,#19757,.F.);
#27468=ORIENTED_EDGE('',*,*,#19569,.T.);
#27469=ORIENTED_EDGE('',*,*,#19294,.T.);
#27470=ORIENTED_EDGE('',*,*,#19554,.T.);
#27471=ORIENTED_EDGE('',*,*,#19758,.F.);
#27472=ORIENTED_EDGE('',*,*,#19562,.T.);
#27473=ORIENTED_EDGE('',*,*,#19290,.T.);
#27474=ORIENTED_EDGE('',*,*,#19547,.T.);
#27475=ORIENTED_EDGE('',*,*,#19759,.F.);
#27476=ORIENTED_EDGE('',*,*,#19555,.T.);
#27477=ORIENTED_EDGE('',*,*,#19286,.T.);
#27478=ORIENTED_EDGE('',*,*,#19540,.T.);
#27479=ORIENTED_EDGE('',*,*,#19760,.F.);
#27480=ORIENTED_EDGE('',*,*,#19548,.T.);
#27481=ORIENTED_EDGE('',*,*,#19282,.T.);
#27482=ORIENTED_EDGE('',*,*,#19533,.T.);
#27483=ORIENTED_EDGE('',*,*,#19761,.F.);
#27484=ORIENTED_EDGE('',*,*,#19541,.T.);
#27485=ORIENTED_EDGE('',*,*,#19278,.T.);
#27486=ORIENTED_EDGE('',*,*,#19526,.T.);
#27487=ORIENTED_EDGE('',*,*,#19762,.F.);
#27488=ORIENTED_EDGE('',*,*,#19534,.T.);
#27489=ORIENTED_EDGE('',*,*,#19274,.T.);
#27490=ORIENTED_EDGE('',*,*,#19519,.T.);
#27491=ORIENTED_EDGE('',*,*,#19763,.F.);
#27492=ORIENTED_EDGE('',*,*,#19527,.T.);
#27493=ORIENTED_EDGE('',*,*,#19270,.T.);
#27494=ORIENTED_EDGE('',*,*,#19512,.T.);
#27495=ORIENTED_EDGE('',*,*,#19764,.F.);
#27496=ORIENTED_EDGE('',*,*,#19520,.T.);
#27497=ORIENTED_EDGE('',*,*,#19266,.T.);
#27498=ORIENTED_EDGE('',*,*,#19505,.T.);
#27499=ORIENTED_EDGE('',*,*,#19765,.F.);
#27500=ORIENTED_EDGE('',*,*,#19513,.T.);
#27501=ORIENTED_EDGE('',*,*,#19262,.T.);
#27502=ORIENTED_EDGE('',*,*,#19498,.T.);
#27503=ORIENTED_EDGE('',*,*,#19766,.F.);
#27504=ORIENTED_EDGE('',*,*,#19506,.T.);
#27505=ORIENTED_EDGE('',*,*,#19258,.T.);
#27506=ORIENTED_EDGE('',*,*,#19491,.T.);
#27507=ORIENTED_EDGE('',*,*,#19767,.F.);
#27508=ORIENTED_EDGE('',*,*,#19499,.T.);
#27509=ORIENTED_EDGE('',*,*,#19254,.T.);
#27510=ORIENTED_EDGE('',*,*,#19484,.T.);
#27511=ORIENTED_EDGE('',*,*,#19768,.F.);
#27512=ORIENTED_EDGE('',*,*,#19492,.T.);
#27513=ORIENTED_EDGE('',*,*,#19250,.T.);
#27514=ORIENTED_EDGE('',*,*,#19477,.T.);
#27515=ORIENTED_EDGE('',*,*,#19769,.F.);
#27516=ORIENTED_EDGE('',*,*,#19485,.T.);
#27517=ORIENTED_EDGE('',*,*,#19246,.T.);
#27518=ORIENTED_EDGE('',*,*,#19470,.T.);
#27519=ORIENTED_EDGE('',*,*,#19770,.F.);
#27520=ORIENTED_EDGE('',*,*,#19478,.T.);
#27521=ORIENTED_EDGE('',*,*,#19242,.T.);
#27522=ORIENTED_EDGE('',*,*,#19463,.T.);
#27523=ORIENTED_EDGE('',*,*,#19771,.F.);
#27524=ORIENTED_EDGE('',*,*,#19471,.T.);
#27525=ORIENTED_EDGE('',*,*,#19238,.T.);
#27526=ORIENTED_EDGE('',*,*,#19456,.T.);
#27527=ORIENTED_EDGE('',*,*,#19772,.F.);
#27528=ORIENTED_EDGE('',*,*,#19464,.T.);
#27529=ORIENTED_EDGE('',*,*,#19234,.T.);
#27530=ORIENTED_EDGE('',*,*,#19449,.T.);
#27531=ORIENTED_EDGE('',*,*,#19773,.F.);
#27532=ORIENTED_EDGE('',*,*,#19457,.T.);
#27533=ORIENTED_EDGE('',*,*,#19230,.T.);
#27534=ORIENTED_EDGE('',*,*,#19442,.T.);
#27535=ORIENTED_EDGE('',*,*,#19774,.F.);
#27536=ORIENTED_EDGE('',*,*,#19450,.T.);
#27537=ORIENTED_EDGE('',*,*,#19226,.T.);
#27538=ORIENTED_EDGE('',*,*,#19435,.T.);
#27539=ORIENTED_EDGE('',*,*,#19775,.F.);
#27540=ORIENTED_EDGE('',*,*,#19443,.T.);
#27541=ORIENTED_EDGE('',*,*,#19222,.T.);
#27542=ORIENTED_EDGE('',*,*,#19428,.T.);
#27543=ORIENTED_EDGE('',*,*,#19776,.F.);
#27544=ORIENTED_EDGE('',*,*,#19436,.T.);
#27545=ORIENTED_EDGE('',*,*,#19218,.T.);
#27546=ORIENTED_EDGE('',*,*,#19421,.T.);
#27547=ORIENTED_EDGE('',*,*,#19777,.F.);
#27548=ORIENTED_EDGE('',*,*,#19429,.T.);
#27549=ORIENTED_EDGE('',*,*,#19214,.T.);
#27550=ORIENTED_EDGE('',*,*,#19414,.T.);
#27551=ORIENTED_EDGE('',*,*,#19778,.F.);
#27552=ORIENTED_EDGE('',*,*,#19422,.T.);
#27553=ORIENTED_EDGE('',*,*,#19210,.T.);
#27554=ORIENTED_EDGE('',*,*,#19407,.T.);
#27555=ORIENTED_EDGE('',*,*,#19779,.F.);
#27556=ORIENTED_EDGE('',*,*,#19415,.T.);
#27557=ORIENTED_EDGE('',*,*,#19206,.T.);
#27558=ORIENTED_EDGE('',*,*,#19392,.F.);
#27559=ORIENTED_EDGE('',*,*,#19780,.F.);
#27560=ORIENTED_EDGE('',*,*,#19781,.F.);
#27561=ORIENTED_EDGE('',*,*,#19782,.T.);
#27562=ORIENTED_EDGE('',*,*,#19393,.F.);
#27563=ORIENTED_EDGE('',*,*,#19782,.F.);
#27564=ORIENTED_EDGE('',*,*,#19783,.F.);
#27565=ORIENTED_EDGE('',*,*,#19784,.F.);
#27566=ORIENTED_EDGE('',*,*,#19391,.F.);
#27567=ORIENTED_EDGE('',*,*,#19733,.F.);
#27568=ORIENTED_EDGE('',*,*,#19785,.F.);
#27569=ORIENTED_EDGE('',*,*,#19780,.T.);
#27570=ORIENTED_EDGE('',*,*,#19408,.T.);
#27571=ORIENTED_EDGE('',*,*,#19394,.T.);
#27572=ORIENTED_EDGE('',*,*,#19784,.T.);
#27573=ORIENTED_EDGE('',*,*,#19786,.F.);
#27574=ORIENTED_EDGE('',*,*,#19409,.T.);
#27575=ORIENTED_EDGE('',*,*,#19786,.T.);
#27576=ORIENTED_EDGE('',*,*,#19783,.T.);
#27577=ORIENTED_EDGE('',*,*,#19781,.T.);
#27578=ORIENTED_EDGE('',*,*,#19785,.T.);
#27579=ORIENTED_EDGE('',*,*,#19732,.T.);
#27580=ORIENTED_EDGE('',*,*,#19728,.T.);
#27581=ORIENTED_EDGE('',*,*,#19726,.T.);
#27582=ORIENTED_EDGE('',*,*,#19731,.T.);
#27583=ORIENTED_EDGE('',*,*,#19734,.T.);
#27584=ORIENTED_EDGE('',*,*,#19721,.T.);
#27585=ORIENTED_EDGE('',*,*,#19719,.T.);
#27586=ORIENTED_EDGE('',*,*,#19724,.T.);
#27587=ORIENTED_EDGE('',*,*,#19735,.T.);
#27588=ORIENTED_EDGE('',*,*,#19714,.T.);
#27589=ORIENTED_EDGE('',*,*,#19712,.T.);
#27590=ORIENTED_EDGE('',*,*,#19717,.T.);
#27591=ORIENTED_EDGE('',*,*,#19736,.T.);
#27592=ORIENTED_EDGE('',*,*,#19707,.T.);
#27593=ORIENTED_EDGE('',*,*,#19705,.T.);
#27594=ORIENTED_EDGE('',*,*,#19710,.T.);
#27595=ORIENTED_EDGE('',*,*,#19737,.T.);
#27596=ORIENTED_EDGE('',*,*,#19700,.T.);
#27597=ORIENTED_EDGE('',*,*,#19698,.T.);
#27598=ORIENTED_EDGE('',*,*,#19703,.T.);
#27599=ORIENTED_EDGE('',*,*,#19738,.T.);
#27600=ORIENTED_EDGE('',*,*,#19693,.T.);
#27601=ORIENTED_EDGE('',*,*,#19691,.T.);
#27602=ORIENTED_EDGE('',*,*,#19696,.T.);
#27603=ORIENTED_EDGE('',*,*,#19739,.T.);
#27604=ORIENTED_EDGE('',*,*,#19686,.T.);
#27605=ORIENTED_EDGE('',*,*,#19684,.T.);
#27606=ORIENTED_EDGE('',*,*,#19689,.T.);
#27607=ORIENTED_EDGE('',*,*,#19740,.T.);
#27608=ORIENTED_EDGE('',*,*,#19679,.T.);
#27609=ORIENTED_EDGE('',*,*,#19677,.T.);
#27610=ORIENTED_EDGE('',*,*,#19682,.T.);
#27611=ORIENTED_EDGE('',*,*,#19741,.T.);
#27612=ORIENTED_EDGE('',*,*,#19672,.T.);
#27613=ORIENTED_EDGE('',*,*,#19670,.T.);
#27614=ORIENTED_EDGE('',*,*,#19675,.T.);
#27615=ORIENTED_EDGE('',*,*,#19742,.T.);
#27616=ORIENTED_EDGE('',*,*,#19665,.T.);
#27617=ORIENTED_EDGE('',*,*,#19663,.T.);
#27618=ORIENTED_EDGE('',*,*,#19668,.T.);
#27619=ORIENTED_EDGE('',*,*,#19743,.T.);
#27620=ORIENTED_EDGE('',*,*,#19658,.T.);
#27621=ORIENTED_EDGE('',*,*,#19656,.T.);
#27622=ORIENTED_EDGE('',*,*,#19661,.T.);
#27623=ORIENTED_EDGE('',*,*,#19744,.T.);
#27624=ORIENTED_EDGE('',*,*,#19651,.T.);
#27625=ORIENTED_EDGE('',*,*,#19649,.T.);
#27626=ORIENTED_EDGE('',*,*,#19654,.T.);
#27627=ORIENTED_EDGE('',*,*,#19745,.T.);
#27628=ORIENTED_EDGE('',*,*,#19644,.T.);
#27629=ORIENTED_EDGE('',*,*,#19642,.T.);
#27630=ORIENTED_EDGE('',*,*,#19647,.T.);
#27631=ORIENTED_EDGE('',*,*,#19746,.T.);
#27632=ORIENTED_EDGE('',*,*,#19637,.T.);
#27633=ORIENTED_EDGE('',*,*,#19635,.T.);
#27634=ORIENTED_EDGE('',*,*,#19640,.T.);
#27635=ORIENTED_EDGE('',*,*,#19747,.T.);
#27636=ORIENTED_EDGE('',*,*,#19630,.T.);
#27637=ORIENTED_EDGE('',*,*,#19628,.T.);
#27638=ORIENTED_EDGE('',*,*,#19633,.T.);
#27639=ORIENTED_EDGE('',*,*,#19748,.T.);
#27640=ORIENTED_EDGE('',*,*,#19623,.T.);
#27641=ORIENTED_EDGE('',*,*,#19621,.T.);
#27642=ORIENTED_EDGE('',*,*,#19626,.T.);
#27643=ORIENTED_EDGE('',*,*,#19749,.T.);
#27644=ORIENTED_EDGE('',*,*,#19616,.T.);
#27645=ORIENTED_EDGE('',*,*,#19614,.T.);
#27646=ORIENTED_EDGE('',*,*,#19619,.T.);
#27647=ORIENTED_EDGE('',*,*,#19750,.T.);
#27648=ORIENTED_EDGE('',*,*,#19609,.T.);
#27649=ORIENTED_EDGE('',*,*,#19607,.T.);
#27650=ORIENTED_EDGE('',*,*,#19612,.T.);
#27651=ORIENTED_EDGE('',*,*,#19751,.T.);
#27652=ORIENTED_EDGE('',*,*,#19602,.T.);
#27653=ORIENTED_EDGE('',*,*,#19600,.T.);
#27654=ORIENTED_EDGE('',*,*,#19605,.T.);
#27655=ORIENTED_EDGE('',*,*,#19752,.T.);
#27656=ORIENTED_EDGE('',*,*,#19595,.T.);
#27657=ORIENTED_EDGE('',*,*,#19593,.T.);
#27658=ORIENTED_EDGE('',*,*,#19598,.T.);
#27659=ORIENTED_EDGE('',*,*,#19753,.T.);
#27660=ORIENTED_EDGE('',*,*,#19588,.T.);
#27661=ORIENTED_EDGE('',*,*,#19586,.T.);
#27662=ORIENTED_EDGE('',*,*,#19591,.T.);
#27663=ORIENTED_EDGE('',*,*,#19754,.T.);
#27664=ORIENTED_EDGE('',*,*,#19581,.T.);
#27665=ORIENTED_EDGE('',*,*,#19579,.T.);
#27666=ORIENTED_EDGE('',*,*,#19584,.T.);
#27667=ORIENTED_EDGE('',*,*,#19755,.T.);
#27668=ORIENTED_EDGE('',*,*,#19574,.T.);
#27669=ORIENTED_EDGE('',*,*,#19572,.T.);
#27670=ORIENTED_EDGE('',*,*,#19577,.T.);
#27671=ORIENTED_EDGE('',*,*,#19756,.T.);
#27672=ORIENTED_EDGE('',*,*,#19567,.T.);
#27673=ORIENTED_EDGE('',*,*,#19565,.T.);
#27674=ORIENTED_EDGE('',*,*,#19570,.T.);
#27675=ORIENTED_EDGE('',*,*,#19757,.T.);
#27676=ORIENTED_EDGE('',*,*,#19560,.T.);
#27677=ORIENTED_EDGE('',*,*,#19558,.T.);
#27678=ORIENTED_EDGE('',*,*,#19563,.T.);
#27679=ORIENTED_EDGE('',*,*,#19758,.T.);
#27680=ORIENTED_EDGE('',*,*,#19553,.T.);
#27681=ORIENTED_EDGE('',*,*,#19551,.T.);
#27682=ORIENTED_EDGE('',*,*,#19556,.T.);
#27683=ORIENTED_EDGE('',*,*,#19759,.T.);
#27684=ORIENTED_EDGE('',*,*,#19546,.T.);
#27685=ORIENTED_EDGE('',*,*,#19544,.T.);
#27686=ORIENTED_EDGE('',*,*,#19549,.T.);
#27687=ORIENTED_EDGE('',*,*,#19760,.T.);
#27688=ORIENTED_EDGE('',*,*,#19539,.T.);
#27689=ORIENTED_EDGE('',*,*,#19537,.T.);
#27690=ORIENTED_EDGE('',*,*,#19542,.T.);
#27691=ORIENTED_EDGE('',*,*,#19761,.T.);
#27692=ORIENTED_EDGE('',*,*,#19532,.T.);
#27693=ORIENTED_EDGE('',*,*,#19530,.T.);
#27694=ORIENTED_EDGE('',*,*,#19535,.T.);
#27695=ORIENTED_EDGE('',*,*,#19762,.T.);
#27696=ORIENTED_EDGE('',*,*,#19525,.T.);
#27697=ORIENTED_EDGE('',*,*,#19523,.T.);
#27698=ORIENTED_EDGE('',*,*,#19528,.T.);
#27699=ORIENTED_EDGE('',*,*,#19763,.T.);
#27700=ORIENTED_EDGE('',*,*,#19518,.T.);
#27701=ORIENTED_EDGE('',*,*,#19516,.T.);
#27702=ORIENTED_EDGE('',*,*,#19521,.T.);
#27703=ORIENTED_EDGE('',*,*,#19764,.T.);
#27704=ORIENTED_EDGE('',*,*,#19511,.T.);
#27705=ORIENTED_EDGE('',*,*,#19509,.T.);
#27706=ORIENTED_EDGE('',*,*,#19514,.T.);
#27707=ORIENTED_EDGE('',*,*,#19765,.T.);
#27708=ORIENTED_EDGE('',*,*,#19504,.T.);
#27709=ORIENTED_EDGE('',*,*,#19502,.T.);
#27710=ORIENTED_EDGE('',*,*,#19507,.T.);
#27711=ORIENTED_EDGE('',*,*,#19766,.T.);
#27712=ORIENTED_EDGE('',*,*,#19497,.T.);
#27713=ORIENTED_EDGE('',*,*,#19495,.T.);
#27714=ORIENTED_EDGE('',*,*,#19500,.T.);
#27715=ORIENTED_EDGE('',*,*,#19767,.T.);
#27716=ORIENTED_EDGE('',*,*,#19490,.T.);
#27717=ORIENTED_EDGE('',*,*,#19488,.T.);
#27718=ORIENTED_EDGE('',*,*,#19493,.T.);
#27719=ORIENTED_EDGE('',*,*,#19768,.T.);
#27720=ORIENTED_EDGE('',*,*,#19483,.T.);
#27721=ORIENTED_EDGE('',*,*,#19481,.T.);
#27722=ORIENTED_EDGE('',*,*,#19486,.T.);
#27723=ORIENTED_EDGE('',*,*,#19769,.T.);
#27724=ORIENTED_EDGE('',*,*,#19476,.T.);
#27725=ORIENTED_EDGE('',*,*,#19474,.T.);
#27726=ORIENTED_EDGE('',*,*,#19479,.T.);
#27727=ORIENTED_EDGE('',*,*,#19770,.T.);
#27728=ORIENTED_EDGE('',*,*,#19469,.T.);
#27729=ORIENTED_EDGE('',*,*,#19467,.T.);
#27730=ORIENTED_EDGE('',*,*,#19472,.T.);
#27731=ORIENTED_EDGE('',*,*,#19771,.T.);
#27732=ORIENTED_EDGE('',*,*,#19462,.T.);
#27733=ORIENTED_EDGE('',*,*,#19460,.T.);
#27734=ORIENTED_EDGE('',*,*,#19465,.T.);
#27735=ORIENTED_EDGE('',*,*,#19772,.T.);
#27736=ORIENTED_EDGE('',*,*,#19455,.T.);
#27737=ORIENTED_EDGE('',*,*,#19453,.T.);
#27738=ORIENTED_EDGE('',*,*,#19458,.T.);
#27739=ORIENTED_EDGE('',*,*,#19773,.T.);
#27740=ORIENTED_EDGE('',*,*,#19448,.T.);
#27741=ORIENTED_EDGE('',*,*,#19446,.T.);
#27742=ORIENTED_EDGE('',*,*,#19451,.T.);
#27743=ORIENTED_EDGE('',*,*,#19774,.T.);
#27744=ORIENTED_EDGE('',*,*,#19441,.T.);
#27745=ORIENTED_EDGE('',*,*,#19439,.T.);
#27746=ORIENTED_EDGE('',*,*,#19444,.T.);
#27747=ORIENTED_EDGE('',*,*,#19775,.T.);
#27748=ORIENTED_EDGE('',*,*,#19434,.T.);
#27749=ORIENTED_EDGE('',*,*,#19432,.T.);
#27750=ORIENTED_EDGE('',*,*,#19437,.T.);
#27751=ORIENTED_EDGE('',*,*,#19776,.T.);
#27752=ORIENTED_EDGE('',*,*,#19427,.T.);
#27753=ORIENTED_EDGE('',*,*,#19425,.T.);
#27754=ORIENTED_EDGE('',*,*,#19430,.T.);
#27755=ORIENTED_EDGE('',*,*,#19777,.T.);
#27756=ORIENTED_EDGE('',*,*,#19420,.T.);
#27757=ORIENTED_EDGE('',*,*,#19418,.T.);
#27758=ORIENTED_EDGE('',*,*,#19423,.T.);
#27759=ORIENTED_EDGE('',*,*,#19778,.T.);
#27760=ORIENTED_EDGE('',*,*,#19413,.T.);
#27761=ORIENTED_EDGE('',*,*,#19411,.T.);
#27762=ORIENTED_EDGE('',*,*,#19416,.T.);
#27763=ORIENTED_EDGE('',*,*,#19779,.T.);
#27764=ORIENTED_EDGE('',*,*,#19406,.T.);
#27765=ORIENTED_EDGE('',*,*,#19404,.T.);
#27766=ORIENTED_EDGE('',*,*,#19400,.T.);
#27767=ORIENTED_EDGE('',*,*,#19402,.T.);
#27768=ORIENTED_EDGE('',*,*,#19395,.T.);
#27769=ORIENTED_EDGE('',*,*,#19398,.T.);
#31657=PLANE('',#36156);
#31658=PLANE('',#36161);
#31659=PLANE('',#36354);
#31660=PLANE('',#36355);
#31661=PLANE('',#36358);
#31662=PLANE('',#36743);
#32953=ADVANCED_FACE('',(#5272),#906,.T.);
#32954=ADVANCED_FACE('',(#5273),#1395,.T.);
#32955=ADVANCED_FACE('',(#5274,#2131),#31657,.T.);
#32956=ADVANCED_FACE('',(#5275),#907,.F.);
#32957=ADVANCED_FACE('',(#5276,#2132),#31658,.F.);
#32958=ADVANCED_FACE('',(#5277),#31659,.F.);
#32959=ADVANCED_FACE('',(#5278),#31660,.F.);
#32960=ADVANCED_FACE('',(#5279),#1396,.F.);
#32961=ADVANCED_FACE('',(#5280),#31661,.F.);
#32962=ADVANCED_FACE('',(#5281),#1397,.T.);
#32963=ADVANCED_FACE('',(#5282),#1398,.T.);
#32964=ADVANCED_FACE('',(#5283),#1399,.T.);
#32965=ADVANCED_FACE('',(#5284),#1400,.T.);
#32966=ADVANCED_FACE('',(#5285),#1401,.T.);
#32967=ADVANCED_FACE('',(#5286),#1402,.T.);
#32968=ADVANCED_FACE('',(#5287),#1403,.T.);
#32969=ADVANCED_FACE('',(#5288),#1404,.T.);
#32970=ADVANCED_FACE('',(#5289),#1405,.T.);
#32971=ADVANCED_FACE('',(#5290),#1406,.T.);
#32972=ADVANCED_FACE('',(#5291),#1407,.T.);
#32973=ADVANCED_FACE('',(#5292),#1408,.T.);
#32974=ADVANCED_FACE('',(#5293),#1409,.T.);
#32975=ADVANCED_FACE('',(#5294),#1410,.T.);
#32976=ADVANCED_FACE('',(#5295),#1411,.T.);
#32977=ADVANCED_FACE('',(#5296),#1412,.T.);
#32978=ADVANCED_FACE('',(#5297),#1413,.T.);
#32979=ADVANCED_FACE('',(#5298),#1414,.T.);
#32980=ADVANCED_FACE('',(#5299),#1415,.T.);
#32981=ADVANCED_FACE('',(#5300),#1416,.T.);
#32982=ADVANCED_FACE('',(#5301),#1417,.T.);
#32983=ADVANCED_FACE('',(#5302),#1418,.T.);
#32984=ADVANCED_FACE('',(#5303),#1419,.T.);
#32985=ADVANCED_FACE('',(#5304),#1420,.T.);
#32986=ADVANCED_FACE('',(#5305),#1421,.T.);
#32987=ADVANCED_FACE('',(#5306),#1422,.T.);
#32988=ADVANCED_FACE('',(#5307),#1423,.T.);
#32989=ADVANCED_FACE('',(#5308),#1424,.T.);
#32990=ADVANCED_FACE('',(#5309),#1425,.T.);
#32991=ADVANCED_FACE('',(#5310),#1426,.T.);
#32992=ADVANCED_FACE('',(#5311),#1427,.T.);
#32993=ADVANCED_FACE('',(#5312),#1428,.T.);
#32994=ADVANCED_FACE('',(#5313),#1429,.T.);
#32995=ADVANCED_FACE('',(#5314),#1430,.T.);
#32996=ADVANCED_FACE('',(#5315),#1431,.T.);
#32997=ADVANCED_FACE('',(#5316),#1432,.T.);
#32998=ADVANCED_FACE('',(#5317),#1433,.T.);
#32999=ADVANCED_FACE('',(#5318),#1434,.T.);
#33000=ADVANCED_FACE('',(#5319),#1435,.T.);
#33001=ADVANCED_FACE('',(#5320),#1436,.T.);
#33002=ADVANCED_FACE('',(#5321),#1437,.T.);
#33003=ADVANCED_FACE('',(#5322),#1438,.T.);
#33004=ADVANCED_FACE('',(#5323),#1439,.T.);
#33005=ADVANCED_FACE('',(#5324),#1440,.T.);
#33006=ADVANCED_FACE('',(#5325),#1441,.T.);
#33007=ADVANCED_FACE('',(#5326),#1442,.T.);
#33008=ADVANCED_FACE('',(#5327),#1443,.T.);
#33009=ADVANCED_FACE('',(#5328),#1444,.T.);
#33010=ADVANCED_FACE('',(#5329),#1445,.T.);
#33011=ADVANCED_FACE('',(#5330),#1446,.T.);
#33012=ADVANCED_FACE('',(#5331),#1447,.T.);
#33013=ADVANCED_FACE('',(#5332),#1448,.T.);
#33014=ADVANCED_FACE('',(#5333),#1449,.T.);
#33015=ADVANCED_FACE('',(#5334),#1450,.T.);
#33016=ADVANCED_FACE('',(#5335),#1451,.T.);
#33017=ADVANCED_FACE('',(#5336),#1452,.T.);
#33018=ADVANCED_FACE('',(#5337),#1453,.T.);
#33019=ADVANCED_FACE('',(#5338),#1454,.T.);
#33020=ADVANCED_FACE('',(#5339),#1455,.T.);
#33021=ADVANCED_FACE('',(#5340),#1456,.T.);
#33022=ADVANCED_FACE('',(#5341),#1457,.T.);
#33023=ADVANCED_FACE('',(#5342),#1458,.T.);
#33024=ADVANCED_FACE('',(#5343),#1459,.T.);
#33025=ADVANCED_FACE('',(#5344),#1460,.T.);
#33026=ADVANCED_FACE('',(#5345),#1461,.T.);
#33027=ADVANCED_FACE('',(#5346),#1462,.T.);
#33028=ADVANCED_FACE('',(#5347),#1463,.T.);
#33029=ADVANCED_FACE('',(#5348),#1464,.T.);
#33030=ADVANCED_FACE('',(#5349),#1465,.T.);
#33031=ADVANCED_FACE('',(#5350),#1466,.T.);
#33032=ADVANCED_FACE('',(#5351),#1467,.T.);
#33033=ADVANCED_FACE('',(#5352),#1468,.T.);
#33034=ADVANCED_FACE('',(#5353),#1469,.T.);
#33035=ADVANCED_FACE('',(#5354),#1470,.T.);
#33036=ADVANCED_FACE('',(#5355),#1471,.T.);
#33037=ADVANCED_FACE('',(#5356),#1472,.T.);
#33038=ADVANCED_FACE('',(#5357),#1473,.T.);
#33039=ADVANCED_FACE('',(#5358),#1474,.T.);
#33040=ADVANCED_FACE('',(#5359),#1475,.T.);
#33041=ADVANCED_FACE('',(#5360),#1476,.T.);
#33042=ADVANCED_FACE('',(#5361),#1477,.T.);
#33043=ADVANCED_FACE('',(#5362),#1478,.T.);
#33044=ADVANCED_FACE('',(#5363),#1479,.T.);
#33045=ADVANCED_FACE('',(#5364),#1480,.T.);
#33046=ADVANCED_FACE('',(#5365),#1481,.T.);
#33047=ADVANCED_FACE('',(#5366),#1482,.T.);
#33048=ADVANCED_FACE('',(#5367),#1483,.T.);
#33049=ADVANCED_FACE('',(#5368),#1484,.T.);
#33050=ADVANCED_FACE('',(#5369),#1485,.T.);
#33051=ADVANCED_FACE('',(#5370),#1486,.T.);
#33052=ADVANCED_FACE('',(#5371),#1487,.T.);
#33053=ADVANCED_FACE('',(#5372),#1488,.T.);
#33054=ADVANCED_FACE('',(#5373),#1489,.T.);
#33055=ADVANCED_FACE('',(#5374),#1490,.T.);
#33056=ADVANCED_FACE('',(#5375),#1491,.T.);
#33057=ADVANCED_FACE('',(#5376),#1492,.T.);
#33058=ADVANCED_FACE('',(#5377),#1493,.T.);
#33059=ADVANCED_FACE('',(#5378),#1494,.T.);
#33060=ADVANCED_FACE('',(#5379),#1495,.T.);
#33061=ADVANCED_FACE('',(#5380),#1496,.T.);
#33062=ADVANCED_FACE('',(#5381),#1497,.T.);
#33063=ADVANCED_FACE('',(#5382),#1498,.T.);
#33064=ADVANCED_FACE('',(#5383),#1499,.T.);
#33065=ADVANCED_FACE('',(#5384),#1500,.T.);
#33066=ADVANCED_FACE('',(#5385),#1501,.T.);
#33067=ADVANCED_FACE('',(#5386),#1502,.T.);
#33068=ADVANCED_FACE('',(#5387),#1503,.T.);
#33069=ADVANCED_FACE('',(#5388),#1504,.T.);
#33070=ADVANCED_FACE('',(#5389),#1505,.T.);
#33071=ADVANCED_FACE('',(#5390),#1506,.T.);
#33072=ADVANCED_FACE('',(#5391),#1507,.T.);
#33073=ADVANCED_FACE('',(#5392),#1508,.T.);
#33074=ADVANCED_FACE('',(#5393),#1509,.T.);
#33075=ADVANCED_FACE('',(#5394),#1510,.T.);
#33076=ADVANCED_FACE('',(#5395),#1511,.T.);
#33077=ADVANCED_FACE('',(#5396),#1512,.T.);
#33078=ADVANCED_FACE('',(#5397),#1513,.T.);
#33079=ADVANCED_FACE('',(#5398),#1514,.T.);
#33080=ADVANCED_FACE('',(#5399),#1515,.T.);
#33081=ADVANCED_FACE('',(#5400),#1516,.T.);
#33082=ADVANCED_FACE('',(#5401),#1517,.T.);
#33083=ADVANCED_FACE('',(#5402),#1518,.T.);
#33084=ADVANCED_FACE('',(#5403),#1519,.T.);
#33085=ADVANCED_FACE('',(#5404),#1520,.T.);
#33086=ADVANCED_FACE('',(#5405),#1521,.T.);
#33087=ADVANCED_FACE('',(#5406),#1522,.T.);
#33088=ADVANCED_FACE('',(#5407),#1523,.T.);
#33089=ADVANCED_FACE('',(#5408),#1524,.T.);
#33090=ADVANCED_FACE('',(#5409),#1525,.T.);
#33091=ADVANCED_FACE('',(#5410),#1526,.T.);
#33092=ADVANCED_FACE('',(#5411),#1527,.T.);
#33093=ADVANCED_FACE('',(#5412),#1528,.T.);
#33094=ADVANCED_FACE('',(#5413),#1529,.T.);
#33095=ADVANCED_FACE('',(#5414),#1530,.T.);
#33096=ADVANCED_FACE('',(#5415),#1531,.T.);
#33097=ADVANCED_FACE('',(#5416),#1532,.T.);
#33098=ADVANCED_FACE('',(#5417),#1533,.T.);
#33099=ADVANCED_FACE('',(#5418),#1534,.T.);
#33100=ADVANCED_FACE('',(#5419),#1535,.T.);
#33101=ADVANCED_FACE('',(#5420),#1536,.T.);
#33102=ADVANCED_FACE('',(#5421),#1537,.T.);
#33103=ADVANCED_FACE('',(#5422),#1538,.T.);
#33104=ADVANCED_FACE('',(#5423),#1539,.T.);
#33105=ADVANCED_FACE('',(#5424),#1540,.T.);
#33106=ADVANCED_FACE('',(#5425),#1541,.T.);
#33107=ADVANCED_FACE('',(#5426),#1542,.T.);
#33108=ADVANCED_FACE('',(#5427),#1543,.T.);
#33109=ADVANCED_FACE('',(#5428),#1544,.T.);
#33110=ADVANCED_FACE('',(#5429),#1545,.T.);
#33111=ADVANCED_FACE('',(#5430),#1546,.T.);
#33112=ADVANCED_FACE('',(#5431),#1547,.T.);
#33113=ADVANCED_FACE('',(#5432),#1548,.T.);
#33114=ADVANCED_FACE('',(#5433),#1549,.T.);
#33115=ADVANCED_FACE('',(#5434),#1550,.T.);
#33116=ADVANCED_FACE('',(#5435),#1551,.T.);
#33117=ADVANCED_FACE('',(#5436),#1552,.T.);
#33118=ADVANCED_FACE('',(#5437),#1553,.T.);
#33119=ADVANCED_FACE('',(#5438),#1554,.T.);
#33120=ADVANCED_FACE('',(#5439),#1555,.T.);
#33121=ADVANCED_FACE('',(#5440),#1556,.T.);
#33122=ADVANCED_FACE('',(#5441),#1557,.T.);
#33123=ADVANCED_FACE('',(#5442),#1558,.T.);
#33124=ADVANCED_FACE('',(#5443),#1559,.T.);
#33125=ADVANCED_FACE('',(#5444),#1560,.T.);
#33126=ADVANCED_FACE('',(#5445),#1561,.T.);
#33127=ADVANCED_FACE('',(#5446),#1562,.T.);
#33128=ADVANCED_FACE('',(#5447),#1563,.T.);
#33129=ADVANCED_FACE('',(#5448),#1564,.T.);
#33130=ADVANCED_FACE('',(#5449),#1565,.T.);
#33131=ADVANCED_FACE('',(#5450),#1566,.T.);
#33132=ADVANCED_FACE('',(#5451),#1567,.T.);
#33133=ADVANCED_FACE('',(#5452),#1568,.T.);
#33134=ADVANCED_FACE('',(#5453),#1569,.T.);
#33135=ADVANCED_FACE('',(#5454),#1570,.T.);
#33136=ADVANCED_FACE('',(#5455),#1571,.T.);
#33137=ADVANCED_FACE('',(#5456),#1572,.T.);
#33138=ADVANCED_FACE('',(#5457),#1573,.T.);
#33139=ADVANCED_FACE('',(#5458),#1574,.T.);
#33140=ADVANCED_FACE('',(#5459),#1575,.T.);
#33141=ADVANCED_FACE('',(#5460),#1576,.T.);
#33142=ADVANCED_FACE('',(#5461),#1577,.T.);
#33143=ADVANCED_FACE('',(#5462),#1578,.T.);
#33144=ADVANCED_FACE('',(#5463),#1579,.T.);
#33145=ADVANCED_FACE('',(#5464),#1580,.T.);
#33146=ADVANCED_FACE('',(#5465),#1581,.T.);
#33147=ADVANCED_FACE('',(#5466),#1582,.T.);
#33148=ADVANCED_FACE('',(#5467),#1583,.T.);
#33149=ADVANCED_FACE('',(#5468),#1584,.T.);
#33150=ADVANCED_FACE('',(#5469),#1585,.T.);
#33151=ADVANCED_FACE('',(#5470),#1586,.T.);
#33152=ADVANCED_FACE('',(#5471),#1587,.T.);
#33153=ADVANCED_FACE('',(#5472),#1588,.T.);
#33154=ADVANCED_FACE('',(#5473,#2133),#31662,.T.);
#33826=CLOSED_SHELL('',(#32953,#32954,#32955,#32956,#32957,#32958,#32959,
#32960,#32961,#32962,#32963,#32964,#32965,#32966,#32967,#32968,#32969,#32970,
#32971,#32972,#32973,#32974,#32975,#32976,#32977,#32978,#32979,#32980,#32981,
#32982,#32983,#32984,#32985,#32986,#32987,#32988,#32989,#32990,#32991,#32992,
#32993,#32994,#32995,#32996,#32997,#32998,#32999,#33000,#33001,#33002,#33003,
#33004,#33005,#33006,#33007,#33008,#33009,#33010,#33011,#33012,#33013,#33014,
#33015,#33016,#33017,#33018,#33019,#33020,#33021,#33022,#33023,#33024,#33025,
#33026,#33027,#33028,#33029,#33030,#33031,#33032,#33033,#33034,#33035,#33036,
#33037,#33038,#33039,#33040,#33041,#33042,#33043,#33044,#33045,#33046,#33047,
#33048,#33049,#33050,#33051,#33052,#33053,#33054,#33055,#33056,#33057,#33058,
#33059,#33060,#33061,#33062,#33063,#33064,#33065,#33066,#33067,#33068,#33069,
#33070,#33071,#33072,#33073,#33074,#33075,#33076,#33077,#33078,#33079,#33080,
#33081,#33082,#33083,#33084,#33085,#33086,#33087,#33088,#33089,#33090,#33091,
#33092,#33093,#33094,#33095,#33096,#33097,#33098,#33099,#33100,#33101,#33102,
#33103,#33104,#33105,#33106,#33107,#33108,#33109,#33110,#33111,#33112,#33113,
#33114,#33115,#33116,#33117,#33118,#33119,#33120,#33121,#33122,#33123,#33124,
#33125,#33126,#33127,#33128,#33129,#33130,#33131,#33132,#33133,#33134,#33135,
#33136,#33137,#33138,#33139,#33140,#33141,#33142,#33143,#33144,#33145,#33146,
#33147,#33148,#33149,#33150,#33151,#33152,#33153,#33154));
#36148=AXIS2_PLACEMENT_3D('',#56404,#43718,#43719);
#36149=AXIS2_PLACEMENT_3D('',#56405,#43720,#43721);
#36150=AXIS2_PLACEMENT_3D('',#56407,#43722,#43723);
#36151=AXIS2_PLACEMENT_3D('',#56409,#43724,#43725);
#36152=AXIS2_PLACEMENT_3D('',#56411,#43726,#43727);
#36153=AXIS2_PLACEMENT_3D('',#56412,#43728,#43729);
#36154=AXIS2_PLACEMENT_3D('',#56413,#43730,#43731);
#36155=AXIS2_PLACEMENT_3D('',#56416,#43733,#43734);
#36156=AXIS2_PLACEMENT_3D('',#56417,#43735,#43736);
#36157=AXIS2_PLACEMENT_3D('',#56425,#43740,#43741);
#36158=AXIS2_PLACEMENT_3D('',#56426,#43742,#43743);
#36159=AXIS2_PLACEMENT_3D('',#56428,#43744,#43745);
#36160=AXIS2_PLACEMENT_3D('',#56429,#43746,#43747);
#36161=AXIS2_PLACEMENT_3D('',#56430,#43748,#43749);
#36162=AXIS2_PLACEMENT_3D('',#56433,#43750,#43751);
#36163=AXIS2_PLACEMENT_3D('',#56435,#43752,#43753);
#36164=AXIS2_PLACEMENT_3D('',#56437,#43754,#43755);
#36165=AXIS2_PLACEMENT_3D('',#56439,#43756,#43757);
#36166=AXIS2_PLACEMENT_3D('',#56441,#43758,#43759);
#36167=AXIS2_PLACEMENT_3D('',#56443,#43760,#43761);
#36168=AXIS2_PLACEMENT_3D('',#56445,#43762,#43763);
#36169=AXIS2_PLACEMENT_3D('',#56447,#43764,#43765);
#36170=AXIS2_PLACEMENT_3D('',#56449,#43766,#43767);
#36171=AXIS2_PLACEMENT_3D('',#56451,#43768,#43769);
#36172=AXIS2_PLACEMENT_3D('',#56453,#43770,#43771);
#36173=AXIS2_PLACEMENT_3D('',#56455,#43772,#43773);
#36174=AXIS2_PLACEMENT_3D('',#56457,#43774,#43775);
#36175=AXIS2_PLACEMENT_3D('',#56459,#43776,#43777);
#36176=AXIS2_PLACEMENT_3D('',#56461,#43778,#43779);
#36177=AXIS2_PLACEMENT_3D('',#56463,#43780,#43781);
#36178=AXIS2_PLACEMENT_3D('',#56465,#43782,#43783);
#36179=AXIS2_PLACEMENT_3D('',#56467,#43784,#43785);
#36180=AXIS2_PLACEMENT_3D('',#56469,#43786,#43787);
#36181=AXIS2_PLACEMENT_3D('',#56471,#43788,#43789);
#36182=AXIS2_PLACEMENT_3D('',#56473,#43790,#43791);
#36183=AXIS2_PLACEMENT_3D('',#56475,#43792,#43793);
#36184=AXIS2_PLACEMENT_3D('',#56477,#43794,#43795);
#36185=AXIS2_PLACEMENT_3D('',#56479,#43796,#43797);
#36186=AXIS2_PLACEMENT_3D('',#56481,#43798,#43799);
#36187=AXIS2_PLACEMENT_3D('',#56483,#43800,#43801);
#36188=AXIS2_PLACEMENT_3D('',#56485,#43802,#43803);
#36189=AXIS2_PLACEMENT_3D('',#56487,#43804,#43805);
#36190=AXIS2_PLACEMENT_3D('',#56489,#43806,#43807);
#36191=AXIS2_PLACEMENT_3D('',#56491,#43808,#43809);
#36192=AXIS2_PLACEMENT_3D('',#56493,#43810,#43811);
#36193=AXIS2_PLACEMENT_3D('',#56495,#43812,#43813);
#36194=AXIS2_PLACEMENT_3D('',#56497,#43814,#43815);
#36195=AXIS2_PLACEMENT_3D('',#56499,#43816,#43817);
#36196=AXIS2_PLACEMENT_3D('',#56501,#43818,#43819);
#36197=AXIS2_PLACEMENT_3D('',#56503,#43820,#43821);
#36198=AXIS2_PLACEMENT_3D('',#56505,#43822,#43823);
#36199=AXIS2_PLACEMENT_3D('',#56507,#43824,#43825);
#36200=AXIS2_PLACEMENT_3D('',#56509,#43826,#43827);
#36201=AXIS2_PLACEMENT_3D('',#56511,#43828,#43829);
#36202=AXIS2_PLACEMENT_3D('',#56513,#43830,#43831);
#36203=AXIS2_PLACEMENT_3D('',#56515,#43832,#43833);
#36204=AXIS2_PLACEMENT_3D('',#56517,#43834,#43835);
#36205=AXIS2_PLACEMENT_3D('',#56519,#43836,#43837);
#36206=AXIS2_PLACEMENT_3D('',#56521,#43838,#43839);
#36207=AXIS2_PLACEMENT_3D('',#56523,#43840,#43841);
#36208=AXIS2_PLACEMENT_3D('',#56525,#43842,#43843);
#36209=AXIS2_PLACEMENT_3D('',#56527,#43844,#43845);
#36210=AXIS2_PLACEMENT_3D('',#56529,#43846,#43847);
#36211=AXIS2_PLACEMENT_3D('',#56531,#43848,#43849);
#36212=AXIS2_PLACEMENT_3D('',#56533,#43850,#43851);
#36213=AXIS2_PLACEMENT_3D('',#56535,#43852,#43853);
#36214=AXIS2_PLACEMENT_3D('',#56537,#43854,#43855);
#36215=AXIS2_PLACEMENT_3D('',#56539,#43856,#43857);
#36216=AXIS2_PLACEMENT_3D('',#56541,#43858,#43859);
#36217=AXIS2_PLACEMENT_3D('',#56543,#43860,#43861);
#36218=AXIS2_PLACEMENT_3D('',#56545,#43862,#43863);
#36219=AXIS2_PLACEMENT_3D('',#56547,#43864,#43865);
#36220=AXIS2_PLACEMENT_3D('',#56549,#43866,#43867);
#36221=AXIS2_PLACEMENT_3D('',#56551,#43868,#43869);
#36222=AXIS2_PLACEMENT_3D('',#56553,#43870,#43871);
#36223=AXIS2_PLACEMENT_3D('',#56555,#43872,#43873);
#36224=AXIS2_PLACEMENT_3D('',#56557,#43874,#43875);
#36225=AXIS2_PLACEMENT_3D('',#56559,#43876,#43877);
#36226=AXIS2_PLACEMENT_3D('',#56561,#43878,#43879);
#36227=AXIS2_PLACEMENT_3D('',#56563,#43880,#43881);
#36228=AXIS2_PLACEMENT_3D('',#56565,#43882,#43883);
#36229=AXIS2_PLACEMENT_3D('',#56567,#43884,#43885);
#36230=AXIS2_PLACEMENT_3D('',#56569,#43886,#43887);
#36231=AXIS2_PLACEMENT_3D('',#56571,#43888,#43889);
#36232=AXIS2_PLACEMENT_3D('',#56573,#43890,#43891);
#36233=AXIS2_PLACEMENT_3D('',#56575,#43892,#43893);
#36234=AXIS2_PLACEMENT_3D('',#56577,#43894,#43895);
#36235=AXIS2_PLACEMENT_3D('',#56579,#43896,#43897);
#36236=AXIS2_PLACEMENT_3D('',#56581,#43898,#43899);
#36237=AXIS2_PLACEMENT_3D('',#56583,#43900,#43901);
#36238=AXIS2_PLACEMENT_3D('',#56585,#43902,#43903);
#36239=AXIS2_PLACEMENT_3D('',#56587,#43904,#43905);
#36240=AXIS2_PLACEMENT_3D('',#56589,#43906,#43907);
#36241=AXIS2_PLACEMENT_3D('',#56591,#43908,#43909);
#36242=AXIS2_PLACEMENT_3D('',#56593,#43910,#43911);
#36243=AXIS2_PLACEMENT_3D('',#56595,#43912,#43913);
#36244=AXIS2_PLACEMENT_3D('',#56597,#43914,#43915);
#36245=AXIS2_PLACEMENT_3D('',#56599,#43916,#43917);
#36246=AXIS2_PLACEMENT_3D('',#56601,#43918,#43919);
#36247=AXIS2_PLACEMENT_3D('',#56603,#43920,#43921);
#36248=AXIS2_PLACEMENT_3D('',#56605,#43922,#43923);
#36249=AXIS2_PLACEMENT_3D('',#56607,#43924,#43925);
#36250=AXIS2_PLACEMENT_3D('',#56609,#43926,#43927);
#36251=AXIS2_PLACEMENT_3D('',#56611,#43928,#43929);
#36252=AXIS2_PLACEMENT_3D('',#56613,#43930,#43931);
#36253=AXIS2_PLACEMENT_3D('',#56615,#43932,#43933);
#36254=AXIS2_PLACEMENT_3D('',#56617,#43934,#43935);
#36255=AXIS2_PLACEMENT_3D('',#56619,#43936,#43937);
#36256=AXIS2_PLACEMENT_3D('',#56621,#43938,#43939);
#36257=AXIS2_PLACEMENT_3D('',#56623,#43940,#43941);
#36258=AXIS2_PLACEMENT_3D('',#56625,#43942,#43943);
#36259=AXIS2_PLACEMENT_3D('',#56627,#43944,#43945);
#36260=AXIS2_PLACEMENT_3D('',#56629,#43946,#43947);
#36261=AXIS2_PLACEMENT_3D('',#56631,#43948,#43949);
#36262=AXIS2_PLACEMENT_3D('',#56633,#43950,#43951);
#36263=AXIS2_PLACEMENT_3D('',#56635,#43952,#43953);
#36264=AXIS2_PLACEMENT_3D('',#56637,#43954,#43955);
#36265=AXIS2_PLACEMENT_3D('',#56639,#43956,#43957);
#36266=AXIS2_PLACEMENT_3D('',#56641,#43958,#43959);
#36267=AXIS2_PLACEMENT_3D('',#56643,#43960,#43961);
#36268=AXIS2_PLACEMENT_3D('',#56645,#43962,#43963);
#36269=AXIS2_PLACEMENT_3D('',#56647,#43964,#43965);
#36270=AXIS2_PLACEMENT_3D('',#56649,#43966,#43967);
#36271=AXIS2_PLACEMENT_3D('',#56651,#43968,#43969);
#36272=AXIS2_PLACEMENT_3D('',#56653,#43970,#43971);
#36273=AXIS2_PLACEMENT_3D('',#56655,#43972,#43973);
#36274=AXIS2_PLACEMENT_3D('',#56657,#43974,#43975);
#36275=AXIS2_PLACEMENT_3D('',#56659,#43976,#43977);
#36276=AXIS2_PLACEMENT_3D('',#56661,#43978,#43979);
#36277=AXIS2_PLACEMENT_3D('',#56663,#43980,#43981);
#36278=AXIS2_PLACEMENT_3D('',#56665,#43982,#43983);
#36279=AXIS2_PLACEMENT_3D('',#56667,#43984,#43985);
#36280=AXIS2_PLACEMENT_3D('',#56669,#43986,#43987);
#36281=AXIS2_PLACEMENT_3D('',#56671,#43988,#43989);
#36282=AXIS2_PLACEMENT_3D('',#56673,#43990,#43991);
#36283=AXIS2_PLACEMENT_3D('',#56675,#43992,#43993);
#36284=AXIS2_PLACEMENT_3D('',#56677,#43994,#43995);
#36285=AXIS2_PLACEMENT_3D('',#56679,#43996,#43997);
#36286=AXIS2_PLACEMENT_3D('',#56681,#43998,#43999);
#36287=AXIS2_PLACEMENT_3D('',#56683,#44000,#44001);
#36288=AXIS2_PLACEMENT_3D('',#56685,#44002,#44003);
#36289=AXIS2_PLACEMENT_3D('',#56687,#44004,#44005);
#36290=AXIS2_PLACEMENT_3D('',#56689,#44006,#44007);
#36291=AXIS2_PLACEMENT_3D('',#56691,#44008,#44009);
#36292=AXIS2_PLACEMENT_3D('',#56693,#44010,#44011);
#36293=AXIS2_PLACEMENT_3D('',#56695,#44012,#44013);
#36294=AXIS2_PLACEMENT_3D('',#56697,#44014,#44015);
#36295=AXIS2_PLACEMENT_3D('',#56699,#44016,#44017);
#36296=AXIS2_PLACEMENT_3D('',#56701,#44018,#44019);
#36297=AXIS2_PLACEMENT_3D('',#56703,#44020,#44021);
#36298=AXIS2_PLACEMENT_3D('',#56705,#44022,#44023);
#36299=AXIS2_PLACEMENT_3D('',#56707,#44024,#44025);
#36300=AXIS2_PLACEMENT_3D('',#56709,#44026,#44027);
#36301=AXIS2_PLACEMENT_3D('',#56711,#44028,#44029);
#36302=AXIS2_PLACEMENT_3D('',#56713,#44030,#44031);
#36303=AXIS2_PLACEMENT_3D('',#56715,#44032,#44033);
#36304=AXIS2_PLACEMENT_3D('',#56717,#44034,#44035);
#36305=AXIS2_PLACEMENT_3D('',#56719,#44036,#44037);
#36306=AXIS2_PLACEMENT_3D('',#56721,#44038,#44039);
#36307=AXIS2_PLACEMENT_3D('',#56723,#44040,#44041);
#36308=AXIS2_PLACEMENT_3D('',#56725,#44042,#44043);
#36309=AXIS2_PLACEMENT_3D('',#56727,#44044,#44045);
#36310=AXIS2_PLACEMENT_3D('',#56729,#44046,#44047);
#36311=AXIS2_PLACEMENT_3D('',#56731,#44048,#44049);
#36312=AXIS2_PLACEMENT_3D('',#56733,#44050,#44051);
#36313=AXIS2_PLACEMENT_3D('',#56735,#44052,#44053);
#36314=AXIS2_PLACEMENT_3D('',#56737,#44054,#44055);
#36315=AXIS2_PLACEMENT_3D('',#56739,#44056,#44057);
#36316=AXIS2_PLACEMENT_3D('',#56741,#44058,#44059);
#36317=AXIS2_PLACEMENT_3D('',#56743,#44060,#44061);
#36318=AXIS2_PLACEMENT_3D('',#56745,#44062,#44063);
#36319=AXIS2_PLACEMENT_3D('',#56747,#44064,#44065);
#36320=AXIS2_PLACEMENT_3D('',#56749,#44066,#44067);
#36321=AXIS2_PLACEMENT_3D('',#56751,#44068,#44069);
#36322=AXIS2_PLACEMENT_3D('',#56753,#44070,#44071);
#36323=AXIS2_PLACEMENT_3D('',#56755,#44072,#44073);
#36324=AXIS2_PLACEMENT_3D('',#56757,#44074,#44075);
#36325=AXIS2_PLACEMENT_3D('',#56759,#44076,#44077);
#36326=AXIS2_PLACEMENT_3D('',#56761,#44078,#44079);
#36327=AXIS2_PLACEMENT_3D('',#56763,#44080,#44081);
#36328=AXIS2_PLACEMENT_3D('',#56765,#44082,#44083);
#36329=AXIS2_PLACEMENT_3D('',#56767,#44084,#44085);
#36330=AXIS2_PLACEMENT_3D('',#56769,#44086,#44087);
#36331=AXIS2_PLACEMENT_3D('',#56771,#44088,#44089);
#36332=AXIS2_PLACEMENT_3D('',#56773,#44090,#44091);
#36333=AXIS2_PLACEMENT_3D('',#56775,#44092,#44093);
#36334=AXIS2_PLACEMENT_3D('',#56777,#44094,#44095);
#36335=AXIS2_PLACEMENT_3D('',#56779,#44096,#44097);
#36336=AXIS2_PLACEMENT_3D('',#56781,#44098,#44099);
#36337=AXIS2_PLACEMENT_3D('',#56783,#44100,#44101);
#36338=AXIS2_PLACEMENT_3D('',#56785,#44102,#44103);
#36339=AXIS2_PLACEMENT_3D('',#56787,#44104,#44105);
#36340=AXIS2_PLACEMENT_3D('',#56789,#44106,#44107);
#36341=AXIS2_PLACEMENT_3D('',#56791,#44108,#44109);
#36342=AXIS2_PLACEMENT_3D('',#56793,#44110,#44111);
#36343=AXIS2_PLACEMENT_3D('',#56795,#44112,#44113);
#36344=AXIS2_PLACEMENT_3D('',#56797,#44114,#44115);
#36345=AXIS2_PLACEMENT_3D('',#56799,#44116,#44117);
#36346=AXIS2_PLACEMENT_3D('',#56801,#44118,#44119);
#36347=AXIS2_PLACEMENT_3D('',#56803,#44120,#44121);
#36348=AXIS2_PLACEMENT_3D('',#56805,#44122,#44123);
#36349=AXIS2_PLACEMENT_3D('',#56807,#44124,#44125);
#36350=AXIS2_PLACEMENT_3D('',#56809,#44126,#44127);
#36351=AXIS2_PLACEMENT_3D('',#56811,#44128,#44129);
#36352=AXIS2_PLACEMENT_3D('',#56813,#44130,#44131);
#36353=AXIS2_PLACEMENT_3D('',#56814,#44132,#44133);
#36354=AXIS2_PLACEMENT_3D('',#56815,#44134,#44135);
#36355=AXIS2_PLACEMENT_3D('',#56821,#44139,#44140);
#36356=AXIS2_PLACEMENT_3D('',#56825,#44143,#44144);
#36357=AXIS2_PLACEMENT_3D('',#56827,#44145,#44146);
#36358=AXIS2_PLACEMENT_3D('',#56829,#44148,#44149);
#36359=AXIS2_PLACEMENT_3D('',#56831,#44151,#44152);
#36360=AXIS2_PLACEMENT_3D('',#56835,#44154,#44155);
#36361=AXIS2_PLACEMENT_3D('',#56837,#44157,#44158);
#36362=AXIS2_PLACEMENT_3D('',#56839,#44159,#44160);
#36363=AXIS2_PLACEMENT_3D('',#56841,#44162,#44163);
#36364=AXIS2_PLACEMENT_3D('',#56844,#44165,#44166);
#36365=AXIS2_PLACEMENT_3D('',#56845,#44167,#44168);
#36366=AXIS2_PLACEMENT_3D('',#56849,#44170,#44171);
#36367=AXIS2_PLACEMENT_3D('',#56851,#44173,#44174);
#36368=AXIS2_PLACEMENT_3D('',#56853,#44175,#44176);
#36369=AXIS2_PLACEMENT_3D('',#56855,#44178,#44179);
#36370=AXIS2_PLACEMENT_3D('',#56858,#44181,#44182);
#36371=AXIS2_PLACEMENT_3D('',#56859,#44183,#44184);
#36372=AXIS2_PLACEMENT_3D('',#56863,#44186,#44187);
#36373=AXIS2_PLACEMENT_3D('',#56865,#44189,#44190);
#36374=AXIS2_PLACEMENT_3D('',#56867,#44191,#44192);
#36375=AXIS2_PLACEMENT_3D('',#56869,#44194,#44195);
#36376=AXIS2_PLACEMENT_3D('',#56872,#44197,#44198);
#36377=AXIS2_PLACEMENT_3D('',#56873,#44199,#44200);
#36378=AXIS2_PLACEMENT_3D('',#56877,#44202,#44203);
#36379=AXIS2_PLACEMENT_3D('',#56879,#44205,#44206);
#36380=AXIS2_PLACEMENT_3D('',#56881,#44207,#44208);
#36381=AXIS2_PLACEMENT_3D('',#56883,#44210,#44211);
#36382=AXIS2_PLACEMENT_3D('',#56886,#44213,#44214);
#36383=AXIS2_PLACEMENT_3D('',#56887,#44215,#44216);
#36384=AXIS2_PLACEMENT_3D('',#56891,#44218,#44219);
#36385=AXIS2_PLACEMENT_3D('',#56893,#44221,#44222);
#36386=AXIS2_PLACEMENT_3D('',#56895,#44223,#44224);
#36387=AXIS2_PLACEMENT_3D('',#56897,#44226,#44227);
#36388=AXIS2_PLACEMENT_3D('',#56900,#44229,#44230);
#36389=AXIS2_PLACEMENT_3D('',#56901,#44231,#44232);
#36390=AXIS2_PLACEMENT_3D('',#56905,#44234,#44235);
#36391=AXIS2_PLACEMENT_3D('',#56907,#44237,#44238);
#36392=AXIS2_PLACEMENT_3D('',#56909,#44239,#44240);
#36393=AXIS2_PLACEMENT_3D('',#56911,#44242,#44243);
#36394=AXIS2_PLACEMENT_3D('',#56914,#44245,#44246);
#36395=AXIS2_PLACEMENT_3D('',#56915,#44247,#44248);
#36396=AXIS2_PLACEMENT_3D('',#56919,#44250,#44251);
#36397=AXIS2_PLACEMENT_3D('',#56921,#44253,#44254);
#36398=AXIS2_PLACEMENT_3D('',#56923,#44255,#44256);
#36399=AXIS2_PLACEMENT_3D('',#56925,#44258,#44259);
#36400=AXIS2_PLACEMENT_3D('',#56928,#44261,#44262);
#36401=AXIS2_PLACEMENT_3D('',#56929,#44263,#44264);
#36402=AXIS2_PLACEMENT_3D('',#56933,#44266,#44267);
#36403=AXIS2_PLACEMENT_3D('',#56935,#44269,#44270);
#36404=AXIS2_PLACEMENT_3D('',#56937,#44271,#44272);
#36405=AXIS2_PLACEMENT_3D('',#56939,#44274,#44275);
#36406=AXIS2_PLACEMENT_3D('',#56942,#44277,#44278);
#36407=AXIS2_PLACEMENT_3D('',#56943,#44279,#44280);
#36408=AXIS2_PLACEMENT_3D('',#56947,#44282,#44283);
#36409=AXIS2_PLACEMENT_3D('',#56949,#44285,#44286);
#36410=AXIS2_PLACEMENT_3D('',#56951,#44287,#44288);
#36411=AXIS2_PLACEMENT_3D('',#56953,#44290,#44291);
#36412=AXIS2_PLACEMENT_3D('',#56956,#44293,#44294);
#36413=AXIS2_PLACEMENT_3D('',#56957,#44295,#44296);
#36414=AXIS2_PLACEMENT_3D('',#56961,#44298,#44299);
#36415=AXIS2_PLACEMENT_3D('',#56963,#44301,#44302);
#36416=AXIS2_PLACEMENT_3D('',#56965,#44303,#44304);
#36417=AXIS2_PLACEMENT_3D('',#56967,#44306,#44307);
#36418=AXIS2_PLACEMENT_3D('',#56970,#44309,#44310);
#36419=AXIS2_PLACEMENT_3D('',#56971,#44311,#44312);
#36420=AXIS2_PLACEMENT_3D('',#56975,#44314,#44315);
#36421=AXIS2_PLACEMENT_3D('',#56977,#44317,#44318);
#36422=AXIS2_PLACEMENT_3D('',#56979,#44319,#44320);
#36423=AXIS2_PLACEMENT_3D('',#56981,#44322,#44323);
#36424=AXIS2_PLACEMENT_3D('',#56984,#44325,#44326);
#36425=AXIS2_PLACEMENT_3D('',#56985,#44327,#44328);
#36426=AXIS2_PLACEMENT_3D('',#56989,#44330,#44331);
#36427=AXIS2_PLACEMENT_3D('',#56991,#44333,#44334);
#36428=AXIS2_PLACEMENT_3D('',#56993,#44335,#44336);
#36429=AXIS2_PLACEMENT_3D('',#56995,#44338,#44339);
#36430=AXIS2_PLACEMENT_3D('',#56998,#44341,#44342);
#36431=AXIS2_PLACEMENT_3D('',#56999,#44343,#44344);
#36432=AXIS2_PLACEMENT_3D('',#57003,#44346,#44347);
#36433=AXIS2_PLACEMENT_3D('',#57005,#44349,#44350);
#36434=AXIS2_PLACEMENT_3D('',#57007,#44351,#44352);
#36435=AXIS2_PLACEMENT_3D('',#57009,#44354,#44355);
#36436=AXIS2_PLACEMENT_3D('',#57012,#44357,#44358);
#36437=AXIS2_PLACEMENT_3D('',#57013,#44359,#44360);
#36438=AXIS2_PLACEMENT_3D('',#57017,#44362,#44363);
#36439=AXIS2_PLACEMENT_3D('',#57019,#44365,#44366);
#36440=AXIS2_PLACEMENT_3D('',#57021,#44367,#44368);
#36441=AXIS2_PLACEMENT_3D('',#57023,#44370,#44371);
#36442=AXIS2_PLACEMENT_3D('',#57026,#44373,#44374);
#36443=AXIS2_PLACEMENT_3D('',#57027,#44375,#44376);
#36444=AXIS2_PLACEMENT_3D('',#57031,#44378,#44379);
#36445=AXIS2_PLACEMENT_3D('',#57033,#44381,#44382);
#36446=AXIS2_PLACEMENT_3D('',#57035,#44383,#44384);
#36447=AXIS2_PLACEMENT_3D('',#57037,#44386,#44387);
#36448=AXIS2_PLACEMENT_3D('',#57040,#44389,#44390);
#36449=AXIS2_PLACEMENT_3D('',#57041,#44391,#44392);
#36450=AXIS2_PLACEMENT_3D('',#57045,#44394,#44395);
#36451=AXIS2_PLACEMENT_3D('',#57047,#44397,#44398);
#36452=AXIS2_PLACEMENT_3D('',#57049,#44399,#44400);
#36453=AXIS2_PLACEMENT_3D('',#57051,#44402,#44403);
#36454=AXIS2_PLACEMENT_3D('',#57054,#44405,#44406);
#36455=AXIS2_PLACEMENT_3D('',#57055,#44407,#44408);
#36456=AXIS2_PLACEMENT_3D('',#57059,#44410,#44411);
#36457=AXIS2_PLACEMENT_3D('',#57061,#44413,#44414);
#36458=AXIS2_PLACEMENT_3D('',#57063,#44415,#44416);
#36459=AXIS2_PLACEMENT_3D('',#57065,#44418,#44419);
#36460=AXIS2_PLACEMENT_3D('',#57068,#44421,#44422);
#36461=AXIS2_PLACEMENT_3D('',#57069,#44423,#44424);
#36462=AXIS2_PLACEMENT_3D('',#57073,#44426,#44427);
#36463=AXIS2_PLACEMENT_3D('',#57075,#44429,#44430);
#36464=AXIS2_PLACEMENT_3D('',#57077,#44431,#44432);
#36465=AXIS2_PLACEMENT_3D('',#57079,#44434,#44435);
#36466=AXIS2_PLACEMENT_3D('',#57082,#44437,#44438);
#36467=AXIS2_PLACEMENT_3D('',#57083,#44439,#44440);
#36468=AXIS2_PLACEMENT_3D('',#57087,#44442,#44443);
#36469=AXIS2_PLACEMENT_3D('',#57089,#44445,#44446);
#36470=AXIS2_PLACEMENT_3D('',#57091,#44447,#44448);
#36471=AXIS2_PLACEMENT_3D('',#57093,#44450,#44451);
#36472=AXIS2_PLACEMENT_3D('',#57096,#44453,#44454);
#36473=AXIS2_PLACEMENT_3D('',#57097,#44455,#44456);
#36474=AXIS2_PLACEMENT_3D('',#57101,#44458,#44459);
#36475=AXIS2_PLACEMENT_3D('',#57103,#44461,#44462);
#36476=AXIS2_PLACEMENT_3D('',#57105,#44463,#44464);
#36477=AXIS2_PLACEMENT_3D('',#57107,#44466,#44467);
#36478=AXIS2_PLACEMENT_3D('',#57110,#44469,#44470);
#36479=AXIS2_PLACEMENT_3D('',#57111,#44471,#44472);
#36480=AXIS2_PLACEMENT_3D('',#57115,#44474,#44475);
#36481=AXIS2_PLACEMENT_3D('',#57117,#44477,#44478);
#36482=AXIS2_PLACEMENT_3D('',#57119,#44479,#44480);
#36483=AXIS2_PLACEMENT_3D('',#57121,#44482,#44483);
#36484=AXIS2_PLACEMENT_3D('',#57124,#44485,#44486);
#36485=AXIS2_PLACEMENT_3D('',#57125,#44487,#44488);
#36486=AXIS2_PLACEMENT_3D('',#57129,#44490,#44491);
#36487=AXIS2_PLACEMENT_3D('',#57131,#44493,#44494);
#36488=AXIS2_PLACEMENT_3D('',#57133,#44495,#44496);
#36489=AXIS2_PLACEMENT_3D('',#57135,#44498,#44499);
#36490=AXIS2_PLACEMENT_3D('',#57138,#44501,#44502);
#36491=AXIS2_PLACEMENT_3D('',#57139,#44503,#44504);
#36492=AXIS2_PLACEMENT_3D('',#57143,#44506,#44507);
#36493=AXIS2_PLACEMENT_3D('',#57145,#44509,#44510);
#36494=AXIS2_PLACEMENT_3D('',#57147,#44511,#44512);
#36495=AXIS2_PLACEMENT_3D('',#57149,#44514,#44515);
#36496=AXIS2_PLACEMENT_3D('',#57152,#44517,#44518);
#36497=AXIS2_PLACEMENT_3D('',#57153,#44519,#44520);
#36498=AXIS2_PLACEMENT_3D('',#57157,#44522,#44523);
#36499=AXIS2_PLACEMENT_3D('',#57159,#44525,#44526);
#36500=AXIS2_PLACEMENT_3D('',#57161,#44527,#44528);
#36501=AXIS2_PLACEMENT_3D('',#57163,#44530,#44531);
#36502=AXIS2_PLACEMENT_3D('',#57166,#44533,#44534);
#36503=AXIS2_PLACEMENT_3D('',#57167,#44535,#44536);
#36504=AXIS2_PLACEMENT_3D('',#57171,#44538,#44539);
#36505=AXIS2_PLACEMENT_3D('',#57173,#44541,#44542);
#36506=AXIS2_PLACEMENT_3D('',#57175,#44543,#44544);
#36507=AXIS2_PLACEMENT_3D('',#57177,#44546,#44547);
#36508=AXIS2_PLACEMENT_3D('',#57180,#44549,#44550);
#36509=AXIS2_PLACEMENT_3D('',#57181,#44551,#44552);
#36510=AXIS2_PLACEMENT_3D('',#57185,#44554,#44555);
#36511=AXIS2_PLACEMENT_3D('',#57187,#44557,#44558);
#36512=AXIS2_PLACEMENT_3D('',#57189,#44559,#44560);
#36513=AXIS2_PLACEMENT_3D('',#57191,#44562,#44563);
#36514=AXIS2_PLACEMENT_3D('',#57194,#44565,#44566);
#36515=AXIS2_PLACEMENT_3D('',#57195,#44567,#44568);
#36516=AXIS2_PLACEMENT_3D('',#57199,#44570,#44571);
#36517=AXIS2_PLACEMENT_3D('',#57201,#44573,#44574);
#36518=AXIS2_PLACEMENT_3D('',#57203,#44575,#44576);
#36519=AXIS2_PLACEMENT_3D('',#57205,#44578,#44579);
#36520=AXIS2_PLACEMENT_3D('',#57208,#44581,#44582);
#36521=AXIS2_PLACEMENT_3D('',#57209,#44583,#44584);
#36522=AXIS2_PLACEMENT_3D('',#57213,#44586,#44587);
#36523=AXIS2_PLACEMENT_3D('',#57215,#44589,#44590);
#36524=AXIS2_PLACEMENT_3D('',#57217,#44591,#44592);
#36525=AXIS2_PLACEMENT_3D('',#57219,#44594,#44595);
#36526=AXIS2_PLACEMENT_3D('',#57222,#44597,#44598);
#36527=AXIS2_PLACEMENT_3D('',#57223,#44599,#44600);
#36528=AXIS2_PLACEMENT_3D('',#57227,#44602,#44603);
#36529=AXIS2_PLACEMENT_3D('',#57229,#44605,#44606);
#36530=AXIS2_PLACEMENT_3D('',#57231,#44607,#44608);
#36531=AXIS2_PLACEMENT_3D('',#57233,#44610,#44611);
#36532=AXIS2_PLACEMENT_3D('',#57236,#44613,#44614);
#36533=AXIS2_PLACEMENT_3D('',#57237,#44615,#44616);
#36534=AXIS2_PLACEMENT_3D('',#57241,#44618,#44619);
#36535=AXIS2_PLACEMENT_3D('',#57243,#44621,#44622);
#36536=AXIS2_PLACEMENT_3D('',#57245,#44623,#44624);
#36537=AXIS2_PLACEMENT_3D('',#57247,#44626,#44627);
#36538=AXIS2_PLACEMENT_3D('',#57250,#44629,#44630);
#36539=AXIS2_PLACEMENT_3D('',#57251,#44631,#44632);
#36540=AXIS2_PLACEMENT_3D('',#57255,#44634,#44635);
#36541=AXIS2_PLACEMENT_3D('',#57257,#44637,#44638);
#36542=AXIS2_PLACEMENT_3D('',#57259,#44639,#44640);
#36543=AXIS2_PLACEMENT_3D('',#57261,#44642,#44643);
#36544=AXIS2_PLACEMENT_3D('',#57264,#44645,#44646);
#36545=AXIS2_PLACEMENT_3D('',#57265,#44647,#44648);
#36546=AXIS2_PLACEMENT_3D('',#57269,#44650,#44651);
#36547=AXIS2_PLACEMENT_3D('',#57271,#44653,#44654);
#36548=AXIS2_PLACEMENT_3D('',#57273,#44655,#44656);
#36549=AXIS2_PLACEMENT_3D('',#57275,#44658,#44659);
#36550=AXIS2_PLACEMENT_3D('',#57278,#44661,#44662);
#36551=AXIS2_PLACEMENT_3D('',#57279,#44663,#44664);
#36552=AXIS2_PLACEMENT_3D('',#57283,#44666,#44667);
#36553=AXIS2_PLACEMENT_3D('',#57285,#44669,#44670);
#36554=AXIS2_PLACEMENT_3D('',#57287,#44671,#44672);
#36555=AXIS2_PLACEMENT_3D('',#57289,#44674,#44675);
#36556=AXIS2_PLACEMENT_3D('',#57292,#44677,#44678);
#36557=AXIS2_PLACEMENT_3D('',#57293,#44679,#44680);
#36558=AXIS2_PLACEMENT_3D('',#57297,#44682,#44683);
#36559=AXIS2_PLACEMENT_3D('',#57299,#44685,#44686);
#36560=AXIS2_PLACEMENT_3D('',#57301,#44687,#44688);
#36561=AXIS2_PLACEMENT_3D('',#57303,#44690,#44691);
#36562=AXIS2_PLACEMENT_3D('',#57306,#44693,#44694);
#36563=AXIS2_PLACEMENT_3D('',#57307,#44695,#44696);
#36564=AXIS2_PLACEMENT_3D('',#57311,#44698,#44699);
#36565=AXIS2_PLACEMENT_3D('',#57313,#44701,#44702);
#36566=AXIS2_PLACEMENT_3D('',#57315,#44703,#44704);
#36567=AXIS2_PLACEMENT_3D('',#57317,#44706,#44707);
#36568=AXIS2_PLACEMENT_3D('',#57320,#44709,#44710);
#36569=AXIS2_PLACEMENT_3D('',#57321,#44711,#44712);
#36570=AXIS2_PLACEMENT_3D('',#57325,#44714,#44715);
#36571=AXIS2_PLACEMENT_3D('',#57327,#44717,#44718);
#36572=AXIS2_PLACEMENT_3D('',#57329,#44719,#44720);
#36573=AXIS2_PLACEMENT_3D('',#57331,#44722,#44723);
#36574=AXIS2_PLACEMENT_3D('',#57334,#44725,#44726);
#36575=AXIS2_PLACEMENT_3D('',#57335,#44727,#44728);
#36576=AXIS2_PLACEMENT_3D('',#57339,#44730,#44731);
#36577=AXIS2_PLACEMENT_3D('',#57341,#44733,#44734);
#36578=AXIS2_PLACEMENT_3D('',#57343,#44735,#44736);
#36579=AXIS2_PLACEMENT_3D('',#57345,#44738,#44739);
#36580=AXIS2_PLACEMENT_3D('',#57348,#44741,#44742);
#36581=AXIS2_PLACEMENT_3D('',#57349,#44743,#44744);
#36582=AXIS2_PLACEMENT_3D('',#57353,#44746,#44747);
#36583=AXIS2_PLACEMENT_3D('',#57355,#44749,#44750);
#36584=AXIS2_PLACEMENT_3D('',#57357,#44751,#44752);
#36585=AXIS2_PLACEMENT_3D('',#57359,#44754,#44755);
#36586=AXIS2_PLACEMENT_3D('',#57362,#44757,#44758);
#36587=AXIS2_PLACEMENT_3D('',#57363,#44759,#44760);
#36588=AXIS2_PLACEMENT_3D('',#57367,#44762,#44763);
#36589=AXIS2_PLACEMENT_3D('',#57369,#44765,#44766);
#36590=AXIS2_PLACEMENT_3D('',#57371,#44767,#44768);
#36591=AXIS2_PLACEMENT_3D('',#57373,#44770,#44771);
#36592=AXIS2_PLACEMENT_3D('',#57376,#44773,#44774);
#36593=AXIS2_PLACEMENT_3D('',#57377,#44775,#44776);
#36594=AXIS2_PLACEMENT_3D('',#57381,#44778,#44779);
#36595=AXIS2_PLACEMENT_3D('',#57383,#44781,#44782);
#36596=AXIS2_PLACEMENT_3D('',#57385,#44783,#44784);
#36597=AXIS2_PLACEMENT_3D('',#57387,#44786,#44787);
#36598=AXIS2_PLACEMENT_3D('',#57390,#44789,#44790);
#36599=AXIS2_PLACEMENT_3D('',#57391,#44791,#44792);
#36600=AXIS2_PLACEMENT_3D('',#57395,#44794,#44795);
#36601=AXIS2_PLACEMENT_3D('',#57397,#44797,#44798);
#36602=AXIS2_PLACEMENT_3D('',#57399,#44799,#44800);
#36603=AXIS2_PLACEMENT_3D('',#57401,#44802,#44803);
#36604=AXIS2_PLACEMENT_3D('',#57404,#44805,#44806);
#36605=AXIS2_PLACEMENT_3D('',#57405,#44807,#44808);
#36606=AXIS2_PLACEMENT_3D('',#57409,#44810,#44811);
#36607=AXIS2_PLACEMENT_3D('',#57411,#44813,#44814);
#36608=AXIS2_PLACEMENT_3D('',#57413,#44815,#44816);
#36609=AXIS2_PLACEMENT_3D('',#57415,#44818,#44819);
#36610=AXIS2_PLACEMENT_3D('',#57418,#44821,#44822);
#36611=AXIS2_PLACEMENT_3D('',#57419,#44823,#44824);
#36612=AXIS2_PLACEMENT_3D('',#57423,#44826,#44827);
#36613=AXIS2_PLACEMENT_3D('',#57425,#44829,#44830);
#36614=AXIS2_PLACEMENT_3D('',#57427,#44831,#44832);
#36615=AXIS2_PLACEMENT_3D('',#57429,#44834,#44835);
#36616=AXIS2_PLACEMENT_3D('',#57432,#44837,#44838);
#36617=AXIS2_PLACEMENT_3D('',#57433,#44839,#44840);
#36618=AXIS2_PLACEMENT_3D('',#57437,#44842,#44843);
#36619=AXIS2_PLACEMENT_3D('',#57439,#44845,#44846);
#36620=AXIS2_PLACEMENT_3D('',#57441,#44847,#44848);
#36621=AXIS2_PLACEMENT_3D('',#57443,#44850,#44851);
#36622=AXIS2_PLACEMENT_3D('',#57446,#44853,#44854);
#36623=AXIS2_PLACEMENT_3D('',#57447,#44855,#44856);
#36624=AXIS2_PLACEMENT_3D('',#57451,#44858,#44859);
#36625=AXIS2_PLACEMENT_3D('',#57453,#44861,#44862);
#36626=AXIS2_PLACEMENT_3D('',#57455,#44863,#44864);
#36627=AXIS2_PLACEMENT_3D('',#57457,#44866,#44867);
#36628=AXIS2_PLACEMENT_3D('',#57460,#44869,#44870);
#36629=AXIS2_PLACEMENT_3D('',#57461,#44871,#44872);
#36630=AXIS2_PLACEMENT_3D('',#57465,#44874,#44875);
#36631=AXIS2_PLACEMENT_3D('',#57467,#44877,#44878);
#36632=AXIS2_PLACEMENT_3D('',#57469,#44879,#44880);
#36633=AXIS2_PLACEMENT_3D('',#57471,#44882,#44883);
#36634=AXIS2_PLACEMENT_3D('',#57474,#44885,#44886);
#36635=AXIS2_PLACEMENT_3D('',#57475,#44887,#44888);
#36636=AXIS2_PLACEMENT_3D('',#57479,#44890,#44891);
#36637=AXIS2_PLACEMENT_3D('',#57481,#44893,#44894);
#36638=AXIS2_PLACEMENT_3D('',#57483,#44895,#44896);
#36639=AXIS2_PLACEMENT_3D('',#57485,#44898,#44899);
#36640=AXIS2_PLACEMENT_3D('',#57488,#44901,#44902);
#36641=AXIS2_PLACEMENT_3D('',#57489,#44903,#44904);
#36642=AXIS2_PLACEMENT_3D('',#57491,#44905,#44906);
#36643=AXIS2_PLACEMENT_3D('',#57493,#44908,#44909);
#36644=AXIS2_PLACEMENT_3D('',#57494,#44910,#44911);
#36645=AXIS2_PLACEMENT_3D('',#57495,#44912,#44913);
#36646=AXIS2_PLACEMENT_3D('',#57496,#44914,#44915);
#36647=AXIS2_PLACEMENT_3D('',#57497,#44916,#44917);
#36648=AXIS2_PLACEMENT_3D('',#57498,#44918,#44919);
#36649=AXIS2_PLACEMENT_3D('',#57499,#44920,#44921);
#36650=AXIS2_PLACEMENT_3D('',#57500,#44922,#44923);
#36651=AXIS2_PLACEMENT_3D('',#57501,#44924,#44925);
#36652=AXIS2_PLACEMENT_3D('',#57502,#44926,#44927);
#36653=AXIS2_PLACEMENT_3D('',#57503,#44928,#44929);
#36654=AXIS2_PLACEMENT_3D('',#57504,#44930,#44931);
#36655=AXIS2_PLACEMENT_3D('',#57505,#44932,#44933);
#36656=AXIS2_PLACEMENT_3D('',#57506,#44934,#44935);
#36657=AXIS2_PLACEMENT_3D('',#57507,#44936,#44937);
#36658=AXIS2_PLACEMENT_3D('',#57508,#44938,#44939);
#36659=AXIS2_PLACEMENT_3D('',#57509,#44940,#44941);
#36660=AXIS2_PLACEMENT_3D('',#57510,#44942,#44943);
#36661=AXIS2_PLACEMENT_3D('',#57511,#44944,#44945);
#36662=AXIS2_PLACEMENT_3D('',#57512,#44946,#44947);
#36663=AXIS2_PLACEMENT_3D('',#57513,#44948,#44949);
#36664=AXIS2_PLACEMENT_3D('',#57514,#44950,#44951);
#36665=AXIS2_PLACEMENT_3D('',#57515,#44952,#44953);
#36666=AXIS2_PLACEMENT_3D('',#57516,#44954,#44955);
#36667=AXIS2_PLACEMENT_3D('',#57517,#44956,#44957);
#36668=AXIS2_PLACEMENT_3D('',#57518,#44958,#44959);
#36669=AXIS2_PLACEMENT_3D('',#57519,#44960,#44961);
#36670=AXIS2_PLACEMENT_3D('',#57520,#44962,#44963);
#36671=AXIS2_PLACEMENT_3D('',#57521,#44964,#44965);
#36672=AXIS2_PLACEMENT_3D('',#57522,#44966,#44967);
#36673=AXIS2_PLACEMENT_3D('',#57523,#44968,#44969);
#36674=AXIS2_PLACEMENT_3D('',#57524,#44970,#44971);
#36675=AXIS2_PLACEMENT_3D('',#57525,#44972,#44973);
#36676=AXIS2_PLACEMENT_3D('',#57526,#44974,#44975);
#36677=AXIS2_PLACEMENT_3D('',#57527,#44976,#44977);
#36678=AXIS2_PLACEMENT_3D('',#57528,#44978,#44979);
#36679=AXIS2_PLACEMENT_3D('',#57529,#44980,#44981);
#36680=AXIS2_PLACEMENT_3D('',#57530,#44982,#44983);
#36681=AXIS2_PLACEMENT_3D('',#57531,#44984,#44985);
#36682=AXIS2_PLACEMENT_3D('',#57532,#44986,#44987);
#36683=AXIS2_PLACEMENT_3D('',#57533,#44988,#44989);
#36684=AXIS2_PLACEMENT_3D('',#57534,#44990,#44991);
#36685=AXIS2_PLACEMENT_3D('',#57535,#44992,#44993);
#36686=AXIS2_PLACEMENT_3D('',#57536,#44994,#44995);
#36687=AXIS2_PLACEMENT_3D('',#57537,#44996,#44997);
#36688=AXIS2_PLACEMENT_3D('',#57538,#44998,#44999);
#36689=AXIS2_PLACEMENT_3D('',#57539,#45000,#45001);
#36690=AXIS2_PLACEMENT_3D('',#57540,#45002,#45003);
#36691=AXIS2_PLACEMENT_3D('',#57541,#45004,#45005);
#36692=AXIS2_PLACEMENT_3D('',#57542,#45006,#45007);
#36693=AXIS2_PLACEMENT_3D('',#57543,#45008,#45009);
#36694=AXIS2_PLACEMENT_3D('',#57544,#45010,#45011);
#36695=AXIS2_PLACEMENT_3D('',#57545,#45012,#45013);
#36696=AXIS2_PLACEMENT_3D('',#57546,#45014,#45015);
#36697=AXIS2_PLACEMENT_3D('',#57547,#45016,#45017);
#36698=AXIS2_PLACEMENT_3D('',#57548,#45018,#45019);
#36699=AXIS2_PLACEMENT_3D('',#57549,#45020,#45021);
#36700=AXIS2_PLACEMENT_3D('',#57550,#45022,#45023);
#36701=AXIS2_PLACEMENT_3D('',#57551,#45024,#45025);
#36702=AXIS2_PLACEMENT_3D('',#57552,#45026,#45027);
#36703=AXIS2_PLACEMENT_3D('',#57553,#45028,#45029);
#36704=AXIS2_PLACEMENT_3D('',#57554,#45030,#45031);
#36705=AXIS2_PLACEMENT_3D('',#57555,#45032,#45033);
#36706=AXIS2_PLACEMENT_3D('',#57556,#45034,#45035);
#36707=AXIS2_PLACEMENT_3D('',#57557,#45036,#45037);
#36708=AXIS2_PLACEMENT_3D('',#57558,#45038,#45039);
#36709=AXIS2_PLACEMENT_3D('',#57559,#45040,#45041);
#36710=AXIS2_PLACEMENT_3D('',#57560,#45042,#45043);
#36711=AXIS2_PLACEMENT_3D('',#57561,#45044,#45045);
#36712=AXIS2_PLACEMENT_3D('',#57562,#45046,#45047);
#36713=AXIS2_PLACEMENT_3D('',#57563,#45048,#45049);
#36714=AXIS2_PLACEMENT_3D('',#57564,#45050,#45051);
#36715=AXIS2_PLACEMENT_3D('',#57565,#45052,#45053);
#36716=AXIS2_PLACEMENT_3D('',#57566,#45054,#45055);
#36717=AXIS2_PLACEMENT_3D('',#57567,#45056,#45057);
#36718=AXIS2_PLACEMENT_3D('',#57568,#45058,#45059);
#36719=AXIS2_PLACEMENT_3D('',#57569,#45060,#45061);
#36720=AXIS2_PLACEMENT_3D('',#57570,#45062,#45063);
#36721=AXIS2_PLACEMENT_3D('',#57571,#45064,#45065);
#36722=AXIS2_PLACEMENT_3D('',#57572,#45066,#45067);
#36723=AXIS2_PLACEMENT_3D('',#57573,#45068,#45069);
#36724=AXIS2_PLACEMENT_3D('',#57574,#45070,#45071);
#36725=AXIS2_PLACEMENT_3D('',#57575,#45072,#45073);
#36726=AXIS2_PLACEMENT_3D('',#57576,#45074,#45075);
#36727=AXIS2_PLACEMENT_3D('',#57577,#45076,#45077);
#36728=AXIS2_PLACEMENT_3D('',#57578,#45078,#45079);
#36729=AXIS2_PLACEMENT_3D('',#57579,#45080,#45081);
#36730=AXIS2_PLACEMENT_3D('',#57580,#45082,#45083);
#36731=AXIS2_PLACEMENT_3D('',#57581,#45084,#45085);
#36732=AXIS2_PLACEMENT_3D('',#57582,#45086,#45087);
#36733=AXIS2_PLACEMENT_3D('',#57583,#45088,#45089);
#36734=AXIS2_PLACEMENT_3D('',#57584,#45090,#45091);
#36735=AXIS2_PLACEMENT_3D('',#57585,#45092,#45093);
#36736=AXIS2_PLACEMENT_3D('',#57589,#45095,#45096);
#36737=AXIS2_PLACEMENT_3D('',#57591,#45098,#45099);
#36738=AXIS2_PLACEMENT_3D('',#57593,#45100,#45101);
#36739=AXIS2_PLACEMENT_3D('',#57595,#45103,#45104);
#36740=AXIS2_PLACEMENT_3D('',#57596,#45105,#45106);
#36741=AXIS2_PLACEMENT_3D('',#57597,#45107,#45108);
#36742=AXIS2_PLACEMENT_3D('',#57598,#45109,#45110);
#36743=AXIS2_PLACEMENT_3D('',#57599,#45111,#45112);
#43718=DIRECTION('axis',(0.,0.,1.));
#43719=DIRECTION('refdir',(1.,0.,0.));
#43720=DIRECTION('center_axis',(3.66113466765132E-16,1.,1.12027918221652E-15));
#43721=DIRECTION('ref_axis',(-5.6843418860808E-15,1.12502599828683E-15,
-1.));
#43722=DIRECTION('center_axis',(-3.66113466765132E-16,-1.,-1.12027918221652E-15));
#43723=DIRECTION('ref_axis',(5.46077161851015E-15,-1.12027918221652E-15,
1.));
#43724=DIRECTION('center_axis',(1.,-3.66113466765125E-16,-5.9211894646675E-15));
#43725=DIRECTION('ref_axis',(5.9211894646675E-15,-1.11022302462516E-15,
1.));
#43726=DIRECTION('center_axis',(3.66113466765132E-16,1.,1.12027918221652E-15));
#43727=DIRECTION('ref_axis',(5.46077161851015E-15,-1.12027918221652E-15,
1.));
#43728=DIRECTION('center_axis',(3.66113466765132E-16,1.,1.12027918221652E-15));
#43729=DIRECTION('ref_axis',(5.46077161851015E-15,-1.12027918221652E-15,
1.));
#43730=DIRECTION('center_axis',(3.66113466765132E-16,1.,1.12027918221652E-15));
#43731=DIRECTION('ref_axis',(5.46077161851015E-15,-1.12027918221652E-15,
1.));
#43732=DIRECTION('',(-3.66113466765132E-16,-1.,-1.12027918221652E-15));
#43733=DIRECTION('center_axis',(-3.66113466765132E-16,-1.,-1.12027918221652E-15));
#43734=DIRECTION('ref_axis',(5.46077161851015E-15,-1.12027918221652E-15,
1.));
#43735=DIRECTION('center_axis',(3.66113466765132E-16,1.,1.12027918221652E-15));
#43736=DIRECTION('ref_axis',(-5.46077161851015E-15,1.12027918221652E-15,
-1.));
#43737=DIRECTION('',(1.,-3.66113466765126E-16,-5.46077161851015E-15));
#43738=DIRECTION('',(5.46077161851015E-15,-1.12027918221652E-15,1.));
#43739=DIRECTION('',(-1.,3.66113466765126E-16,5.46077161851015E-15));
#43740=DIRECTION('center_axis',(-3.66113466765132E-16,-1.,-1.12027918221652E-15));
#43741=DIRECTION('ref_axis',(-0.916515138991166,-1.12563138007831E-16,0.400000000000005));
#43742=DIRECTION('center_axis',(-3.66113466765132E-16,-1.,-1.12027918221652E-15));
#43743=DIRECTION('ref_axis',(5.015595781836E-15,-1.12328447197369E-15,1.));
#43744=DIRECTION('center_axis',(3.66113466765132E-16,1.,1.12027918221652E-15));
#43745=DIRECTION('ref_axis',(5.46077161851015E-15,-1.12027918221652E-15,
1.));
#43746=DIRECTION('center_axis',(-1.,3.66113466765126E-16,5.2245789394125E-15));
#43747=DIRECTION('ref_axis',(-5.2245789394125E-15,1.12654983381082E-15,
-1.));
#43748=DIRECTION('center_axis',(-3.66113466765132E-16,-1.,-1.12027918221652E-15));
#43749=DIRECTION('ref_axis',(5.46077161851015E-15,-1.12027918221652E-15,
1.));
#43750=DIRECTION('center_axis',(3.66113466765132E-16,1.,1.12027918221652E-15));
#43751=DIRECTION('ref_axis',(-0.0850481328578615,-1.08508296912223E-15,
0.996376843918701));
#43752=DIRECTION('center_axis',(3.66113466765132E-16,1.,1.12027918221652E-15));
#43753=DIRECTION('ref_axis',(-0.97746197494357,1.21358115044514E-16,0.211111552358972));
#43754=DIRECTION('center_axis',(3.66113466765132E-16,1.,1.12027918221652E-15));
#43755=DIRECTION('ref_axis',(-0.632741728117551,1.09915790732807E-15,-0.774362902971737));
#43756=DIRECTION('center_axis',(-3.66113466765132E-16,-1.,-1.12027918221652E-15));
#43757=DIRECTION('ref_axis',(5.46077161851015E-15,-1.12027918221652E-15,
1.));
#43758=DIRECTION('center_axis',(3.66113466765132E-16,1.,1.12027918221652E-15));
#43759=DIRECTION('ref_axis',(0.0457327411615766,-1.13585041865483E-15,0.998953710832413));
#43760=DIRECTION('center_axis',(3.66113466765132E-16,1.,1.12027918221652E-15));
#43761=DIRECTION('ref_axis',(-0.941544065183018,-3.26987276389964E-17,0.336889853392226));
#43762=DIRECTION('center_axis',(3.66113466765132E-16,1.,1.12027918221652E-15));
#43763=DIRECTION('ref_axis',(-0.728403176040296,1.03423609619734E-15,-0.685148752559916));
#43764=DIRECTION('center_axis',(-3.66113466765132E-16,-1.,-1.12027918221652E-15));
#43765=DIRECTION('ref_axis',(5.46077161851015E-15,-1.12027918221652E-15,
1.));
#43766=DIRECTION('center_axis',(3.66113466765132E-16,1.,1.12027918221652E-15));
#43767=DIRECTION('ref_axis',(0.175731115300229,-1.16718315260702E-15,0.984438202791489));
#43768=DIRECTION('center_axis',(3.66113466765132E-16,1.,1.12027918221652E-15));
#43769=DIRECTION('ref_axis',(-0.889516075421853,-1.86196086026804E-16,0.456903875630427));
#43770=DIRECTION('center_axis',(3.66113466765132E-16,1.,1.12027918221652E-15));
#43771=DIRECTION('ref_axis',(-0.811601443669479,9.51618218716255E-16,-0.584211517032673));
#43772=DIRECTION('center_axis',(-3.66113466765132E-16,-1.,-1.12027918221652E-15));
#43773=DIRECTION('ref_axis',(5.46077161851015E-15,-1.12027918221652E-15,
1.));
#43774=DIRECTION('center_axis',(3.66113466765132E-16,1.,1.12027918221652E-15));
#43775=DIRECTION('ref_axis',(0.302722681334224,-1.1785450592138E-15,0.95307868416297));
#43776=DIRECTION('center_axis',(3.66113466765132E-16,1.,1.12027918221652E-15));
#43777=DIRECTION('ref_axis',(-0.822268218989772,-3.36507577759385E-16,0.569100145878903));
#43778=DIRECTION('center_axis',(3.66113466765132E-16,1.,1.12027918221652E-15));
#43779=DIRECTION('ref_axis',(-0.880912985579045,8.52717889674523E-16,-0.473278260474969));
#43780=DIRECTION('center_axis',(-3.66113466765132E-16,-1.,-1.12027918221652E-15));
#43781=DIRECTION('ref_axis',(5.46077161851015E-15,-1.12027918221652E-15,
1.));
#43782=DIRECTION('center_axis',(3.66113466765132E-16,1.,1.12027918221652E-15));
#43783=DIRECTION('ref_axis',(0.424534578360008,-1.16974173310301E-15,0.905411725005089));
#43784=DIRECTION('center_axis',(3.66113466765132E-16,1.,1.12027918221652E-15));
#43785=DIRECTION('ref_axis',(-0.740951125354955,-4.81061331538975E-16,0.671558954847023));
#43786=DIRECTION('center_axis',(3.66113466765132E-16,1.,1.12027918221652E-15));
#43787=DIRECTION('ref_axis',(-0.935151862070134,7.39227321122395E-16,-0.354247081663014));
#43788=DIRECTION('center_axis',(-3.66113466765132E-16,-1.,-1.12027918221652E-15));
#43789=DIRECTION('ref_axis',(5.46077161851015E-15,-1.12027918221652E-15,
1.));
#43790=DIRECTION('center_axis',(3.66113466765132E-16,1.,1.12027918221652E-15));
#43791=DIRECTION('ref_axis',(0.53908257104683,-1.14092380162514E-15,0.842252920204816));
#43792=DIRECTION('center_axis',(3.66113466765132E-16,1.,1.12027918221652E-15));
#43793=DIRECTION('ref_axis',(-0.646956152534853,-6.17383992560537E-16,0.762527203906392));
#43794=DIRECTION('center_axis',(3.66113466765132E-16,1.,1.12027918221652E-15));
#43795=DIRECTION('ref_axis',(-0.973390030928123,6.13088368153331E-16,-0.229154637067959));
#43796=DIRECTION('center_axis',(-3.66113466765132E-16,-1.,-1.12027918221652E-15));
#43797=DIRECTION('ref_axis',(5.46077161851015E-15,-1.12027918221652E-15,
1.));
#43798=DIRECTION('center_axis',(3.66113466765132E-16,1.,1.12027918221652E-15));
#43799=DIRECTION('ref_axis',(0.644406711481115,-1.09258434757764E-15,0.764682934423213));
#43800=DIRECTION('center_axis',(3.66113466765132E-16,1.,1.12027918221652E-15));
#43801=DIRECTION('ref_axis',(-0.541891580574746,-7.43143042298206E-16,0.840448401094442));
#43802=DIRECTION('center_axis',(3.66113466765132E-16,1.,1.12027918221652E-15));
#43803=DIRECTION('ref_axis',(-0.994973226482231,4.76459303224952E-16,-0.100141293099001));
#43804=DIRECTION('center_axis',(-3.66113466765132E-16,-1.,-1.12027918221652E-15));
#43805=DIRECTION('ref_axis',(5.46077161851015E-15,-1.12027918221652E-15,
1.));
#43806=DIRECTION('center_axis',(3.66113466765132E-16,1.,1.12027918221652E-15));
#43807=DIRECTION('ref_axis',(0.738704874418665,-1.02555047242146E-15,0.674029011623465));
#43808=DIRECTION('center_axis',(3.66113466765132E-16,1.,1.12027918221652E-15));
#43809=DIRECTION('ref_axis',(-0.427555093430276,-8.56186708543976E-16,0.903989293123446));
#43810=DIRECTION('center_axis',(3.66113466765132E-16,1.,1.12027918221652E-15));
#43811=DIRECTION('ref_axis',(-0.999532154272533,3.3167788751892E-16,0.0305854961592914));
#43812=DIRECTION('center_axis',(-3.66113466765132E-16,-1.,-1.12027918221652E-15));
#43813=DIRECTION('ref_axis',(5.46077161851015E-15,-1.12027918221652E-15,
1.));
#43814=DIRECTION('center_axis',(3.66113466765132E-16,1.,1.12027918221652E-15));
#43815=DIRECTION('ref_axis',(0.820363592147227,-9.40969144345853E-16,0.571842265558692));
#43816=DIRECTION('center_axis',(3.66113466765132E-16,1.,1.12027918221652E-15));
#43817=DIRECTION('ref_axis',(-0.305903020096547,-9.54580782826758E-16,0.952062677713926));
#43818=DIRECTION('center_axis',(3.66113466765132E-16,1.,1.12027918221652E-15));
#43819=DIRECTION('ref_axis',(-0.986988809780564,1.81221371198957E-16,0.160788959098396));
#43820=DIRECTION('center_axis',(-3.66113466765132E-16,-1.,-1.12027918221652E-15));
#43821=DIRECTION('ref_axis',(5.46077161851015E-15,-1.12027918221652E-15,
1.));
#43822=DIRECTION('center_axis',(3.66113466765132E-16,1.,1.12027918221652E-15));
#43823=DIRECTION('ref_axis',(0.887985661366392,-8.40287573324551E-16,0.459871139785583));
#43824=DIRECTION('center_axis',(3.66113466765132E-16,1.,1.12027918221652E-15));
#43825=DIRECTION('ref_axis',(-0.179016861276626,-1.03664171525558E-15,0.983846005927078));
#43826=DIRECTION('center_axis',(3.66113466765132E-16,1.,1.12027918221652E-15));
#43827=DIRECTION('ref_axis',(-0.957557813108254,2.76641069737215E-17,0.288241278368207));
#43828=DIRECTION('center_axis',(-3.66113466765132E-16,-1.,-1.12027918221652E-15));
#43829=DIRECTION('ref_axis',(5.46077161851015E-15,-1.12027918221652E-15,
1.));
#43830=DIRECTION('center_axis',(3.66113466765132E-16,1.,1.12027918221652E-15));
#43831=DIRECTION('ref_axis',(0.940414049723441,-7.25228448951937E-16,0.340031491310375));
#43832=DIRECTION('center_axis',(3.66113466765132E-16,1.,1.12027918221652E-15));
#43833=DIRECTION('ref_axis',(-0.0490676743274118,-1.100965420525E-15,0.998795456205173));
#43834=DIRECTION('center_axis',(3.66113466765132E-16,1.,1.12027918221652E-15));
#43835=DIRECTION('ref_axis',(-0.91174273676848,-1.26366497791772E-16,0.410761709449557));
#43836=DIRECTION('center_axis',(-3.66113466765132E-16,-1.,-1.12027918221652E-15));
#43837=DIRECTION('ref_axis',(5.46077161851015E-15,-1.12027918221652E-15,
1.));
#43838=DIRECTION('center_axis',(3.66113466765132E-16,1.,1.12027918221652E-15));
#43839=DIRECTION('ref_axis',(0.976751692957689,-5.97760464746442E-16,0.214373809744306));
#43840=DIRECTION('center_axis',(3.66113466765132E-16,1.,1.12027918221652E-15));
#43841=DIRECTION('ref_axis',(0.0817210741336744,-1.14645130220395E-15,0.99665523930918));
#43842=DIRECTION('center_axis',(3.66113466765132E-16,1.,1.12027918221652E-15));
#43843=DIRECTION('ref_axis',(-0.850327489419754,-2.78234936744637E-16,0.526253893797564));
#43844=DIRECTION('center_axis',(-3.66113466765132E-16,-1.,-1.12027918221652E-15));
#43845=DIRECTION('ref_axis',(5.46077161851015E-15,-1.12027918221652E-15,
1.));
#43846=DIRECTION('center_axis',(3.66113466765132E-16,1.,1.12027918221652E-15));
#43847=DIRECTION('ref_axis',(0.996376843918701,-4.60064633258624E-16,0.0850481328578616));
#43848=DIRECTION('center_axis',(3.66113466765132E-16,1.,1.12027918221652E-15));
#43849=DIRECTION('ref_axis',(0.211111552358972,-1.17232108424584E-15,0.97746197494357));
#43850=DIRECTION('center_axis',(3.66113466765132E-16,1.,1.12027918221652E-15));
#43851=DIRECTION('ref_axis',(-0.774362902971737,-4.25342698788503E-16,0.632741728117551));
#43852=DIRECTION('center_axis',(-3.66113466765132E-16,-1.,-1.12027918221652E-15));
#43853=DIRECTION('ref_axis',(5.46077161851015E-15,-1.12027918221652E-15,
1.));
#43854=DIRECTION('center_axis',(3.66113466765132E-16,1.,1.12027918221652E-15));
#43855=DIRECTION('ref_axis',(0.998953710832413,-3.14496968341737E-16,-0.0457327411615765));
#43856=DIRECTION('center_axis',(3.66113466765132E-16,1.,1.12027918221652E-15));
#43857=DIRECTION('ref_axis',(0.336889853392226,-1.17813212750748E-15,0.941544065183018));
#43858=DIRECTION('center_axis',(3.66113466765132E-16,1.,1.12027918221652E-15));
#43859=DIRECTION('ref_axis',(-0.685148752559916,-5.65172729328823E-16,0.728403176040296));
#43860=DIRECTION('center_axis',(-3.66113466765132E-16,-1.,-1.12027918221652E-15));
#43861=DIRECTION('ref_axis',(5.46077161851015E-15,-1.12027918221652E-15,
1.));
#43862=DIRECTION('center_axis',(3.66113466765132E-16,1.,1.12027918221652E-15));
#43863=DIRECTION('ref_axis',(0.98443820279149,-1.63548173101491E-16,-0.175731115300228));
#43864=DIRECTION('center_axis',(3.66113466765132E-16,1.,1.12027918221652E-15));
#43865=DIRECTION('ref_axis',(0.456903875630426,-1.16378500342752E-15,0.889516075421853));
#43866=DIRECTION('center_axis',(3.66113466765132E-16,1.,1.12027918221652E-15));
#43867=DIRECTION('ref_axis',(-0.584211517032673,-6.95332497774842E-16,0.811601443669479));
#43868=DIRECTION('center_axis',(-3.66113466765132E-16,-1.,-1.12027918221652E-15));
#43869=DIRECTION('ref_axis',(5.46077161851015E-15,-1.12027918221652E-15,
1.));
#43870=DIRECTION('center_axis',(3.66113466765132E-16,1.,1.12027918221652E-15));
#43871=DIRECTION('ref_axis',(0.95307868416297,-9.80102327535809E-18,-0.302722681334224));
#43872=DIRECTION('center_axis',(3.66113466765132E-16,1.,1.12027918221652E-15));
#43873=DIRECTION('ref_axis',(0.569100145878903,-1.12952519527676E-15,0.822268218989772));
#43874=DIRECTION('center_axis',(3.66113466765132E-16,1.,1.12027918221652E-15));
#43875=DIRECTION('ref_axis',(-0.473278260474969,-8.13594934401345E-16,0.880912985579045));
#43876=DIRECTION('center_axis',(-3.66113466765132E-16,-1.,-1.12027918221652E-15));
#43877=DIRECTION('ref_axis',(5.46077161851015E-15,-1.12027918221652E-15,
1.));
#43878=DIRECTION('center_axis',(3.66113466765132E-16,1.,1.12027918221652E-15));
#43879=DIRECTION('ref_axis',(0.905411725005089,1.44113824776374E-16,-0.424534578360008));
#43880=DIRECTION('center_axis',(3.66113466765132E-16,1.,1.12027918221652E-15));
#43881=DIRECTION('ref_axis',(0.671558954847023,-1.07593889787127E-15,0.740951125354955));
#43882=DIRECTION('center_axis',(3.66113466765132E-16,1.,1.12027918221652E-15));
#43883=DIRECTION('ref_axis',(-0.354247081663014,-9.17936536129109E-16,0.935151862070134));
#43884=DIRECTION('center_axis',(-3.66113466765132E-16,-1.,-1.12027918221652E-15));
#43885=DIRECTION('ref_axis',(5.46077161851015E-15,-1.12027918221652E-15,
1.));
#43886=DIRECTION('center_axis',(3.66113466765132E-16,1.,1.12027918221652E-15));
#43887=DIRECTION('ref_axis',(0.842252920204816,2.9556284533028E-16,-0.53908257104683));
#43888=DIRECTION('center_axis',(3.66113466765132E-16,1.,1.12027918221652E-15));
#43889=DIRECTION('ref_axis',(0.762527203906392,-1.00394298761658E-15,0.646956152534853));
#43890=DIRECTION('center_axis',(3.66113466765132E-16,1.,1.12027918221652E-15));
#43891=DIRECTION('ref_axis',(-0.229154637067958,-1.00657198922362E-15,0.973390030928123));
#43892=DIRECTION('center_axis',(-3.66113466765132E-16,-1.,-1.12027918221652E-15));
#43893=DIRECTION('ref_axis',(5.46077161851015E-15,-1.12027918221652E-15,
1.));
#43894=DIRECTION('center_axis',(3.66113466765132E-16,1.,1.12027918221652E-15));
#43895=DIRECTION('ref_axis',(0.764682934423213,4.41954703655085E-16,-0.644406711481115));
#43896=DIRECTION('center_axis',(3.66113466765132E-16,1.,1.12027918221652E-15));
#43897=DIRECTION('ref_axis',(0.840448401094441,-9.14769334498193E-16,0.541891580574747));
#43898=DIRECTION('center_axis',(3.66113466765132E-16,1.,1.12027918221652E-15));
#43899=DIRECTION('ref_axis',(-0.100141293099002,-1.07798471650803E-15,0.994973226482231));
#43900=DIRECTION('center_axis',(-3.66113466765132E-16,-1.,-1.12027918221652E-15));
#43901=DIRECTION('ref_axis',(5.46077161851015E-15,-1.12027918221652E-15,
1.));
#43902=DIRECTION('center_axis',(3.66113466765132E-16,1.,1.12027918221652E-15));
#43903=DIRECTION('ref_axis',(0.674029011623465,5.80784594467357E-16,-0.738704874418665));
#43904=DIRECTION('center_axis',(3.66113466765132E-16,1.,1.12027918221652E-15));
#43905=DIRECTION('ref_axis',(0.903989293123446,-8.09943724444564E-16,0.427555093430276));
#43906=DIRECTION('center_axis',(3.66113466765132E-16,1.,1.12027918221652E-15));
#43907=DIRECTION('ref_axis',(0.0305854961592909,-1.13095282641916E-15,0.999532154272533));
#43908=DIRECTION('center_axis',(-3.66113466765132E-16,-1.,-1.12027918221652E-15));
#43909=DIRECTION('ref_axis',(5.46077161851015E-15,-1.12027918221652E-15,
1.));
#43910=DIRECTION('center_axis',(3.66113466765132E-16,1.,1.12027918221652E-15));
#43911=DIRECTION('ref_axis',(0.571842265558692,7.09677099844383E-16,-0.820363592147227));
#43912=DIRECTION('center_axis',(3.66113466765132E-16,1.,1.12027918221652E-15));
#43913=DIRECTION('ref_axis',(0.952062677713926,-6.91259752706864E-16,0.305903020096547));
#43914=DIRECTION('center_axis',(3.66113466765132E-16,1.,1.12027918221652E-15));
#43915=DIRECTION('ref_axis',(0.160788959098396,-1.1645700199109E-15,0.986988809780564));
#43916=DIRECTION('center_axis',(-3.66113466765132E-16,-1.,-1.12027918221652E-15));
#43917=DIRECTION('ref_axis',(5.46077161851015E-15,-1.12027918221652E-15,
1.));
#43918=DIRECTION('center_axis',(3.66113466765132E-16,1.,1.12027918221652E-15));
#43919=DIRECTION('ref_axis',(0.459871139785583,8.26426833283406E-16,-0.887985661366392));
#43920=DIRECTION('center_axis',(3.66113466765132E-16,1.,1.12027918221652E-15));
#43921=DIRECTION('ref_axis',(0.983846005927078,-5.60748134946939E-16,0.179016861276626));
#43922=DIRECTION('center_axis',(3.66113466765132E-16,1.,1.12027918221652E-15));
#43923=DIRECTION('ref_axis',(0.288241278368206,-1.17826109748215E-15,0.957557813108254));
#43924=DIRECTION('center_axis',(-3.66113466765132E-16,-1.,-1.12027918221652E-15));
#43925=DIRECTION('ref_axis',(5.46077161851015E-15,-1.12027918221652E-15,
1.));
#43926=DIRECTION('center_axis',(3.66113466765132E-16,1.,1.12027918221652E-15));
#43927=DIRECTION('ref_axis',(0.340031491310375,9.29036174476144E-16,-0.940414049723441));
#43928=DIRECTION('center_axis',(3.66113466765132E-16,1.,1.12027918221652E-15));
#43929=DIRECTION('ref_axis',(0.998795456205173,-4.20641961129317E-16,0.0490676743274118));
#43930=DIRECTION('center_axis',(3.66113466765132E-16,1.,1.12027918221652E-15));
#43931=DIRECTION('ref_axis',(0.410761709449557,-1.17179180099979E-15,0.91174273676848));
#43932=DIRECTION('center_axis',(-3.66113466765132E-16,-1.,-1.12027918221652E-15));
#43933=DIRECTION('ref_axis',(5.46077161851015E-15,-1.12027918221652E-15,
1.));
#43934=DIRECTION('center_axis',(3.66113466765132E-16,1.,1.12027918221652E-15));
#43935=DIRECTION('ref_axis',(0.214373809744306,1.01574944914611E-15,-0.976751692957689));
#43936=DIRECTION('center_axis',(3.66113466765132E-16,1.,1.12027918221652E-15));
#43937=DIRECTION('ref_axis',(0.99665523930918,-2.73338486732788E-16,-0.0817210741336743));
#43938=DIRECTION('center_axis',(3.66113466765132E-16,1.,1.12027918221652E-15));
#43939=DIRECTION('ref_axis',(0.526253893797564,-1.14527282192027E-15,0.850327489419754));
#43940=DIRECTION('center_axis',(-3.66113466765132E-16,-1.,-1.12027918221652E-15));
#43941=DIRECTION('ref_axis',(5.46077161851015E-15,-1.12027918221652E-15,
1.));
#43942=DIRECTION('center_axis',(3.66113466765132E-16,1.,1.12027918221652E-15));
#43943=DIRECTION('ref_axis',(0.0850481328578621,1.08508296912223E-15,-0.996376843918701));
#43944=DIRECTION('center_axis',(3.66113466765132E-16,1.,1.12027918221652E-15));
#43945=DIRECTION('ref_axis',(0.977461974943571,-1.21358115044515E-16,-0.211111552358971));
#43946=DIRECTION('center_axis',(3.66113466765132E-16,1.,1.12027918221652E-15));
#43947=DIRECTION('ref_axis',(0.63274172811755,-1.09915790732807E-15,0.774362902971737));
#43948=DIRECTION('center_axis',(-3.66113466765132E-16,-1.,-1.12027918221652E-15));
#43949=DIRECTION('ref_axis',(5.46077161851015E-15,-1.12027918221652E-15,
1.));
#43950=DIRECTION('center_axis',(3.66113466765132E-16,1.,1.12027918221652E-15));
#43951=DIRECTION('ref_axis',(-0.0457327411615761,1.13585041865483E-15,-0.998953710832413));
#43952=DIRECTION('center_axis',(3.66113466765132E-16,1.,1.12027918221652E-15));
#43953=DIRECTION('ref_axis',(0.941544065183019,3.2698727638996E-17,-0.336889853392226));
#43954=DIRECTION('center_axis',(3.66113466765132E-16,1.,1.12027918221652E-15));
#43955=DIRECTION('ref_axis',(0.728403176040296,-1.03423609619734E-15,0.685148752559917));
#43956=DIRECTION('center_axis',(-3.66113466765132E-16,-1.,-1.12027918221652E-15));
#43957=DIRECTION('ref_axis',(5.46077161851015E-15,-1.12027918221652E-15,
1.));
#43958=DIRECTION('center_axis',(3.66113466765132E-16,1.,1.12027918221652E-15));
#43959=DIRECTION('ref_axis',(-0.175731115300228,1.16718315260702E-15,-0.98443820279149));
#43960=DIRECTION('center_axis',(3.66113466765132E-16,1.,1.12027918221652E-15));
#43961=DIRECTION('ref_axis',(0.889516075421853,1.86196086026803E-16,-0.456903875630426));
#43962=DIRECTION('center_axis',(3.66113466765132E-16,1.,1.12027918221652E-15));
#43963=DIRECTION('ref_axis',(0.811601443669479,-9.51618218716256E-16,0.584211517032674));
#43964=DIRECTION('center_axis',(-3.66113466765132E-16,-1.,-1.12027918221652E-15));
#43965=DIRECTION('ref_axis',(5.46077161851015E-15,-1.12027918221652E-15,
1.));
#43966=DIRECTION('center_axis',(3.66113466765132E-16,1.,1.12027918221652E-15));
#43967=DIRECTION('ref_axis',(-0.302722681334224,1.1785450592138E-15,-0.95307868416297));
#43968=DIRECTION('center_axis',(3.66113466765132E-16,1.,1.12027918221652E-15));
#43969=DIRECTION('ref_axis',(0.822268218989772,3.36507577759385E-16,-0.569100145878903));
#43970=DIRECTION('center_axis',(3.66113466765132E-16,1.,1.12027918221652E-15));
#43971=DIRECTION('ref_axis',(0.880912985579045,-8.52717889674523E-16,0.473278260474969));
#43972=DIRECTION('center_axis',(-3.66113466765132E-16,-1.,-1.12027918221652E-15));
#43973=DIRECTION('ref_axis',(5.46077161851015E-15,-1.12027918221652E-15,
1.));
#43974=DIRECTION('center_axis',(3.66113466765132E-16,1.,1.12027918221652E-15));
#43975=DIRECTION('ref_axis',(-0.424534578360008,1.16974173310301E-15,-0.905411725005089));
#43976=DIRECTION('center_axis',(3.66113466765132E-16,1.,1.12027918221652E-15));
#43977=DIRECTION('ref_axis',(0.740951125354955,4.81061331538975E-16,-0.671558954847023));
#43978=DIRECTION('center_axis',(3.66113466765132E-16,1.,1.12027918221652E-15));
#43979=DIRECTION('ref_axis',(0.935151862070134,-7.39227321122395E-16,0.354247081663014));
#43980=DIRECTION('center_axis',(-3.66113466765132E-16,-1.,-1.12027918221652E-15));
#43981=DIRECTION('ref_axis',(5.46077161851015E-15,-1.12027918221652E-15,
1.));
#43982=DIRECTION('center_axis',(3.66113466765132E-16,1.,1.12027918221652E-15));
#43983=DIRECTION('ref_axis',(-0.53908257104683,1.14092380162514E-15,-0.842252920204816));
#43984=DIRECTION('center_axis',(3.66113466765132E-16,1.,1.12027918221652E-15));
#43985=DIRECTION('ref_axis',(0.646956152534853,6.17383992560536E-16,-0.762527203906392));
#43986=DIRECTION('center_axis',(3.66113466765132E-16,1.,1.12027918221652E-15));
#43987=DIRECTION('ref_axis',(0.973390030928123,-6.13088368153331E-16,0.229154637067959));
#43988=DIRECTION('center_axis',(-3.66113466765132E-16,-1.,-1.12027918221652E-15));
#43989=DIRECTION('ref_axis',(5.46077161851015E-15,-1.12027918221652E-15,
1.));
#43990=DIRECTION('center_axis',(3.66113466765132E-16,1.,1.12027918221652E-15));
#43991=DIRECTION('ref_axis',(-0.644406711481115,1.09258434757764E-15,-0.764682934423213));
#43992=DIRECTION('center_axis',(3.66113466765132E-16,1.,1.12027918221652E-15));
#43993=DIRECTION('ref_axis',(0.541891580574746,7.43143042298206E-16,-0.840448401094442));
#43994=DIRECTION('center_axis',(3.66113466765132E-16,1.,1.12027918221652E-15));
#43995=DIRECTION('ref_axis',(0.994973226482231,-4.76459303224953E-16,0.100141293099002));
#43996=DIRECTION('center_axis',(-3.66113466765132E-16,-1.,-1.12027918221652E-15));
#43997=DIRECTION('ref_axis',(5.46077161851015E-15,-1.12027918221652E-15,
1.));
#43998=DIRECTION('center_axis',(3.66113466765132E-16,1.,1.12027918221652E-15));
#43999=DIRECTION('ref_axis',(-0.738704874418665,1.02555047242146E-15,-0.674029011623465));
#44000=DIRECTION('center_axis',(3.66113466765132E-16,1.,1.12027918221652E-15));
#44001=DIRECTION('ref_axis',(0.427555093430276,8.56186708543976E-16,-0.903989293123446));
#44002=DIRECTION('center_axis',(3.66113466765132E-16,1.,1.12027918221652E-15));
#44003=DIRECTION('ref_axis',(0.999532154272533,-3.31677887518921E-16,-0.0305854961592909));
#44004=DIRECTION('center_axis',(-3.66113466765132E-16,-1.,-1.12027918221652E-15));
#44005=DIRECTION('ref_axis',(5.46077161851015E-15,-1.12027918221652E-15,
1.));
#44006=DIRECTION('center_axis',(3.66113466765132E-16,1.,1.12027918221652E-15));
#44007=DIRECTION('ref_axis',(-0.820363592147226,9.40969144345854E-16,-0.571842265558694));
#44008=DIRECTION('center_axis',(3.66113466765132E-16,1.,1.12027918221652E-15));
#44009=DIRECTION('ref_axis',(0.305903020096548,9.54580782826757E-16,-0.952062677713926));
#44010=DIRECTION('center_axis',(3.66113466765132E-16,1.,1.12027918221652E-15));
#44011=DIRECTION('ref_axis',(0.986988809780564,-1.81221371198957E-16,-0.160788959098396));
#44012=DIRECTION('center_axis',(-3.66113466765132E-16,-1.,-1.12027918221652E-15));
#44013=DIRECTION('ref_axis',(5.46077161851015E-15,-1.12027918221652E-15,
1.));
#44014=DIRECTION('center_axis',(3.66113466765132E-16,1.,1.12027918221652E-15));
#44015=DIRECTION('ref_axis',(-0.887985661366392,8.40287573324551E-16,-0.459871139785583));
#44016=DIRECTION('center_axis',(3.66113466765132E-16,1.,1.12027918221652E-15));
#44017=DIRECTION('ref_axis',(0.179016861276627,1.03664171525558E-15,-0.983846005927078));
#44018=DIRECTION('center_axis',(3.66113466765132E-16,1.,1.12027918221652E-15));
#44019=DIRECTION('ref_axis',(0.957557813108254,-2.76641069737229E-17,-0.288241278368206));
#44020=DIRECTION('center_axis',(-3.66113466765132E-16,-1.,-1.12027918221652E-15));
#44021=DIRECTION('ref_axis',(5.46077161851015E-15,-1.12027918221652E-15,
1.));
#44022=DIRECTION('center_axis',(3.66113466765132E-16,1.,1.12027918221652E-15));
#44023=DIRECTION('ref_axis',(-0.940414049723441,7.25228448951937E-16,-0.340031491310375));
#44024=DIRECTION('center_axis',(3.66113466765132E-16,1.,1.12027918221652E-15));
#44025=DIRECTION('ref_axis',(0.0490676743274116,1.100965420525E-15,-0.998795456205173));
#44026=DIRECTION('center_axis',(3.66113466765132E-16,1.,1.12027918221652E-15));
#44027=DIRECTION('ref_axis',(0.91174273676848,1.26366497791772E-16,-0.410761709449557));
#44028=DIRECTION('center_axis',(-3.66113466765132E-16,-1.,-1.12027918221652E-15));
#44029=DIRECTION('ref_axis',(5.46077161851015E-15,-1.12027918221652E-15,
1.));
#44030=DIRECTION('center_axis',(3.66113466765132E-16,1.,1.12027918221652E-15));
#44031=DIRECTION('ref_axis',(-0.976751692957689,5.97760464746442E-16,-0.214373809744306));
#44032=DIRECTION('center_axis',(3.66113466765132E-16,1.,1.12027918221652E-15));
#44033=DIRECTION('ref_axis',(-0.081721074133674,1.14645130220395E-15,-0.99665523930918));
#44034=DIRECTION('center_axis',(3.66113466765132E-16,1.,1.12027918221652E-15));
#44035=DIRECTION('ref_axis',(0.850327489419755,2.78234936744635E-16,-0.526253893797563));
#44036=DIRECTION('center_axis',(-3.66113466765132E-16,-1.,-1.12027918221652E-15));
#44037=DIRECTION('ref_axis',(5.46077161851015E-15,-1.12027918221652E-15,
1.));
#44038=DIRECTION('center_axis',(3.66113466765132E-16,1.,1.12027918221652E-15));
#44039=DIRECTION('ref_axis',(-0.996376843918701,4.60064633258625E-16,-0.0850481328578625));
#44040=DIRECTION('center_axis',(3.66113466765132E-16,1.,1.12027918221652E-15));
#44041=DIRECTION('ref_axis',(-0.211111552358971,1.17232108424584E-15,-0.977461974943571));
#44042=DIRECTION('center_axis',(3.66113466765132E-16,1.,1.12027918221652E-15));
#44043=DIRECTION('ref_axis',(0.774362902971737,4.25342698788503E-16,-0.63274172811755));
#44044=DIRECTION('center_axis',(-3.66113466765132E-16,-1.,-1.12027918221652E-15));
#44045=DIRECTION('ref_axis',(5.46077161851015E-15,-1.12027918221652E-15,
1.));
#44046=DIRECTION('center_axis',(3.66113466765132E-16,1.,1.12027918221652E-15));
#44047=DIRECTION('ref_axis',(-0.998953710832413,3.14496968341738E-16,0.045732741161576));
#44048=DIRECTION('center_axis',(3.66113466765132E-16,1.,1.12027918221652E-15));
#44049=DIRECTION('ref_axis',(-0.336889853392226,1.17813212750748E-15,-0.941544065183019));
#44050=DIRECTION('center_axis',(3.66113466765132E-16,1.,1.12027918221652E-15));
#44051=DIRECTION('ref_axis',(0.685148752559917,5.65172729328822E-16,-0.728403176040296));
#44052=DIRECTION('center_axis',(-3.66113466765132E-16,-1.,-1.12027918221652E-15));
#44053=DIRECTION('ref_axis',(5.46077161851015E-15,-1.12027918221652E-15,
1.));
#44054=DIRECTION('center_axis',(3.66113466765132E-16,1.,1.12027918221652E-15));
#44055=DIRECTION('ref_axis',(-0.98443820279149,1.63548173101491E-16,0.175731115300228));
#44056=DIRECTION('center_axis',(3.66113466765132E-16,1.,1.12027918221652E-15));
#44057=DIRECTION('ref_axis',(-0.456903875630426,1.16378500342752E-15,-0.889516075421853));
#44058=DIRECTION('center_axis',(3.66113466765132E-16,1.,1.12027918221652E-15));
#44059=DIRECTION('ref_axis',(0.584211517032674,6.95332497774842E-16,-0.811601443669479));
#44060=DIRECTION('center_axis',(-3.66113466765132E-16,-1.,-1.12027918221652E-15));
#44061=DIRECTION('ref_axis',(5.46077161851015E-15,-1.12027918221652E-15,
1.));
#44062=DIRECTION('center_axis',(3.66113466765132E-16,1.,1.12027918221652E-15));
#44063=DIRECTION('ref_axis',(-0.95307868416297,9.80102327535809E-18,0.302722681334224));
#44064=DIRECTION('center_axis',(3.66113466765132E-16,1.,1.12027918221652E-15));
#44065=DIRECTION('ref_axis',(-0.569100145878903,1.12952519527676E-15,-0.822268218989772));
#44066=DIRECTION('center_axis',(3.66113466765132E-16,1.,1.12027918221652E-15));
#44067=DIRECTION('ref_axis',(0.473278260474969,8.13594934401345E-16,-0.880912985579045));
#44068=DIRECTION('center_axis',(-3.66113466765132E-16,-1.,-1.12027918221652E-15));
#44069=DIRECTION('ref_axis',(5.46077161851015E-15,-1.12027918221652E-15,
1.));
#44070=DIRECTION('center_axis',(3.66113466765132E-16,1.,1.12027918221652E-15));
#44071=DIRECTION('ref_axis',(-0.905411725005089,-1.44113824776374E-16,0.424534578360008));
#44072=DIRECTION('center_axis',(3.66113466765132E-16,1.,1.12027918221652E-15));
#44073=DIRECTION('ref_axis',(-0.671558954847023,1.07593889787127E-15,-0.740951125354955));
#44074=DIRECTION('center_axis',(3.66113466765132E-16,1.,1.12027918221652E-15));
#44075=DIRECTION('ref_axis',(0.354247081663014,9.17936536129109E-16,-0.935151862070134));
#44076=DIRECTION('center_axis',(-3.66113466765132E-16,-1.,-1.12027918221652E-15));
#44077=DIRECTION('ref_axis',(5.46077161851015E-15,-1.12027918221652E-15,
1.));
#44078=DIRECTION('center_axis',(3.66113466765132E-16,1.,1.12027918221652E-15));
#44079=DIRECTION('ref_axis',(-0.842252920204816,-2.9556284533028E-16,0.53908257104683));
#44080=DIRECTION('center_axis',(3.66113466765132E-16,1.,1.12027918221652E-15));
#44081=DIRECTION('ref_axis',(-0.762527203906392,1.00394298761658E-15,-0.646956152534853));
#44082=DIRECTION('center_axis',(3.66113466765132E-16,1.,1.12027918221652E-15));
#44083=DIRECTION('ref_axis',(0.229154637067959,1.00657198922362E-15,-0.973390030928123));
#44084=DIRECTION('center_axis',(-3.66113466765132E-16,-1.,-1.12027918221652E-15));
#44085=DIRECTION('ref_axis',(5.46077161851015E-15,-1.12027918221652E-15,
1.));
#44086=DIRECTION('center_axis',(3.66113466765132E-16,1.,1.12027918221652E-15));
#44087=DIRECTION('ref_axis',(-0.764682934423213,-4.41954703655085E-16,0.644406711481115));
#44088=DIRECTION('center_axis',(3.66113466765132E-16,1.,1.12027918221652E-15));
#44089=DIRECTION('ref_axis',(-0.840448401094441,9.14769334498193E-16,-0.541891580574747));
#44090=DIRECTION('center_axis',(3.66113466765132E-16,1.,1.12027918221652E-15));
#44091=DIRECTION('ref_axis',(0.100141293099002,1.07798471650803E-15,-0.994973226482231));
#44092=DIRECTION('center_axis',(-3.66113466765132E-16,-1.,-1.12027918221652E-15));
#44093=DIRECTION('ref_axis',(5.46077161851015E-15,-1.12027918221652E-15,
1.));
#44094=DIRECTION('center_axis',(3.66113466765132E-16,1.,1.12027918221652E-15));
#44095=DIRECTION('ref_axis',(-0.674029011623465,-5.80784594467357E-16,0.738704874418665));
#44096=DIRECTION('center_axis',(3.66113466765132E-16,1.,1.12027918221652E-15));
#44097=DIRECTION('ref_axis',(-0.903989293123446,8.09943724444565E-16,-0.427555093430277));
#44098=DIRECTION('center_axis',(3.66113466765132E-16,1.,1.12027918221652E-15));
#44099=DIRECTION('ref_axis',(-0.0305854961592907,1.13095282641916E-15,-0.999532154272533));
#44100=DIRECTION('center_axis',(-3.66113466765132E-16,-1.,-1.12027918221652E-15));
#44101=DIRECTION('ref_axis',(5.46077161851015E-15,-1.12027918221652E-15,
1.));
#44102=DIRECTION('center_axis',(3.66113466765132E-16,1.,1.12027918221652E-15));
#44103=DIRECTION('ref_axis',(-0.571842265558694,-7.09677099844381E-16,0.820363592147226));
#44104=DIRECTION('center_axis',(3.66113466765132E-16,1.,1.12027918221652E-15));
#44105=DIRECTION('ref_axis',(-0.952062677713926,6.91259752706865E-16,-0.305903020096548));
#44106=DIRECTION('center_axis',(3.66113466765132E-16,1.,1.12027918221652E-15));
#44107=DIRECTION('ref_axis',(-0.160788959098396,1.1645700199109E-15,-0.986988809780564));
#44108=DIRECTION('center_axis',(-3.66113466765132E-16,-1.,-1.12027918221652E-15));
#44109=DIRECTION('ref_axis',(5.46077161851015E-15,-1.12027918221652E-15,
1.));
#44110=DIRECTION('center_axis',(3.66113466765132E-16,1.,1.12027918221652E-15));
#44111=DIRECTION('ref_axis',(-0.459871139785583,-8.26426833283405E-16,0.887985661366392));
#44112=DIRECTION('center_axis',(3.66113466765132E-16,1.,1.12027918221652E-15));
#44113=DIRECTION('ref_axis',(-0.983846005927078,5.60748134946939E-16,-0.179016861276627));
#44114=DIRECTION('center_axis',(3.66113466765132E-16,1.,1.12027918221652E-15));
#44115=DIRECTION('ref_axis',(-0.288241278368206,1.17826109748215E-15,-0.957557813108254));
#44116=DIRECTION('center_axis',(-3.66113466765132E-16,-1.,-1.12027918221652E-15));
#44117=DIRECTION('ref_axis',(5.46077161851015E-15,-1.12027918221652E-15,
1.));
#44118=DIRECTION('center_axis',(3.66113466765132E-16,1.,1.12027918221652E-15));
#44119=DIRECTION('ref_axis',(-0.340031491310375,-9.29036174476144E-16,0.940414049723441));
#44120=DIRECTION('center_axis',(3.66113466765132E-16,1.,1.12027918221652E-15));
#44121=DIRECTION('ref_axis',(-0.998795456205173,4.20641961129317E-16,-0.0490676743274121));
#44122=DIRECTION('center_axis',(3.66113466765132E-16,1.,1.12027918221652E-15));
#44123=DIRECTION('ref_axis',(-0.410761709449556,1.17179180099979E-15,-0.91174273676848));
#44124=DIRECTION('center_axis',(-3.66113466765132E-16,-1.,-1.12027918221652E-15));
#44125=DIRECTION('ref_axis',(5.46077161851015E-15,-1.12027918221652E-15,
1.));
#44126=DIRECTION('center_axis',(3.66113466765132E-16,1.,1.12027918221652E-15));
#44127=DIRECTION('ref_axis',(-0.214373809744306,-1.01574944914611E-15,0.976751692957689));
#44128=DIRECTION('center_axis',(3.66113466765132E-16,1.,1.12027918221652E-15));
#44129=DIRECTION('ref_axis',(-0.99665523930918,2.73338486732788E-16,0.0817210741336742));
#44130=DIRECTION('center_axis',(3.66113466765132E-16,1.,1.12027918221652E-15));
#44131=DIRECTION('ref_axis',(-0.526253893797564,1.14527282192027E-15,-0.850327489419754));
#44132=DIRECTION('center_axis',(-3.66113466765132E-16,-1.,-1.12027918221652E-15));
#44133=DIRECTION('ref_axis',(5.46077161851015E-15,-1.12027918221652E-15,
1.));
#44134=DIRECTION('center_axis',(1.,-3.66113466765126E-16,-5.46077161851015E-15));
#44135=DIRECTION('ref_axis',(5.46077161851015E-15,-1.12027918221652E-15,
1.));
#44136=DIRECTION('',(-5.46077161851015E-15,1.12027918221652E-15,-1.));
#44137=DIRECTION('',(-3.66113466765132E-16,-1.,-1.12027918221652E-15));
#44138=DIRECTION('',(-3.66113466765132E-16,-1.,-1.12027918221652E-15));
#44139=DIRECTION('center_axis',(-5.46077161851015E-15,1.12027918221652E-15,
-1.));
#44140=DIRECTION('ref_axis',(1.,-3.66113466765126E-16,-5.46077161851015E-15));
#44141=DIRECTION('',(-1.,3.66113466765126E-16,5.46077161851015E-15));
#44142=DIRECTION('',(3.66113466765132E-16,1.,1.12027918221652E-15));
#44143=DIRECTION('center_axis',(-3.66113466765132E-16,-1.,-1.12027918221652E-15));
#44144=DIRECTION('ref_axis',(-1.,3.66113466765124E-16,6.8542715880177E-15));
#44145=DIRECTION('center_axis',(3.66113466765132E-16,1.,1.12027918221652E-15));
#44146=DIRECTION('ref_axis',(5.46077161851015E-15,-1.12027918221652E-15,
1.));
#44147=DIRECTION('',(-3.66113466765132E-16,-1.,-1.12027918221652E-15));
#44148=DIRECTION('center_axis',(5.46077161851015E-15,-1.12027918221652E-15,
1.));
#44149=DIRECTION('ref_axis',(-1.,3.66113466765126E-16,5.46077161851015E-15));
#44150=DIRECTION('',(1.,-3.66113466765126E-16,-5.46077161851015E-15));
#44151=DIRECTION('center_axis',(3.66113466765132E-16,1.,1.12027918221652E-15));
#44152=DIRECTION('ref_axis',(-0.97746197494357,1.21358115044514E-16,0.211111552358972));
#44153=DIRECTION('',(3.66113466765132E-16,1.,1.12027918221652E-15));
#44154=DIRECTION('center_axis',(-3.66113466765132E-16,-1.,-1.12027918221652E-15));
#44155=DIRECTION('ref_axis',(-0.97746197494357,1.21358115044514E-16,0.211111552358972));
#44156=DIRECTION('',(3.66113466765132E-16,1.,1.12027918221652E-15));
#44157=DIRECTION('center_axis',(3.66113466765132E-16,1.,1.12027918221652E-15));
#44158=DIRECTION('ref_axis',(-0.632741728117551,1.09915790732807E-15,-0.774362902971737));
#44159=DIRECTION('center_axis',(-3.66113466765132E-16,-1.,-1.12027918221652E-15));
#44160=DIRECTION('ref_axis',(-0.632741728117551,1.09915790732807E-15,-0.774362902971737));
#44161=DIRECTION('',(-3.66113466765132E-16,-1.,-1.12027918221652E-15));
#44162=DIRECTION('center_axis',(3.66113466765132E-16,1.,1.12027918221652E-15));
#44163=DIRECTION('ref_axis',(-0.0850481328578615,-1.08508296912223E-15,
0.996376843918701));
#44164=DIRECTION('',(3.66113466765132E-16,1.,1.12027918221652E-15));
#44165=DIRECTION('center_axis',(-3.66113466765132E-16,-1.,-1.12027918221652E-15));
#44166=DIRECTION('ref_axis',(-0.0850481328578615,-1.08508296912223E-15,
0.996376843918701));
#44167=DIRECTION('center_axis',(3.66113466765132E-16,1.,1.12027918221652E-15));
#44168=DIRECTION('ref_axis',(-0.941544065183018,-3.26987276389964E-17,0.336889853392226));
#44169=DIRECTION('',(3.66113466765132E-16,1.,1.12027918221652E-15));
#44170=DIRECTION('center_axis',(-3.66113466765132E-16,-1.,-1.12027918221652E-15));
#44171=DIRECTION('ref_axis',(-0.941544065183018,-3.26987276389964E-17,0.336889853392226));
#44172=DIRECTION('',(3.66113466765132E-16,1.,1.12027918221652E-15));
#44173=DIRECTION('center_axis',(3.66113466765132E-16,1.,1.12027918221652E-15));
#44174=DIRECTION('ref_axis',(-0.728403176040296,1.03423609619734E-15,-0.685148752559916));
#44175=DIRECTION('center_axis',(-3.66113466765132E-16,-1.,-1.12027918221652E-15));
#44176=DIRECTION('ref_axis',(-0.728403176040296,1.03423609619734E-15,-0.685148752559916));
#44177=DIRECTION('',(-3.66113466765132E-16,-1.,-1.12027918221652E-15));
#44178=DIRECTION('center_axis',(3.66113466765132E-16,1.,1.12027918221652E-15));
#44179=DIRECTION('ref_axis',(0.0457327411615766,-1.13585041865483E-15,0.998953710832413));
#44180=DIRECTION('',(3.66113466765132E-16,1.,1.12027918221652E-15));
#44181=DIRECTION('center_axis',(-3.66113466765132E-16,-1.,-1.12027918221652E-15));
#44182=DIRECTION('ref_axis',(0.0457327411615766,-1.13585041865483E-15,0.998953710832413));
#44183=DIRECTION('center_axis',(3.66113466765132E-16,1.,1.12027918221652E-15));
#44184=DIRECTION('ref_axis',(-0.889516075421853,-1.86196086026804E-16,0.456903875630427));
#44185=DIRECTION('',(3.66113466765132E-16,1.,1.12027918221652E-15));
#44186=DIRECTION('center_axis',(-3.66113466765132E-16,-1.,-1.12027918221652E-15));
#44187=DIRECTION('ref_axis',(-0.889516075421853,-1.86196086026804E-16,0.456903875630427));
#44188=DIRECTION('',(3.66113466765132E-16,1.,1.12027918221652E-15));
#44189=DIRECTION('center_axis',(3.66113466765132E-16,1.,1.12027918221652E-15));
#44190=DIRECTION('ref_axis',(-0.811601443669479,9.51618218716255E-16,-0.584211517032673));
#44191=DIRECTION('center_axis',(-3.66113466765132E-16,-1.,-1.12027918221652E-15));
#44192=DIRECTION('ref_axis',(-0.811601443669479,9.51618218716255E-16,-0.584211517032673));
#44193=DIRECTION('',(-3.66113466765132E-16,-1.,-1.12027918221652E-15));
#44194=DIRECTION('center_axis',(3.66113466765132E-16,1.,1.12027918221652E-15));
#44195=DIRECTION('ref_axis',(0.175731115300229,-1.16718315260702E-15,0.984438202791489));
#44196=DIRECTION('',(3.66113466765132E-16,1.,1.12027918221652E-15));
#44197=DIRECTION('center_axis',(-3.66113466765132E-16,-1.,-1.12027918221652E-15));
#44198=DIRECTION('ref_axis',(0.175731115300229,-1.16718315260702E-15,0.984438202791489));
#44199=DIRECTION('center_axis',(3.66113466765132E-16,1.,1.12027918221652E-15));
#44200=DIRECTION('ref_axis',(-0.822268218989772,-3.36507577759385E-16,0.569100145878903));
#44201=DIRECTION('',(3.66113466765132E-16,1.,1.12027918221652E-15));
#44202=DIRECTION('center_axis',(-3.66113466765132E-16,-1.,-1.12027918221652E-15));
#44203=DIRECTION('ref_axis',(-0.822268218989772,-3.36507577759385E-16,0.569100145878903));
#44204=DIRECTION('',(3.66113466765132E-16,1.,1.12027918221652E-15));
#44205=DIRECTION('center_axis',(3.66113466765132E-16,1.,1.12027918221652E-15));
#44206=DIRECTION('ref_axis',(-0.880912985579045,8.52717889674523E-16,-0.473278260474969));
#44207=DIRECTION('center_axis',(-3.66113466765132E-16,-1.,-1.12027918221652E-15));
#44208=DIRECTION('ref_axis',(-0.880912985579045,8.52717889674523E-16,-0.473278260474969));
#44209=DIRECTION('',(-3.66113466765132E-16,-1.,-1.12027918221652E-15));
#44210=DIRECTION('center_axis',(3.66113466765132E-16,1.,1.12027918221652E-15));
#44211=DIRECTION('ref_axis',(0.302722681334224,-1.1785450592138E-15,0.95307868416297));
#44212=DIRECTION('',(3.66113466765132E-16,1.,1.12027918221652E-15));
#44213=DIRECTION('center_axis',(-3.66113466765132E-16,-1.,-1.12027918221652E-15));
#44214=DIRECTION('ref_axis',(0.302722681334224,-1.1785450592138E-15,0.95307868416297));
#44215=DIRECTION('center_axis',(3.66113466765132E-16,1.,1.12027918221652E-15));
#44216=DIRECTION('ref_axis',(-0.740951125354955,-4.81061331538975E-16,0.671558954847023));
#44217=DIRECTION('',(3.66113466765132E-16,1.,1.12027918221652E-15));
#44218=DIRECTION('center_axis',(-3.66113466765132E-16,-1.,-1.12027918221652E-15));
#44219=DIRECTION('ref_axis',(-0.740951125354955,-4.81061331538975E-16,0.671558954847023));
#44220=DIRECTION('',(3.66113466765132E-16,1.,1.12027918221652E-15));
#44221=DIRECTION('center_axis',(3.66113466765132E-16,1.,1.12027918221652E-15));
#44222=DIRECTION('ref_axis',(-0.935151862070134,7.39227321122395E-16,-0.354247081663014));
#44223=DIRECTION('center_axis',(-3.66113466765132E-16,-1.,-1.12027918221652E-15));
#44224=DIRECTION('ref_axis',(-0.935151862070134,7.39227321122395E-16,-0.354247081663014));
#44225=DIRECTION('',(-3.66113466765132E-16,-1.,-1.12027918221652E-15));
#44226=DIRECTION('center_axis',(3.66113466765132E-16,1.,1.12027918221652E-15));
#44227=DIRECTION('ref_axis',(0.424534578360008,-1.16974173310301E-15,0.905411725005089));
#44228=DIRECTION('',(3.66113466765132E-16,1.,1.12027918221652E-15));
#44229=DIRECTION('center_axis',(-3.66113466765132E-16,-1.,-1.12027918221652E-15));
#44230=DIRECTION('ref_axis',(0.424534578360008,-1.16974173310301E-15,0.905411725005089));
#44231=DIRECTION('center_axis',(3.66113466765132E-16,1.,1.12027918221652E-15));
#44232=DIRECTION('ref_axis',(-0.646956152534853,-6.17383992560537E-16,0.762527203906392));
#44233=DIRECTION('',(3.66113466765132E-16,1.,1.12027918221652E-15));
#44234=DIRECTION('center_axis',(-3.66113466765132E-16,-1.,-1.12027918221652E-15));
#44235=DIRECTION('ref_axis',(-0.646956152534853,-6.17383992560537E-16,0.762527203906392));
#44236=DIRECTION('',(3.66113466765132E-16,1.,1.12027918221652E-15));
#44237=DIRECTION('center_axis',(3.66113466765132E-16,1.,1.12027918221652E-15));
#44238=DIRECTION('ref_axis',(-0.973390030928123,6.13088368153331E-16,-0.229154637067959));
#44239=DIRECTION('center_axis',(-3.66113466765132E-16,-1.,-1.12027918221652E-15));
#44240=DIRECTION('ref_axis',(-0.973390030928123,6.13088368153331E-16,-0.229154637067959));
#44241=DIRECTION('',(-3.66113466765132E-16,-1.,-1.12027918221652E-15));
#44242=DIRECTION('center_axis',(3.66113466765132E-16,1.,1.12027918221652E-15));
#44243=DIRECTION('ref_axis',(0.53908257104683,-1.14092380162514E-15,0.842252920204816));
#44244=DIRECTION('',(3.66113466765132E-16,1.,1.12027918221652E-15));
#44245=DIRECTION('center_axis',(-3.66113466765132E-16,-1.,-1.12027918221652E-15));
#44246=DIRECTION('ref_axis',(0.53908257104683,-1.14092380162514E-15,0.842252920204816));
#44247=DIRECTION('center_axis',(3.66113466765132E-16,1.,1.12027918221652E-15));
#44248=DIRECTION('ref_axis',(-0.541891580574746,-7.43143042298206E-16,0.840448401094442));
#44249=DIRECTION('',(3.66113466765132E-16,1.,1.12027918221652E-15));
#44250=DIRECTION('center_axis',(-3.66113466765132E-16,-1.,-1.12027918221652E-15));
#44251=DIRECTION('ref_axis',(-0.541891580574746,-7.43143042298206E-16,0.840448401094442));
#44252=DIRECTION('',(3.66113466765132E-16,1.,1.12027918221652E-15));
#44253=DIRECTION('center_axis',(3.66113466765132E-16,1.,1.12027918221652E-15));
#44254=DIRECTION('ref_axis',(-0.994973226482231,4.76459303224952E-16,-0.100141293099001));
#44255=DIRECTION('center_axis',(-3.66113466765132E-16,-1.,-1.12027918221652E-15));
#44256=DIRECTION('ref_axis',(-0.994973226482231,4.76459303224952E-16,-0.100141293099001));
#44257=DIRECTION('',(-3.66113466765132E-16,-1.,-1.12027918221652E-15));
#44258=DIRECTION('center_axis',(3.66113466765132E-16,1.,1.12027918221652E-15));
#44259=DIRECTION('ref_axis',(0.644406711481115,-1.09258434757764E-15,0.764682934423213));
#44260=DIRECTION('',(3.66113466765132E-16,1.,1.12027918221652E-15));
#44261=DIRECTION('center_axis',(-3.66113466765132E-16,-1.,-1.12027918221652E-15));
#44262=DIRECTION('ref_axis',(0.644406711481115,-1.09258434757764E-15,0.764682934423213));
#44263=DIRECTION('center_axis',(3.66113466765132E-16,1.,1.12027918221652E-15));
#44264=DIRECTION('ref_axis',(-0.427555093430276,-8.56186708543976E-16,0.903989293123446));
#44265=DIRECTION('',(3.66113466765132E-16,1.,1.12027918221652E-15));
#44266=DIRECTION('center_axis',(-3.66113466765132E-16,-1.,-1.12027918221652E-15));
#44267=DIRECTION('ref_axis',(-0.427555093430276,-8.56186708543976E-16,0.903989293123446));
#44268=DIRECTION('',(3.66113466765132E-16,1.,1.12027918221652E-15));
#44269=DIRECTION('center_axis',(3.66113466765132E-16,1.,1.12027918221652E-15));
#44270=DIRECTION('ref_axis',(-0.999532154272533,3.3167788751892E-16,0.0305854961592914));
#44271=DIRECTION('center_axis',(-3.66113466765132E-16,-1.,-1.12027918221652E-15));
#44272=DIRECTION('ref_axis',(-0.999532154272533,3.3167788751892E-16,0.0305854961592914));
#44273=DIRECTION('',(-3.66113466765132E-16,-1.,-1.12027918221652E-15));
#44274=DIRECTION('center_axis',(3.66113466765132E-16,1.,1.12027918221652E-15));
#44275=DIRECTION('ref_axis',(0.738704874418665,-1.02555047242146E-15,0.674029011623465));
#44276=DIRECTION('',(3.66113466765132E-16,1.,1.12027918221652E-15));
#44277=DIRECTION('center_axis',(-3.66113466765132E-16,-1.,-1.12027918221652E-15));
#44278=DIRECTION('ref_axis',(0.738704874418665,-1.02555047242146E-15,0.674029011623465));
#44279=DIRECTION('center_axis',(3.66113466765132E-16,1.,1.12027918221652E-15));
#44280=DIRECTION('ref_axis',(-0.305903020096547,-9.54580782826758E-16,0.952062677713926));
#44281=DIRECTION('',(3.66113466765132E-16,1.,1.12027918221652E-15));
#44282=DIRECTION('center_axis',(-3.66113466765132E-16,-1.,-1.12027918221652E-15));
#44283=DIRECTION('ref_axis',(-0.305903020096547,-9.54580782826758E-16,0.952062677713926));
#44284=DIRECTION('',(3.66113466765132E-16,1.,1.12027918221652E-15));
#44285=DIRECTION('center_axis',(3.66113466765132E-16,1.,1.12027918221652E-15));
#44286=DIRECTION('ref_axis',(-0.986988809780564,1.81221371198957E-16,0.160788959098396));
#44287=DIRECTION('center_axis',(-3.66113466765132E-16,-1.,-1.12027918221652E-15));
#44288=DIRECTION('ref_axis',(-0.986988809780564,1.81221371198957E-16,0.160788959098396));
#44289=DIRECTION('',(-3.66113466765132E-16,-1.,-1.12027918221652E-15));
#44290=DIRECTION('center_axis',(3.66113466765132E-16,1.,1.12027918221652E-15));
#44291=DIRECTION('ref_axis',(0.820363592147227,-9.40969144345853E-16,0.571842265558692));
#44292=DIRECTION('',(3.66113466765132E-16,1.,1.12027918221652E-15));
#44293=DIRECTION('center_axis',(-3.66113466765132E-16,-1.,-1.12027918221652E-15));
#44294=DIRECTION('ref_axis',(0.820363592147227,-9.40969144345853E-16,0.571842265558692));
#44295=DIRECTION('center_axis',(3.66113466765132E-16,1.,1.12027918221652E-15));
#44296=DIRECTION('ref_axis',(-0.179016861276626,-1.03664171525558E-15,0.983846005927078));
#44297=DIRECTION('',(3.66113466765132E-16,1.,1.12027918221652E-15));
#44298=DIRECTION('center_axis',(-3.66113466765132E-16,-1.,-1.12027918221652E-15));
#44299=DIRECTION('ref_axis',(-0.179016861276626,-1.03664171525558E-15,0.983846005927078));
#44300=DIRECTION('',(3.66113466765132E-16,1.,1.12027918221652E-15));
#44301=DIRECTION('center_axis',(3.66113466765132E-16,1.,1.12027918221652E-15));
#44302=DIRECTION('ref_axis',(-0.957557813108254,2.76641069737215E-17,0.288241278368207));
#44303=DIRECTION('center_axis',(-3.66113466765132E-16,-1.,-1.12027918221652E-15));
#44304=DIRECTION('ref_axis',(-0.957557813108254,2.76641069737215E-17,0.288241278368207));
#44305=DIRECTION('',(-3.66113466765132E-16,-1.,-1.12027918221652E-15));
#44306=DIRECTION('center_axis',(3.66113466765132E-16,1.,1.12027918221652E-15));
#44307=DIRECTION('ref_axis',(0.887985661366392,-8.40287573324551E-16,0.459871139785583));
#44308=DIRECTION('',(3.66113466765132E-16,1.,1.12027918221652E-15));
#44309=DIRECTION('center_axis',(-3.66113466765132E-16,-1.,-1.12027918221652E-15));
#44310=DIRECTION('ref_axis',(0.887985661366392,-8.40287573324551E-16,0.459871139785583));
#44311=DIRECTION('center_axis',(3.66113466765132E-16,1.,1.12027918221652E-15));
#44312=DIRECTION('ref_axis',(-0.0490676743274118,-1.100965420525E-15,0.998795456205173));
#44313=DIRECTION('',(3.66113466765132E-16,1.,1.12027918221652E-15));
#44314=DIRECTION('center_axis',(-3.66113466765132E-16,-1.,-1.12027918221652E-15));
#44315=DIRECTION('ref_axis',(-0.0490676743274118,-1.100965420525E-15,0.998795456205173));
#44316=DIRECTION('',(3.66113466765132E-16,1.,1.12027918221652E-15));
#44317=DIRECTION('center_axis',(3.66113466765132E-16,1.,1.12027918221652E-15));
#44318=DIRECTION('ref_axis',(-0.91174273676848,-1.26366497791772E-16,0.410761709449557));
#44319=DIRECTION('center_axis',(-3.66113466765132E-16,-1.,-1.12027918221652E-15));
#44320=DIRECTION('ref_axis',(-0.91174273676848,-1.26366497791772E-16,0.410761709449557));
#44321=DIRECTION('',(-3.66113466765132E-16,-1.,-1.12027918221652E-15));
#44322=DIRECTION('center_axis',(3.66113466765132E-16,1.,1.12027918221652E-15));
#44323=DIRECTION('ref_axis',(0.940414049723441,-7.25228448951937E-16,0.340031491310375));
#44324=DIRECTION('',(3.66113466765132E-16,1.,1.12027918221652E-15));
#44325=DIRECTION('center_axis',(-3.66113466765132E-16,-1.,-1.12027918221652E-15));
#44326=DIRECTION('ref_axis',(0.940414049723441,-7.25228448951937E-16,0.340031491310375));
#44327=DIRECTION('center_axis',(3.66113466765132E-16,1.,1.12027918221652E-15));
#44328=DIRECTION('ref_axis',(0.0817210741336744,-1.14645130220395E-15,0.99665523930918));
#44329=DIRECTION('',(3.66113466765132E-16,1.,1.12027918221652E-15));
#44330=DIRECTION('center_axis',(-3.66113466765132E-16,-1.,-1.12027918221652E-15));
#44331=DIRECTION('ref_axis',(0.0817210741336744,-1.14645130220395E-15,0.99665523930918));
#44332=DIRECTION('',(3.66113466765132E-16,1.,1.12027918221652E-15));
#44333=DIRECTION('center_axis',(3.66113466765132E-16,1.,1.12027918221652E-15));
#44334=DIRECTION('ref_axis',(-0.850327489419754,-2.78234936744637E-16,0.526253893797564));
#44335=DIRECTION('center_axis',(-3.66113466765132E-16,-1.,-1.12027918221652E-15));
#44336=DIRECTION('ref_axis',(-0.850327489419754,-2.78234936744637E-16,0.526253893797564));
#44337=DIRECTION('',(-3.66113466765132E-16,-1.,-1.12027918221652E-15));
#44338=DIRECTION('center_axis',(3.66113466765132E-16,1.,1.12027918221652E-15));
#44339=DIRECTION('ref_axis',(0.976751692957689,-5.97760464746442E-16,0.214373809744306));
#44340=DIRECTION('',(3.66113466765132E-16,1.,1.12027918221652E-15));
#44341=DIRECTION('center_axis',(-3.66113466765132E-16,-1.,-1.12027918221652E-15));
#44342=DIRECTION('ref_axis',(0.976751692957689,-5.97760464746442E-16,0.214373809744306));
#44343=DIRECTION('center_axis',(3.66113466765132E-16,1.,1.12027918221652E-15));
#44344=DIRECTION('ref_axis',(0.211111552358972,-1.17232108424584E-15,0.97746197494357));
#44345=DIRECTION('',(3.66113466765132E-16,1.,1.12027918221652E-15));
#44346=DIRECTION('center_axis',(-3.66113466765132E-16,-1.,-1.12027918221652E-15));
#44347=DIRECTION('ref_axis',(0.211111552358972,-1.17232108424584E-15,0.97746197494357));
#44348=DIRECTION('',(3.66113466765132E-16,1.,1.12027918221652E-15));
#44349=DIRECTION('center_axis',(3.66113466765132E-16,1.,1.12027918221652E-15));
#44350=DIRECTION('ref_axis',(-0.774362902971737,-4.25342698788503E-16,0.632741728117551));
#44351=DIRECTION('center_axis',(-3.66113466765132E-16,-1.,-1.12027918221652E-15));
#44352=DIRECTION('ref_axis',(-0.774362902971737,-4.25342698788503E-16,0.632741728117551));
#44353=DIRECTION('',(-3.66113466765132E-16,-1.,-1.12027918221652E-15));
#44354=DIRECTION('center_axis',(3.66113466765132E-16,1.,1.12027918221652E-15));
#44355=DIRECTION('ref_axis',(0.996376843918701,-4.60064633258624E-16,0.0850481328578616));
#44356=DIRECTION('',(3.66113466765132E-16,1.,1.12027918221652E-15));
#44357=DIRECTION('center_axis',(-3.66113466765132E-16,-1.,-1.12027918221652E-15));
#44358=DIRECTION('ref_axis',(0.996376843918701,-4.60064633258624E-16,0.0850481328578616));
#44359=DIRECTION('center_axis',(3.66113466765132E-16,1.,1.12027918221652E-15));
#44360=DIRECTION('ref_axis',(0.336889853392226,-1.17813212750748E-15,0.941544065183018));
#44361=DIRECTION('',(3.66113466765132E-16,1.,1.12027918221652E-15));
#44362=DIRECTION('center_axis',(-3.66113466765132E-16,-1.,-1.12027918221652E-15));
#44363=DIRECTION('ref_axis',(0.336889853392226,-1.17813212750748E-15,0.941544065183018));
#44364=DIRECTION('',(3.66113466765132E-16,1.,1.12027918221652E-15));
#44365=DIRECTION('center_axis',(3.66113466765132E-16,1.,1.12027918221652E-15));
#44366=DIRECTION('ref_axis',(-0.685148752559916,-5.65172729328823E-16,0.728403176040296));
#44367=DIRECTION('center_axis',(-3.66113466765132E-16,-1.,-1.12027918221652E-15));
#44368=DIRECTION('ref_axis',(-0.685148752559916,-5.65172729328823E-16,0.728403176040296));
#44369=DIRECTION('',(-3.66113466765132E-16,-1.,-1.12027918221652E-15));
#44370=DIRECTION('center_axis',(3.66113466765132E-16,1.,1.12027918221652E-15));
#44371=DIRECTION('ref_axis',(0.998953710832413,-3.14496968341737E-16,-0.0457327411615765));
#44372=DIRECTION('',(3.66113466765132E-16,1.,1.12027918221652E-15));
#44373=DIRECTION('center_axis',(-3.66113466765132E-16,-1.,-1.12027918221652E-15));
#44374=DIRECTION('ref_axis',(0.998953710832413,-3.14496968341737E-16,-0.0457327411615765));
#44375=DIRECTION('center_axis',(3.66113466765132E-16,1.,1.12027918221652E-15));
#44376=DIRECTION('ref_axis',(0.456903875630426,-1.16378500342752E-15,0.889516075421853));
#44377=DIRECTION('',(3.66113466765132E-16,1.,1.12027918221652E-15));
#44378=DIRECTION('center_axis',(-3.66113466765132E-16,-1.,-1.12027918221652E-15));
#44379=DIRECTION('ref_axis',(0.456903875630426,-1.16378500342752E-15,0.889516075421853));
#44380=DIRECTION('',(3.66113466765132E-16,1.,1.12027918221652E-15));
#44381=DIRECTION('center_axis',(3.66113466765132E-16,1.,1.12027918221652E-15));
#44382=DIRECTION('ref_axis',(-0.584211517032673,-6.95332497774842E-16,0.811601443669479));
#44383=DIRECTION('center_axis',(-3.66113466765132E-16,-1.,-1.12027918221652E-15));
#44384=DIRECTION('ref_axis',(-0.584211517032673,-6.95332497774842E-16,0.811601443669479));
#44385=DIRECTION('',(-3.66113466765132E-16,-1.,-1.12027918221652E-15));
#44386=DIRECTION('center_axis',(3.66113466765132E-16,1.,1.12027918221652E-15));
#44387=DIRECTION('ref_axis',(0.98443820279149,-1.63548173101491E-16,-0.175731115300228));
#44388=DIRECTION('',(3.66113466765132E-16,1.,1.12027918221652E-15));
#44389=DIRECTION('center_axis',(-3.66113466765132E-16,-1.,-1.12027918221652E-15));
#44390=DIRECTION('ref_axis',(0.98443820279149,-1.63548173101491E-16,-0.175731115300228));
#44391=DIRECTION('center_axis',(3.66113466765132E-16,1.,1.12027918221652E-15));
#44392=DIRECTION('ref_axis',(0.569100145878903,-1.12952519527676E-15,0.822268218989772));
#44393=DIRECTION('',(3.66113466765132E-16,1.,1.12027918221652E-15));
#44394=DIRECTION('center_axis',(-3.66113466765132E-16,-1.,-1.12027918221652E-15));
#44395=DIRECTION('ref_axis',(0.569100145878903,-1.12952519527676E-15,0.822268218989772));
#44396=DIRECTION('',(3.66113466765132E-16,1.,1.12027918221652E-15));
#44397=DIRECTION('center_axis',(3.66113466765132E-16,1.,1.12027918221652E-15));
#44398=DIRECTION('ref_axis',(-0.473278260474969,-8.13594934401345E-16,0.880912985579045));
#44399=DIRECTION('center_axis',(-3.66113466765132E-16,-1.,-1.12027918221652E-15));
#44400=DIRECTION('ref_axis',(-0.473278260474969,-8.13594934401345E-16,0.880912985579045));
#44401=DIRECTION('',(-3.66113466765132E-16,-1.,-1.12027918221652E-15));
#44402=DIRECTION('center_axis',(3.66113466765132E-16,1.,1.12027918221652E-15));
#44403=DIRECTION('ref_axis',(0.95307868416297,-9.80102327535809E-18,-0.302722681334224));
#44404=DIRECTION('',(3.66113466765132E-16,1.,1.12027918221652E-15));
#44405=DIRECTION('center_axis',(-3.66113466765132E-16,-1.,-1.12027918221652E-15));
#44406=DIRECTION('ref_axis',(0.95307868416297,-9.80102327535809E-18,-0.302722681334224));
#44407=DIRECTION('center_axis',(3.66113466765132E-16,1.,1.12027918221652E-15));
#44408=DIRECTION('ref_axis',(0.671558954847023,-1.07593889787127E-15,0.740951125354955));
#44409=DIRECTION('',(3.66113466765132E-16,1.,1.12027918221652E-15));
#44410=DIRECTION('center_axis',(-3.66113466765132E-16,-1.,-1.12027918221652E-15));
#44411=DIRECTION('ref_axis',(0.671558954847023,-1.07593889787127E-15,0.740951125354955));
#44412=DIRECTION('',(3.66113466765132E-16,1.,1.12027918221652E-15));
#44413=DIRECTION('center_axis',(3.66113466765132E-16,1.,1.12027918221652E-15));
#44414=DIRECTION('ref_axis',(-0.354247081663014,-9.17936536129109E-16,0.935151862070134));
#44415=DIRECTION('center_axis',(-3.66113466765132E-16,-1.,-1.12027918221652E-15));
#44416=DIRECTION('ref_axis',(-0.354247081663014,-9.17936536129109E-16,0.935151862070134));
#44417=DIRECTION('',(-3.66113466765132E-16,-1.,-1.12027918221652E-15));
#44418=DIRECTION('center_axis',(3.66113466765132E-16,1.,1.12027918221652E-15));
#44419=DIRECTION('ref_axis',(0.905411725005089,1.44113824776374E-16,-0.424534578360008));
#44420=DIRECTION('',(3.66113466765132E-16,1.,1.12027918221652E-15));
#44421=DIRECTION('center_axis',(-3.66113466765132E-16,-1.,-1.12027918221652E-15));
#44422=DIRECTION('ref_axis',(0.905411725005089,1.44113824776374E-16,-0.424534578360008));
#44423=DIRECTION('center_axis',(3.66113466765132E-16,1.,1.12027918221652E-15));
#44424=DIRECTION('ref_axis',(0.762527203906392,-1.00394298761658E-15,0.646956152534853));
#44425=DIRECTION('',(3.66113466765132E-16,1.,1.12027918221652E-15));
#44426=DIRECTION('center_axis',(-3.66113466765132E-16,-1.,-1.12027918221652E-15));
#44427=DIRECTION('ref_axis',(0.762527203906392,-1.00394298761658E-15,0.646956152534853));
#44428=DIRECTION('',(3.66113466765132E-16,1.,1.12027918221652E-15));
#44429=DIRECTION('center_axis',(3.66113466765132E-16,1.,1.12027918221652E-15));
#44430=DIRECTION('ref_axis',(-0.229154637067958,-1.00657198922362E-15,0.973390030928123));
#44431=DIRECTION('center_axis',(-3.66113466765132E-16,-1.,-1.12027918221652E-15));
#44432=DIRECTION('ref_axis',(-0.229154637067958,-1.00657198922362E-15,0.973390030928123));
#44433=DIRECTION('',(-3.66113466765132E-16,-1.,-1.12027918221652E-15));
#44434=DIRECTION('center_axis',(3.66113466765132E-16,1.,1.12027918221652E-15));
#44435=DIRECTION('ref_axis',(0.842252920204816,2.9556284533028E-16,-0.53908257104683));
#44436=DIRECTION('',(3.66113466765132E-16,1.,1.12027918221652E-15));
#44437=DIRECTION('center_axis',(-3.66113466765132E-16,-1.,-1.12027918221652E-15));
#44438=DIRECTION('ref_axis',(0.842252920204816,2.9556284533028E-16,-0.53908257104683));
#44439=DIRECTION('center_axis',(3.66113466765132E-16,1.,1.12027918221652E-15));
#44440=DIRECTION('ref_axis',(0.840448401094441,-9.14769334498193E-16,0.541891580574747));
#44441=DIRECTION('',(3.66113466765132E-16,1.,1.12027918221652E-15));
#44442=DIRECTION('center_axis',(-3.66113466765132E-16,-1.,-1.12027918221652E-15));
#44443=DIRECTION('ref_axis',(0.840448401094441,-9.14769334498193E-16,0.541891580574747));
#44444=DIRECTION('',(3.66113466765132E-16,1.,1.12027918221652E-15));
#44445=DIRECTION('center_axis',(3.66113466765132E-16,1.,1.12027918221652E-15));
#44446=DIRECTION('ref_axis',(-0.100141293099002,-1.07798471650803E-15,0.994973226482231));
#44447=DIRECTION('center_axis',(-3.66113466765132E-16,-1.,-1.12027918221652E-15));
#44448=DIRECTION('ref_axis',(-0.100141293099002,-1.07798471650803E-15,0.994973226482231));
#44449=DIRECTION('',(-3.66113466765132E-16,-1.,-1.12027918221652E-15));
#44450=DIRECTION('center_axis',(3.66113466765132E-16,1.,1.12027918221652E-15));
#44451=DIRECTION('ref_axis',(0.764682934423213,4.41954703655085E-16,-0.644406711481115));
#44452=DIRECTION('',(3.66113466765132E-16,1.,1.12027918221652E-15));
#44453=DIRECTION('center_axis',(-3.66113466765132E-16,-1.,-1.12027918221652E-15));
#44454=DIRECTION('ref_axis',(0.764682934423213,4.41954703655085E-16,-0.644406711481115));
#44455=DIRECTION('center_axis',(3.66113466765132E-16,1.,1.12027918221652E-15));
#44456=DIRECTION('ref_axis',(0.903989293123446,-8.09943724444564E-16,0.427555093430276));
#44457=DIRECTION('',(3.66113466765132E-16,1.,1.12027918221652E-15));
#44458=DIRECTION('center_axis',(-3.66113466765132E-16,-1.,-1.12027918221652E-15));
#44459=DIRECTION('ref_axis',(0.903989293123446,-8.09943724444564E-16,0.427555093430276));
#44460=DIRECTION('',(3.66113466765132E-16,1.,1.12027918221652E-15));
#44461=DIRECTION('center_axis',(3.66113466765132E-16,1.,1.12027918221652E-15));
#44462=DIRECTION('ref_axis',(0.0305854961592909,-1.13095282641916E-15,0.999532154272533));
#44463=DIRECTION('center_axis',(-3.66113466765132E-16,-1.,-1.12027918221652E-15));
#44464=DIRECTION('ref_axis',(0.0305854961592909,-1.13095282641916E-15,0.999532154272533));
#44465=DIRECTION('',(-3.66113466765132E-16,-1.,-1.12027918221652E-15));
#44466=DIRECTION('center_axis',(3.66113466765132E-16,1.,1.12027918221652E-15));
#44467=DIRECTION('ref_axis',(0.674029011623465,5.80784594467357E-16,-0.738704874418665));
#44468=DIRECTION('',(3.66113466765132E-16,1.,1.12027918221652E-15));
#44469=DIRECTION('center_axis',(-3.66113466765132E-16,-1.,-1.12027918221652E-15));
#44470=DIRECTION('ref_axis',(0.674029011623465,5.80784594467357E-16,-0.738704874418665));
#44471=DIRECTION('center_axis',(3.66113466765132E-16,1.,1.12027918221652E-15));
#44472=DIRECTION('ref_axis',(0.952062677713926,-6.91259752706864E-16,0.305903020096547));
#44473=DIRECTION('',(3.66113466765132E-16,1.,1.12027918221652E-15));
#44474=DIRECTION('center_axis',(-3.66113466765132E-16,-1.,-1.12027918221652E-15));
#44475=DIRECTION('ref_axis',(0.952062677713926,-6.91259752706864E-16,0.305903020096547));
#44476=DIRECTION('',(3.66113466765132E-16,1.,1.12027918221652E-15));
#44477=DIRECTION('center_axis',(3.66113466765132E-16,1.,1.12027918221652E-15));
#44478=DIRECTION('ref_axis',(0.160788959098396,-1.1645700199109E-15,0.986988809780564));
#44479=DIRECTION('center_axis',(-3.66113466765132E-16,-1.,-1.12027918221652E-15));
#44480=DIRECTION('ref_axis',(0.160788959098396,-1.1645700199109E-15,0.986988809780564));
#44481=DIRECTION('',(-3.66113466765132E-16,-1.,-1.12027918221652E-15));
#44482=DIRECTION('center_axis',(3.66113466765132E-16,1.,1.12027918221652E-15));
#44483=DIRECTION('ref_axis',(0.571842265558692,7.09677099844383E-16,-0.820363592147227));
#44484=DIRECTION('',(3.66113466765132E-16,1.,1.12027918221652E-15));
#44485=DIRECTION('center_axis',(-3.66113466765132E-16,-1.,-1.12027918221652E-15));
#44486=DIRECTION('ref_axis',(0.571842265558692,7.09677099844383E-16,-0.820363592147227));
#44487=DIRECTION('center_axis',(3.66113466765132E-16,1.,1.12027918221652E-15));
#44488=DIRECTION('ref_axis',(0.983846005927078,-5.60748134946939E-16,0.179016861276626));
#44489=DIRECTION('',(3.66113466765132E-16,1.,1.12027918221652E-15));
#44490=DIRECTION('center_axis',(-3.66113466765132E-16,-1.,-1.12027918221652E-15));
#44491=DIRECTION('ref_axis',(0.983846005927078,-5.60748134946939E-16,0.179016861276626));
#44492=DIRECTION('',(3.66113466765132E-16,1.,1.12027918221652E-15));
#44493=DIRECTION('center_axis',(3.66113466765132E-16,1.,1.12027918221652E-15));
#44494=DIRECTION('ref_axis',(0.288241278368206,-1.17826109748215E-15,0.957557813108254));
#44495=DIRECTION('center_axis',(-3.66113466765132E-16,-1.,-1.12027918221652E-15));
#44496=DIRECTION('ref_axis',(0.288241278368206,-1.17826109748215E-15,0.957557813108254));
#44497=DIRECTION('',(-3.66113466765132E-16,-1.,-1.12027918221652E-15));
#44498=DIRECTION('center_axis',(3.66113466765132E-16,1.,1.12027918221652E-15));
#44499=DIRECTION('ref_axis',(0.459871139785583,8.26426833283406E-16,-0.887985661366392));
#44500=DIRECTION('',(3.66113466765132E-16,1.,1.12027918221652E-15));
#44501=DIRECTION('center_axis',(-3.66113466765132E-16,-1.,-1.12027918221652E-15));
#44502=DIRECTION('ref_axis',(0.459871139785583,8.26426833283406E-16,-0.887985661366392));
#44503=DIRECTION('center_axis',(3.66113466765132E-16,1.,1.12027918221652E-15));
#44504=DIRECTION('ref_axis',(0.998795456205173,-4.20641961129317E-16,0.0490676743274118));
#44505=DIRECTION('',(3.66113466765132E-16,1.,1.12027918221652E-15));
#44506=DIRECTION('center_axis',(-3.66113466765132E-16,-1.,-1.12027918221652E-15));
#44507=DIRECTION('ref_axis',(0.998795456205173,-4.20641961129317E-16,0.0490676743274118));
#44508=DIRECTION('',(3.66113466765132E-16,1.,1.12027918221652E-15));
#44509=DIRECTION('center_axis',(3.66113466765132E-16,1.,1.12027918221652E-15));
#44510=DIRECTION('ref_axis',(0.410761709449557,-1.17179180099979E-15,0.91174273676848));
#44511=DIRECTION('center_axis',(-3.66113466765132E-16,-1.,-1.12027918221652E-15));
#44512=DIRECTION('ref_axis',(0.410761709449557,-1.17179180099979E-15,0.91174273676848));
#44513=DIRECTION('',(-3.66113466765132E-16,-1.,-1.12027918221652E-15));
#44514=DIRECTION('center_axis',(3.66113466765132E-16,1.,1.12027918221652E-15));
#44515=DIRECTION('ref_axis',(0.340031491310375,9.29036174476144E-16,-0.940414049723441));
#44516=DIRECTION('',(3.66113466765132E-16,1.,1.12027918221652E-15));
#44517=DIRECTION('center_axis',(-3.66113466765132E-16,-1.,-1.12027918221652E-15));
#44518=DIRECTION('ref_axis',(0.340031491310375,9.29036174476144E-16,-0.940414049723441));
#44519=DIRECTION('center_axis',(3.66113466765132E-16,1.,1.12027918221652E-15));
#44520=DIRECTION('ref_axis',(0.99665523930918,-2.73338486732788E-16,-0.0817210741336743));
#44521=DIRECTION('',(3.66113466765132E-16,1.,1.12027918221652E-15));
#44522=DIRECTION('center_axis',(-3.66113466765132E-16,-1.,-1.12027918221652E-15));
#44523=DIRECTION('ref_axis',(0.99665523930918,-2.73338486732788E-16,-0.0817210741336743));
#44524=DIRECTION('',(3.66113466765132E-16,1.,1.12027918221652E-15));
#44525=DIRECTION('center_axis',(3.66113466765132E-16,1.,1.12027918221652E-15));
#44526=DIRECTION('ref_axis',(0.526253893797564,-1.14527282192027E-15,0.850327489419754));
#44527=DIRECTION('center_axis',(-3.66113466765132E-16,-1.,-1.12027918221652E-15));
#44528=DIRECTION('ref_axis',(0.526253893797564,-1.14527282192027E-15,0.850327489419754));
#44529=DIRECTION('',(-3.66113466765132E-16,-1.,-1.12027918221652E-15));
#44530=DIRECTION('center_axis',(3.66113466765132E-16,1.,1.12027918221652E-15));
#44531=DIRECTION('ref_axis',(0.214373809744306,1.01574944914611E-15,-0.976751692957689));
#44532=DIRECTION('',(3.66113466765132E-16,1.,1.12027918221652E-15));
#44533=DIRECTION('center_axis',(-3.66113466765132E-16,-1.,-1.12027918221652E-15));
#44534=DIRECTION('ref_axis',(0.214373809744306,1.01574944914611E-15,-0.976751692957689));
#44535=DIRECTION('center_axis',(3.66113466765132E-16,1.,1.12027918221652E-15));
#44536=DIRECTION('ref_axis',(0.977461974943571,-1.21358115044515E-16,-0.211111552358971));
#44537=DIRECTION('',(3.66113466765132E-16,1.,1.12027918221652E-15));
#44538=DIRECTION('center_axis',(-3.66113466765132E-16,-1.,-1.12027918221652E-15));
#44539=DIRECTION('ref_axis',(0.977461974943571,-1.21358115044515E-16,-0.211111552358971));
#44540=DIRECTION('',(3.66113466765132E-16,1.,1.12027918221652E-15));
#44541=DIRECTION('center_axis',(3.66113466765132E-16,1.,1.12027918221652E-15));
#44542=DIRECTION('ref_axis',(0.63274172811755,-1.09915790732807E-15,0.774362902971737));
#44543=DIRECTION('center_axis',(-3.66113466765132E-16,-1.,-1.12027918221652E-15));
#44544=DIRECTION('ref_axis',(0.63274172811755,-1.09915790732807E-15,0.774362902971737));
#44545=DIRECTION('',(-3.66113466765132E-16,-1.,-1.12027918221652E-15));
#44546=DIRECTION('center_axis',(3.66113466765132E-16,1.,1.12027918221652E-15));
#44547=DIRECTION('ref_axis',(0.0850481328578621,1.08508296912223E-15,-0.996376843918701));
#44548=DIRECTION('',(3.66113466765132E-16,1.,1.12027918221652E-15));
#44549=DIRECTION('center_axis',(-3.66113466765132E-16,-1.,-1.12027918221652E-15));
#44550=DIRECTION('ref_axis',(0.0850481328578621,1.08508296912223E-15,-0.996376843918701));
#44551=DIRECTION('center_axis',(3.66113466765132E-16,1.,1.12027918221652E-15));
#44552=DIRECTION('ref_axis',(0.941544065183019,3.2698727638996E-17,-0.336889853392226));
#44553=DIRECTION('',(3.66113466765132E-16,1.,1.12027918221652E-15));
#44554=DIRECTION('center_axis',(-3.66113466765132E-16,-1.,-1.12027918221652E-15));
#44555=DIRECTION('ref_axis',(0.941544065183019,3.2698727638996E-17,-0.336889853392226));
#44556=DIRECTION('',(3.66113466765132E-16,1.,1.12027918221652E-15));
#44557=DIRECTION('center_axis',(3.66113466765132E-16,1.,1.12027918221652E-15));
#44558=DIRECTION('ref_axis',(0.728403176040296,-1.03423609619734E-15,0.685148752559917));
#44559=DIRECTION('center_axis',(-3.66113466765132E-16,-1.,-1.12027918221652E-15));
#44560=DIRECTION('ref_axis',(0.728403176040296,-1.03423609619734E-15,0.685148752559917));
#44561=DIRECTION('',(-3.66113466765132E-16,-1.,-1.12027918221652E-15));
#44562=DIRECTION('center_axis',(3.66113466765132E-16,1.,1.12027918221652E-15));
#44563=DIRECTION('ref_axis',(-0.0457327411615761,1.13585041865483E-15,-0.998953710832413));
#44564=DIRECTION('',(3.66113466765132E-16,1.,1.12027918221652E-15));
#44565=DIRECTION('center_axis',(-3.66113466765132E-16,-1.,-1.12027918221652E-15));
#44566=DIRECTION('ref_axis',(-0.0457327411615761,1.13585041865483E-15,-0.998953710832413));
#44567=DIRECTION('center_axis',(3.66113466765132E-16,1.,1.12027918221652E-15));
#44568=DIRECTION('ref_axis',(0.889516075421853,1.86196086026803E-16,-0.456903875630426));
#44569=DIRECTION('',(3.66113466765132E-16,1.,1.12027918221652E-15));
#44570=DIRECTION('center_axis',(-3.66113466765132E-16,-1.,-1.12027918221652E-15));
#44571=DIRECTION('ref_axis',(0.889516075421853,1.86196086026803E-16,-0.456903875630426));
#44572=DIRECTION('',(3.66113466765132E-16,1.,1.12027918221652E-15));
#44573=DIRECTION('center_axis',(3.66113466765132E-16,1.,1.12027918221652E-15));
#44574=DIRECTION('ref_axis',(0.811601443669479,-9.51618218716256E-16,0.584211517032674));
#44575=DIRECTION('center_axis',(-3.66113466765132E-16,-1.,-1.12027918221652E-15));
#44576=DIRECTION('ref_axis',(0.811601443669479,-9.51618218716256E-16,0.584211517032674));
#44577=DIRECTION('',(-3.66113466765132E-16,-1.,-1.12027918221652E-15));
#44578=DIRECTION('center_axis',(3.66113466765132E-16,1.,1.12027918221652E-15));
#44579=DIRECTION('ref_axis',(-0.175731115300228,1.16718315260702E-15,-0.98443820279149));
#44580=DIRECTION('',(3.66113466765132E-16,1.,1.12027918221652E-15));
#44581=DIRECTION('center_axis',(-3.66113466765132E-16,-1.,-1.12027918221652E-15));
#44582=DIRECTION('ref_axis',(-0.175731115300228,1.16718315260702E-15,-0.98443820279149));
#44583=DIRECTION('center_axis',(3.66113466765132E-16,1.,1.12027918221652E-15));
#44584=DIRECTION('ref_axis',(0.822268218989772,3.36507577759385E-16,-0.569100145878903));
#44585=DIRECTION('',(3.66113466765132E-16,1.,1.12027918221652E-15));
#44586=DIRECTION('center_axis',(-3.66113466765132E-16,-1.,-1.12027918221652E-15));
#44587=DIRECTION('ref_axis',(0.822268218989772,3.36507577759385E-16,-0.569100145878903));
#44588=DIRECTION('',(3.66113466765132E-16,1.,1.12027918221652E-15));
#44589=DIRECTION('center_axis',(3.66113466765132E-16,1.,1.12027918221652E-15));
#44590=DIRECTION('ref_axis',(0.880912985579045,-8.52717889674523E-16,0.473278260474969));
#44591=DIRECTION('center_axis',(-3.66113466765132E-16,-1.,-1.12027918221652E-15));
#44592=DIRECTION('ref_axis',(0.880912985579045,-8.52717889674523E-16,0.473278260474969));
#44593=DIRECTION('',(-3.66113466765132E-16,-1.,-1.12027918221652E-15));
#44594=DIRECTION('center_axis',(3.66113466765132E-16,1.,1.12027918221652E-15));
#44595=DIRECTION('ref_axis',(-0.302722681334224,1.1785450592138E-15,-0.95307868416297));
#44596=DIRECTION('',(3.66113466765132E-16,1.,1.12027918221652E-15));
#44597=DIRECTION('center_axis',(-3.66113466765132E-16,-1.,-1.12027918221652E-15));
#44598=DIRECTION('ref_axis',(-0.302722681334224,1.1785450592138E-15,-0.95307868416297));
#44599=DIRECTION('center_axis',(3.66113466765132E-16,1.,1.12027918221652E-15));
#44600=DIRECTION('ref_axis',(0.740951125354955,4.81061331538975E-16,-0.671558954847023));
#44601=DIRECTION('',(3.66113466765132E-16,1.,1.12027918221652E-15));
#44602=DIRECTION('center_axis',(-3.66113466765132E-16,-1.,-1.12027918221652E-15));
#44603=DIRECTION('ref_axis',(0.740951125354955,4.81061331538975E-16,-0.671558954847023));
#44604=DIRECTION('',(3.66113466765132E-16,1.,1.12027918221652E-15));
#44605=DIRECTION('center_axis',(3.66113466765132E-16,1.,1.12027918221652E-15));
#44606=DIRECTION('ref_axis',(0.935151862070134,-7.39227321122395E-16,0.354247081663014));
#44607=DIRECTION('center_axis',(-3.66113466765132E-16,-1.,-1.12027918221652E-15));
#44608=DIRECTION('ref_axis',(0.935151862070134,-7.39227321122395E-16,0.354247081663014));
#44609=DIRECTION('',(-3.66113466765132E-16,-1.,-1.12027918221652E-15));
#44610=DIRECTION('center_axis',(3.66113466765132E-16,1.,1.12027918221652E-15));
#44611=DIRECTION('ref_axis',(-0.424534578360008,1.16974173310301E-15,-0.905411725005089));
#44612=DIRECTION('',(3.66113466765132E-16,1.,1.12027918221652E-15));
#44613=DIRECTION('center_axis',(-3.66113466765132E-16,-1.,-1.12027918221652E-15));
#44614=DIRECTION('ref_axis',(-0.424534578360008,1.16974173310301E-15,-0.905411725005089));
#44615=DIRECTION('center_axis',(3.66113466765132E-16,1.,1.12027918221652E-15));
#44616=DIRECTION('ref_axis',(0.646956152534853,6.17383992560536E-16,-0.762527203906392));
#44617=DIRECTION('',(3.66113466765132E-16,1.,1.12027918221652E-15));
#44618=DIRECTION('center_axis',(-3.66113466765132E-16,-1.,-1.12027918221652E-15));
#44619=DIRECTION('ref_axis',(0.646956152534853,6.17383992560536E-16,-0.762527203906392));
#44620=DIRECTION('',(3.66113466765132E-16,1.,1.12027918221652E-15));
#44621=DIRECTION('center_axis',(3.66113466765132E-16,1.,1.12027918221652E-15));
#44622=DIRECTION('ref_axis',(0.973390030928123,-6.13088368153331E-16,0.229154637067959));
#44623=DIRECTION('center_axis',(-3.66113466765132E-16,-1.,-1.12027918221652E-15));
#44624=DIRECTION('ref_axis',(0.973390030928123,-6.13088368153331E-16,0.229154637067959));
#44625=DIRECTION('',(-3.66113466765132E-16,-1.,-1.12027918221652E-15));
#44626=DIRECTION('center_axis',(3.66113466765132E-16,1.,1.12027918221652E-15));
#44627=DIRECTION('ref_axis',(-0.53908257104683,1.14092380162514E-15,-0.842252920204816));
#44628=DIRECTION('',(3.66113466765132E-16,1.,1.12027918221652E-15));
#44629=DIRECTION('center_axis',(-3.66113466765132E-16,-1.,-1.12027918221652E-15));
#44630=DIRECTION('ref_axis',(-0.53908257104683,1.14092380162514E-15,-0.842252920204816));
#44631=DIRECTION('center_axis',(3.66113466765132E-16,1.,1.12027918221652E-15));
#44632=DIRECTION('ref_axis',(0.541891580574746,7.43143042298206E-16,-0.840448401094442));
#44633=DIRECTION('',(3.66113466765132E-16,1.,1.12027918221652E-15));
#44634=DIRECTION('center_axis',(-3.66113466765132E-16,-1.,-1.12027918221652E-15));
#44635=DIRECTION('ref_axis',(0.541891580574746,7.43143042298206E-16,-0.840448401094442));
#44636=DIRECTION('',(3.66113466765132E-16,1.,1.12027918221652E-15));
#44637=DIRECTION('center_axis',(3.66113466765132E-16,1.,1.12027918221652E-15));
#44638=DIRECTION('ref_axis',(0.994973226482231,-4.76459303224953E-16,0.100141293099002));
#44639=DIRECTION('center_axis',(-3.66113466765132E-16,-1.,-1.12027918221652E-15));
#44640=DIRECTION('ref_axis',(0.994973226482231,-4.76459303224953E-16,0.100141293099002));
#44641=DIRECTION('',(-3.66113466765132E-16,-1.,-1.12027918221652E-15));
#44642=DIRECTION('center_axis',(3.66113466765132E-16,1.,1.12027918221652E-15));
#44643=DIRECTION('ref_axis',(-0.644406711481115,1.09258434757764E-15,-0.764682934423213));
#44644=DIRECTION('',(3.66113466765132E-16,1.,1.12027918221652E-15));
#44645=DIRECTION('center_axis',(-3.66113466765132E-16,-1.,-1.12027918221652E-15));
#44646=DIRECTION('ref_axis',(-0.644406711481115,1.09258434757764E-15,-0.764682934423213));
#44647=DIRECTION('center_axis',(3.66113466765132E-16,1.,1.12027918221652E-15));
#44648=DIRECTION('ref_axis',(0.427555093430276,8.56186708543976E-16,-0.903989293123446));
#44649=DIRECTION('',(3.66113466765132E-16,1.,1.12027918221652E-15));
#44650=DIRECTION('center_axis',(-3.66113466765132E-16,-1.,-1.12027918221652E-15));
#44651=DIRECTION('ref_axis',(0.427555093430276,8.56186708543976E-16,-0.903989293123446));
#44652=DIRECTION('',(3.66113466765132E-16,1.,1.12027918221652E-15));
#44653=DIRECTION('center_axis',(3.66113466765132E-16,1.,1.12027918221652E-15));
#44654=DIRECTION('ref_axis',(0.999532154272533,-3.31677887518921E-16,-0.0305854961592909));
#44655=DIRECTION('center_axis',(-3.66113466765132E-16,-1.,-1.12027918221652E-15));
#44656=DIRECTION('ref_axis',(0.999532154272533,-3.31677887518921E-16,-0.0305854961592909));
#44657=DIRECTION('',(-3.66113466765132E-16,-1.,-1.12027918221652E-15));
#44658=DIRECTION('center_axis',(3.66113466765132E-16,1.,1.12027918221652E-15));
#44659=DIRECTION('ref_axis',(-0.738704874418665,1.02555047242146E-15,-0.674029011623465));
#44660=DIRECTION('',(3.66113466765132E-16,1.,1.12027918221652E-15));
#44661=DIRECTION('center_axis',(-3.66113466765132E-16,-1.,-1.12027918221652E-15));
#44662=DIRECTION('ref_axis',(-0.738704874418665,1.02555047242146E-15,-0.674029011623465));
#44663=DIRECTION('center_axis',(3.66113466765132E-16,1.,1.12027918221652E-15));
#44664=DIRECTION('ref_axis',(0.305903020096548,9.54580782826757E-16,-0.952062677713926));
#44665=DIRECTION('',(3.66113466765132E-16,1.,1.12027918221652E-15));
#44666=DIRECTION('center_axis',(-3.66113466765132E-16,-1.,-1.12027918221652E-15));
#44667=DIRECTION('ref_axis',(0.305903020096548,9.54580782826757E-16,-0.952062677713926));
#44668=DIRECTION('',(3.66113466765132E-16,1.,1.12027918221652E-15));
#44669=DIRECTION('center_axis',(3.66113466765132E-16,1.,1.12027918221652E-15));
#44670=DIRECTION('ref_axis',(0.986988809780564,-1.81221371198957E-16,-0.160788959098396));
#44671=DIRECTION('center_axis',(-3.66113466765132E-16,-1.,-1.12027918221652E-15));
#44672=DIRECTION('ref_axis',(0.986988809780564,-1.81221371198957E-16,-0.160788959098396));
#44673=DIRECTION('',(-3.66113466765132E-16,-1.,-1.12027918221652E-15));
#44674=DIRECTION('center_axis',(3.66113466765132E-16,1.,1.12027918221652E-15));
#44675=DIRECTION('ref_axis',(-0.820363592147226,9.40969144345854E-16,-0.571842265558694));
#44676=DIRECTION('',(3.66113466765132E-16,1.,1.12027918221652E-15));
#44677=DIRECTION('center_axis',(-3.66113466765132E-16,-1.,-1.12027918221652E-15));
#44678=DIRECTION('ref_axis',(-0.820363592147226,9.40969144345854E-16,-0.571842265558694));
#44679=DIRECTION('center_axis',(3.66113466765132E-16,1.,1.12027918221652E-15));
#44680=DIRECTION('ref_axis',(0.179016861276627,1.03664171525558E-15,-0.983846005927078));
#44681=DIRECTION('',(3.66113466765132E-16,1.,1.12027918221652E-15));
#44682=DIRECTION('center_axis',(-3.66113466765132E-16,-1.,-1.12027918221652E-15));
#44683=DIRECTION('ref_axis',(0.179016861276627,1.03664171525558E-15,-0.983846005927078));
#44684=DIRECTION('',(3.66113466765132E-16,1.,1.12027918221652E-15));
#44685=DIRECTION('center_axis',(3.66113466765132E-16,1.,1.12027918221652E-15));
#44686=DIRECTION('ref_axis',(0.957557813108254,-2.76641069737229E-17,-0.288241278368206));
#44687=DIRECTION('center_axis',(-3.66113466765132E-16,-1.,-1.12027918221652E-15));
#44688=DIRECTION('ref_axis',(0.957557813108254,-2.76641069737229E-17,-0.288241278368206));
#44689=DIRECTION('',(-3.66113466765132E-16,-1.,-1.12027918221652E-15));
#44690=DIRECTION('center_axis',(3.66113466765132E-16,1.,1.12027918221652E-15));
#44691=DIRECTION('ref_axis',(-0.887985661366392,8.40287573324551E-16,-0.459871139785583));
#44692=DIRECTION('',(3.66113466765132E-16,1.,1.12027918221652E-15));
#44693=DIRECTION('center_axis',(-3.66113466765132E-16,-1.,-1.12027918221652E-15));
#44694=DIRECTION('ref_axis',(-0.887985661366392,8.40287573324551E-16,-0.459871139785583));
#44695=DIRECTION('center_axis',(3.66113466765132E-16,1.,1.12027918221652E-15));
#44696=DIRECTION('ref_axis',(0.0490676743274116,1.100965420525E-15,-0.998795456205173));
#44697=DIRECTION('',(3.66113466765132E-16,1.,1.12027918221652E-15));
#44698=DIRECTION('center_axis',(-3.66113466765132E-16,-1.,-1.12027918221652E-15));
#44699=DIRECTION('ref_axis',(0.0490676743274116,1.100965420525E-15,-0.998795456205173));
#44700=DIRECTION('',(3.66113466765132E-16,1.,1.12027918221652E-15));
#44701=DIRECTION('center_axis',(3.66113466765132E-16,1.,1.12027918221652E-15));
#44702=DIRECTION('ref_axis',(0.91174273676848,1.26366497791772E-16,-0.410761709449557));
#44703=DIRECTION('center_axis',(-3.66113466765132E-16,-1.,-1.12027918221652E-15));
#44704=DIRECTION('ref_axis',(0.91174273676848,1.26366497791772E-16,-0.410761709449557));
#44705=DIRECTION('',(-3.66113466765132E-16,-1.,-1.12027918221652E-15));
#44706=DIRECTION('center_axis',(3.66113466765132E-16,1.,1.12027918221652E-15));
#44707=DIRECTION('ref_axis',(-0.940414049723441,7.25228448951937E-16,-0.340031491310375));
#44708=DIRECTION('',(3.66113466765132E-16,1.,1.12027918221652E-15));
#44709=DIRECTION('center_axis',(-3.66113466765132E-16,-1.,-1.12027918221652E-15));
#44710=DIRECTION('ref_axis',(-0.940414049723441,7.25228448951937E-16,-0.340031491310375));
#44711=DIRECTION('center_axis',(3.66113466765132E-16,1.,1.12027918221652E-15));
#44712=DIRECTION('ref_axis',(-0.081721074133674,1.14645130220395E-15,-0.99665523930918));
#44713=DIRECTION('',(3.66113466765132E-16,1.,1.12027918221652E-15));
#44714=DIRECTION('center_axis',(-3.66113466765132E-16,-1.,-1.12027918221652E-15));
#44715=DIRECTION('ref_axis',(-0.081721074133674,1.14645130220395E-15,-0.99665523930918));
#44716=DIRECTION('',(3.66113466765132E-16,1.,1.12027918221652E-15));
#44717=DIRECTION('center_axis',(3.66113466765132E-16,1.,1.12027918221652E-15));
#44718=DIRECTION('ref_axis',(0.850327489419755,2.78234936744635E-16,-0.526253893797563));
#44719=DIRECTION('center_axis',(-3.66113466765132E-16,-1.,-1.12027918221652E-15));
#44720=DIRECTION('ref_axis',(0.850327489419755,2.78234936744635E-16,-0.526253893797563));
#44721=DIRECTION('',(-3.66113466765132E-16,-1.,-1.12027918221652E-15));
#44722=DIRECTION('center_axis',(3.66113466765132E-16,1.,1.12027918221652E-15));
#44723=DIRECTION('ref_axis',(-0.976751692957689,5.97760464746442E-16,-0.214373809744306));
#44724=DIRECTION('',(3.66113466765132E-16,1.,1.12027918221652E-15));
#44725=DIRECTION('center_axis',(-3.66113466765132E-16,-1.,-1.12027918221652E-15));
#44726=DIRECTION('ref_axis',(-0.976751692957689,5.97760464746442E-16,-0.214373809744306));
#44727=DIRECTION('center_axis',(3.66113466765132E-16,1.,1.12027918221652E-15));
#44728=DIRECTION('ref_axis',(-0.211111552358971,1.17232108424584E-15,-0.977461974943571));
#44729=DIRECTION('',(3.66113466765132E-16,1.,1.12027918221652E-15));
#44730=DIRECTION('center_axis',(-3.66113466765132E-16,-1.,-1.12027918221652E-15));
#44731=DIRECTION('ref_axis',(-0.211111552358971,1.17232108424584E-15,-0.977461974943571));
#44732=DIRECTION('',(3.66113466765132E-16,1.,1.12027918221652E-15));
#44733=DIRECTION('center_axis',(3.66113466765132E-16,1.,1.12027918221652E-15));
#44734=DIRECTION('ref_axis',(0.774362902971737,4.25342698788503E-16,-0.63274172811755));
#44735=DIRECTION('center_axis',(-3.66113466765132E-16,-1.,-1.12027918221652E-15));
#44736=DIRECTION('ref_axis',(0.774362902971737,4.25342698788503E-16,-0.63274172811755));
#44737=DIRECTION('',(-3.66113466765132E-16,-1.,-1.12027918221652E-15));
#44738=DIRECTION('center_axis',(3.66113466765132E-16,1.,1.12027918221652E-15));
#44739=DIRECTION('ref_axis',(-0.996376843918701,4.60064633258625E-16,-0.0850481328578625));
#44740=DIRECTION('',(3.66113466765132E-16,1.,1.12027918221652E-15));
#44741=DIRECTION('center_axis',(-3.66113466765132E-16,-1.,-1.12027918221652E-15));
#44742=DIRECTION('ref_axis',(-0.996376843918701,4.60064633258625E-16,-0.0850481328578625));
#44743=DIRECTION('center_axis',(3.66113466765132E-16,1.,1.12027918221652E-15));
#44744=DIRECTION('ref_axis',(-0.336889853392226,1.17813212750748E-15,-0.941544065183019));
#44745=DIRECTION('',(3.66113466765132E-16,1.,1.12027918221652E-15));
#44746=DIRECTION('center_axis',(-3.66113466765132E-16,-1.,-1.12027918221652E-15));
#44747=DIRECTION('ref_axis',(-0.336889853392226,1.17813212750748E-15,-0.941544065183019));
#44748=DIRECTION('',(3.66113466765132E-16,1.,1.12027918221652E-15));
#44749=DIRECTION('center_axis',(3.66113466765132E-16,1.,1.12027918221652E-15));
#44750=DIRECTION('ref_axis',(0.685148752559917,5.65172729328822E-16,-0.728403176040296));
#44751=DIRECTION('center_axis',(-3.66113466765132E-16,-1.,-1.12027918221652E-15));
#44752=DIRECTION('ref_axis',(0.685148752559917,5.65172729328822E-16,-0.728403176040296));
#44753=DIRECTION('',(-3.66113466765132E-16,-1.,-1.12027918221652E-15));
#44754=DIRECTION('center_axis',(3.66113466765132E-16,1.,1.12027918221652E-15));
#44755=DIRECTION('ref_axis',(-0.998953710832413,3.14496968341738E-16,0.045732741161576));
#44756=DIRECTION('',(3.66113466765132E-16,1.,1.12027918221652E-15));
#44757=DIRECTION('center_axis',(-3.66113466765132E-16,-1.,-1.12027918221652E-15));
#44758=DIRECTION('ref_axis',(-0.998953710832413,3.14496968341738E-16,0.045732741161576));
#44759=DIRECTION('center_axis',(3.66113466765132E-16,1.,1.12027918221652E-15));
#44760=DIRECTION('ref_axis',(-0.456903875630426,1.16378500342752E-15,-0.889516075421853));
#44761=DIRECTION('',(3.66113466765132E-16,1.,1.12027918221652E-15));
#44762=DIRECTION('center_axis',(-3.66113466765132E-16,-1.,-1.12027918221652E-15));
#44763=DIRECTION('ref_axis',(-0.456903875630426,1.16378500342752E-15,-0.889516075421853));
#44764=DIRECTION('',(3.66113466765132E-16,1.,1.12027918221652E-15));
#44765=DIRECTION('center_axis',(3.66113466765132E-16,1.,1.12027918221652E-15));
#44766=DIRECTION('ref_axis',(0.584211517032674,6.95332497774842E-16,-0.811601443669479));
#44767=DIRECTION('center_axis',(-3.66113466765132E-16,-1.,-1.12027918221652E-15));
#44768=DIRECTION('ref_axis',(0.584211517032674,6.95332497774842E-16,-0.811601443669479));
#44769=DIRECTION('',(-3.66113466765132E-16,-1.,-1.12027918221652E-15));
#44770=DIRECTION('center_axis',(3.66113466765132E-16,1.,1.12027918221652E-15));
#44771=DIRECTION('ref_axis',(-0.98443820279149,1.63548173101491E-16,0.175731115300228));
#44772=DIRECTION('',(3.66113466765132E-16,1.,1.12027918221652E-15));
#44773=DIRECTION('center_axis',(-3.66113466765132E-16,-1.,-1.12027918221652E-15));
#44774=DIRECTION('ref_axis',(-0.98443820279149,1.63548173101491E-16,0.175731115300228));
#44775=DIRECTION('center_axis',(3.66113466765132E-16,1.,1.12027918221652E-15));
#44776=DIRECTION('ref_axis',(-0.569100145878903,1.12952519527676E-15,-0.822268218989772));
#44777=DIRECTION('',(3.66113466765132E-16,1.,1.12027918221652E-15));
#44778=DIRECTION('center_axis',(-3.66113466765132E-16,-1.,-1.12027918221652E-15));
#44779=DIRECTION('ref_axis',(-0.569100145878903,1.12952519527676E-15,-0.822268218989772));
#44780=DIRECTION('',(3.66113466765132E-16,1.,1.12027918221652E-15));
#44781=DIRECTION('center_axis',(3.66113466765132E-16,1.,1.12027918221652E-15));
#44782=DIRECTION('ref_axis',(0.473278260474969,8.13594934401345E-16,-0.880912985579045));
#44783=DIRECTION('center_axis',(-3.66113466765132E-16,-1.,-1.12027918221652E-15));
#44784=DIRECTION('ref_axis',(0.473278260474969,8.13594934401345E-16,-0.880912985579045));
#44785=DIRECTION('',(-3.66113466765132E-16,-1.,-1.12027918221652E-15));
#44786=DIRECTION('center_axis',(3.66113466765132E-16,1.,1.12027918221652E-15));
#44787=DIRECTION('ref_axis',(-0.95307868416297,9.80102327535809E-18,0.302722681334224));
#44788=DIRECTION('',(3.66113466765132E-16,1.,1.12027918221652E-15));
#44789=DIRECTION('center_axis',(-3.66113466765132E-16,-1.,-1.12027918221652E-15));
#44790=DIRECTION('ref_axis',(-0.95307868416297,9.80102327535809E-18,0.302722681334224));
#44791=DIRECTION('center_axis',(3.66113466765132E-16,1.,1.12027918221652E-15));
#44792=DIRECTION('ref_axis',(-0.671558954847023,1.07593889787127E-15,-0.740951125354955));
#44793=DIRECTION('',(3.66113466765132E-16,1.,1.12027918221652E-15));
#44794=DIRECTION('center_axis',(-3.66113466765132E-16,-1.,-1.12027918221652E-15));
#44795=DIRECTION('ref_axis',(-0.671558954847023,1.07593889787127E-15,-0.740951125354955));
#44796=DIRECTION('',(3.66113466765132E-16,1.,1.12027918221652E-15));
#44797=DIRECTION('center_axis',(3.66113466765132E-16,1.,1.12027918221652E-15));
#44798=DIRECTION('ref_axis',(0.354247081663014,9.17936536129109E-16,-0.935151862070134));
#44799=DIRECTION('center_axis',(-3.66113466765132E-16,-1.,-1.12027918221652E-15));
#44800=DIRECTION('ref_axis',(0.354247081663014,9.17936536129109E-16,-0.935151862070134));
#44801=DIRECTION('',(-3.66113466765132E-16,-1.,-1.12027918221652E-15));
#44802=DIRECTION('center_axis',(3.66113466765132E-16,1.,1.12027918221652E-15));
#44803=DIRECTION('ref_axis',(-0.905411725005089,-1.44113824776374E-16,0.424534578360008));
#44804=DIRECTION('',(3.66113466765132E-16,1.,1.12027918221652E-15));
#44805=DIRECTION('center_axis',(-3.66113466765132E-16,-1.,-1.12027918221652E-15));
#44806=DIRECTION('ref_axis',(-0.905411725005089,-1.44113824776374E-16,0.424534578360008));
#44807=DIRECTION('center_axis',(3.66113466765132E-16,1.,1.12027918221652E-15));
#44808=DIRECTION('ref_axis',(-0.762527203906392,1.00394298761658E-15,-0.646956152534853));
#44809=DIRECTION('',(3.66113466765132E-16,1.,1.12027918221652E-15));
#44810=DIRECTION('center_axis',(-3.66113466765132E-16,-1.,-1.12027918221652E-15));
#44811=DIRECTION('ref_axis',(-0.762527203906392,1.00394298761658E-15,-0.646956152534853));
#44812=DIRECTION('',(3.66113466765132E-16,1.,1.12027918221652E-15));
#44813=DIRECTION('center_axis',(3.66113466765132E-16,1.,1.12027918221652E-15));
#44814=DIRECTION('ref_axis',(0.229154637067959,1.00657198922362E-15,-0.973390030928123));
#44815=DIRECTION('center_axis',(-3.66113466765132E-16,-1.,-1.12027918221652E-15));
#44816=DIRECTION('ref_axis',(0.229154637067959,1.00657198922362E-15,-0.973390030928123));
#44817=DIRECTION('',(-3.66113466765132E-16,-1.,-1.12027918221652E-15));
#44818=DIRECTION('center_axis',(3.66113466765132E-16,1.,1.12027918221652E-15));
#44819=DIRECTION('ref_axis',(-0.842252920204816,-2.9556284533028E-16,0.53908257104683));
#44820=DIRECTION('',(3.66113466765132E-16,1.,1.12027918221652E-15));
#44821=DIRECTION('center_axis',(-3.66113466765132E-16,-1.,-1.12027918221652E-15));
#44822=DIRECTION('ref_axis',(-0.842252920204816,-2.9556284533028E-16,0.53908257104683));
#44823=DIRECTION('center_axis',(3.66113466765132E-16,1.,1.12027918221652E-15));
#44824=DIRECTION('ref_axis',(-0.840448401094441,9.14769334498193E-16,-0.541891580574747));
#44825=DIRECTION('',(3.66113466765132E-16,1.,1.12027918221652E-15));
#44826=DIRECTION('center_axis',(-3.66113466765132E-16,-1.,-1.12027918221652E-15));
#44827=DIRECTION('ref_axis',(-0.840448401094441,9.14769334498193E-16,-0.541891580574747));
#44828=DIRECTION('',(3.66113466765132E-16,1.,1.12027918221652E-15));
#44829=DIRECTION('center_axis',(3.66113466765132E-16,1.,1.12027918221652E-15));
#44830=DIRECTION('ref_axis',(0.100141293099002,1.07798471650803E-15,-0.994973226482231));
#44831=DIRECTION('center_axis',(-3.66113466765132E-16,-1.,-1.12027918221652E-15));
#44832=DIRECTION('ref_axis',(0.100141293099002,1.07798471650803E-15,-0.994973226482231));
#44833=DIRECTION('',(-3.66113466765132E-16,-1.,-1.12027918221652E-15));
#44834=DIRECTION('center_axis',(3.66113466765132E-16,1.,1.12027918221652E-15));
#44835=DIRECTION('ref_axis',(-0.764682934423213,-4.41954703655085E-16,0.644406711481115));
#44836=DIRECTION('',(3.66113466765132E-16,1.,1.12027918221652E-15));
#44837=DIRECTION('center_axis',(-3.66113466765132E-16,-1.,-1.12027918221652E-15));
#44838=DIRECTION('ref_axis',(-0.764682934423213,-4.41954703655085E-16,0.644406711481115));
#44839=DIRECTION('center_axis',(3.66113466765132E-16,1.,1.12027918221652E-15));
#44840=DIRECTION('ref_axis',(-0.903989293123446,8.09943724444565E-16,-0.427555093430277));
#44841=DIRECTION('',(3.66113466765132E-16,1.,1.12027918221652E-15));
#44842=DIRECTION('center_axis',(-3.66113466765132E-16,-1.,-1.12027918221652E-15));
#44843=DIRECTION('ref_axis',(-0.903989293123446,8.09943724444565E-16,-0.427555093430277));
#44844=DIRECTION('',(3.66113466765132E-16,1.,1.12027918221652E-15));
#44845=DIRECTION('center_axis',(3.66113466765132E-16,1.,1.12027918221652E-15));
#44846=DIRECTION('ref_axis',(-0.0305854961592907,1.13095282641916E-15,-0.999532154272533));
#44847=DIRECTION('center_axis',(-3.66113466765132E-16,-1.,-1.12027918221652E-15));
#44848=DIRECTION('ref_axis',(-0.0305854961592907,1.13095282641916E-15,-0.999532154272533));
#44849=DIRECTION('',(-3.66113466765132E-16,-1.,-1.12027918221652E-15));
#44850=DIRECTION('center_axis',(3.66113466765132E-16,1.,1.12027918221652E-15));
#44851=DIRECTION('ref_axis',(-0.674029011623465,-5.80784594467357E-16,0.738704874418665));
#44852=DIRECTION('',(3.66113466765132E-16,1.,1.12027918221652E-15));
#44853=DIRECTION('center_axis',(-3.66113466765132E-16,-1.,-1.12027918221652E-15));
#44854=DIRECTION('ref_axis',(-0.674029011623465,-5.80784594467357E-16,0.738704874418665));
#44855=DIRECTION('center_axis',(3.66113466765132E-16,1.,1.12027918221652E-15));
#44856=DIRECTION('ref_axis',(-0.952062677713926,6.91259752706865E-16,-0.305903020096548));
#44857=DIRECTION('',(3.66113466765132E-16,1.,1.12027918221652E-15));
#44858=DIRECTION('center_axis',(-3.66113466765132E-16,-1.,-1.12027918221652E-15));
#44859=DIRECTION('ref_axis',(-0.952062677713926,6.91259752706865E-16,-0.305903020096548));
#44860=DIRECTION('',(3.66113466765132E-16,1.,1.12027918221652E-15));
#44861=DIRECTION('center_axis',(3.66113466765132E-16,1.,1.12027918221652E-15));
#44862=DIRECTION('ref_axis',(-0.160788959098396,1.1645700199109E-15,-0.986988809780564));
#44863=DIRECTION('center_axis',(-3.66113466765132E-16,-1.,-1.12027918221652E-15));
#44864=DIRECTION('ref_axis',(-0.160788959098396,1.1645700199109E-15,-0.986988809780564));
#44865=DIRECTION('',(-3.66113466765132E-16,-1.,-1.12027918221652E-15));
#44866=DIRECTION('center_axis',(3.66113466765132E-16,1.,1.12027918221652E-15));
#44867=DIRECTION('ref_axis',(-0.571842265558694,-7.09677099844381E-16,0.820363592147226));
#44868=DIRECTION('',(3.66113466765132E-16,1.,1.12027918221652E-15));
#44869=DIRECTION('center_axis',(-3.66113466765132E-16,-1.,-1.12027918221652E-15));
#44870=DIRECTION('ref_axis',(-0.571842265558694,-7.09677099844381E-16,0.820363592147226));
#44871=DIRECTION('center_axis',(3.66113466765132E-16,1.,1.12027918221652E-15));
#44872=DIRECTION('ref_axis',(-0.983846005927078,5.60748134946939E-16,-0.179016861276627));
#44873=DIRECTION('',(3.66113466765132E-16,1.,1.12027918221652E-15));
#44874=DIRECTION('center_axis',(-3.66113466765132E-16,-1.,-1.12027918221652E-15));
#44875=DIRECTION('ref_axis',(-0.983846005927078,5.60748134946939E-16,-0.179016861276627));
#44876=DIRECTION('',(3.66113466765132E-16,1.,1.12027918221652E-15));
#44877=DIRECTION('center_axis',(3.66113466765132E-16,1.,1.12027918221652E-15));
#44878=DIRECTION('ref_axis',(-0.288241278368206,1.17826109748215E-15,-0.957557813108254));
#44879=DIRECTION('center_axis',(-3.66113466765132E-16,-1.,-1.12027918221652E-15));
#44880=DIRECTION('ref_axis',(-0.288241278368206,1.17826109748215E-15,-0.957557813108254));
#44881=DIRECTION('',(-3.66113466765132E-16,-1.,-1.12027918221652E-15));
#44882=DIRECTION('center_axis',(3.66113466765132E-16,1.,1.12027918221652E-15));
#44883=DIRECTION('ref_axis',(-0.459871139785583,-8.26426833283405E-16,0.887985661366392));
#44884=DIRECTION('',(3.66113466765132E-16,1.,1.12027918221652E-15));
#44885=DIRECTION('center_axis',(-3.66113466765132E-16,-1.,-1.12027918221652E-15));
#44886=DIRECTION('ref_axis',(-0.459871139785583,-8.26426833283405E-16,0.887985661366392));
#44887=DIRECTION('center_axis',(3.66113466765132E-16,1.,1.12027918221652E-15));
#44888=DIRECTION('ref_axis',(-0.998795456205173,4.20641961129317E-16,-0.0490676743274121));
#44889=DIRECTION('',(3.66113466765132E-16,1.,1.12027918221652E-15));
#44890=DIRECTION('center_axis',(-3.66113466765132E-16,-1.,-1.12027918221652E-15));
#44891=DIRECTION('ref_axis',(-0.998795456205173,4.20641961129317E-16,-0.0490676743274121));
#44892=DIRECTION('',(3.66113466765132E-16,1.,1.12027918221652E-15));
#44893=DIRECTION('center_axis',(3.66113466765132E-16,1.,1.12027918221652E-15));
#44894=DIRECTION('ref_axis',(-0.410761709449556,1.17179180099979E-15,-0.91174273676848));
#44895=DIRECTION('center_axis',(-3.66113466765132E-16,-1.,-1.12027918221652E-15));
#44896=DIRECTION('ref_axis',(-0.410761709449556,1.17179180099979E-15,-0.91174273676848));
#44897=DIRECTION('',(-3.66113466765132E-16,-1.,-1.12027918221652E-15));
#44898=DIRECTION('center_axis',(3.66113466765132E-16,1.,1.12027918221652E-15));
#44899=DIRECTION('ref_axis',(-0.340031491310375,-9.29036174476144E-16,0.940414049723441));
#44900=DIRECTION('',(3.66113466765132E-16,1.,1.12027918221652E-15));
#44901=DIRECTION('center_axis',(-3.66113466765132E-16,-1.,-1.12027918221652E-15));
#44902=DIRECTION('ref_axis',(-0.340031491310375,-9.29036174476144E-16,0.940414049723441));
#44903=DIRECTION('center_axis',(3.66113466765132E-16,1.,1.12027918221652E-15));
#44904=DIRECTION('ref_axis',(5.46077161851015E-15,-1.12027918221652E-15,
1.));
#44905=DIRECTION('center_axis',(-3.66113466765132E-16,-1.,-1.12027918221652E-15));
#44906=DIRECTION('ref_axis',(5.46077161851015E-15,-1.12027918221652E-15,
1.));
#44907=DIRECTION('',(3.66113466765132E-16,1.,1.12027918221652E-15));
#44908=DIRECTION('center_axis',(3.66113466765132E-16,1.,1.12027918221652E-15));
#44909=DIRECTION('ref_axis',(5.46077161851015E-15,-1.12027918221652E-15,
1.));
#44910=DIRECTION('center_axis',(-3.66113466765132E-16,-1.,-1.12027918221652E-15));
#44911=DIRECTION('ref_axis',(5.46077161851015E-15,-1.12027918221652E-15,
1.));
#44912=DIRECTION('center_axis',(3.66113466765132E-16,1.,1.12027918221652E-15));
#44913=DIRECTION('ref_axis',(5.46077161851015E-15,-1.12027918221652E-15,
1.));
#44914=DIRECTION('center_axis',(-3.66113466765132E-16,-1.,-1.12027918221652E-15));
#44915=DIRECTION('ref_axis',(5.46077161851015E-15,-1.12027918221652E-15,
1.));
#44916=DIRECTION('center_axis',(3.66113466765132E-16,1.,1.12027918221652E-15));
#44917=DIRECTION('ref_axis',(5.46077161851015E-15,-1.12027918221652E-15,
1.));
#44918=DIRECTION('center_axis',(-3.66113466765132E-16,-1.,-1.12027918221652E-15));
#44919=DIRECTION('ref_axis',(5.46077161851015E-15,-1.12027918221652E-15,
1.));
#44920=DIRECTION('center_axis',(3.66113466765132E-16,1.,1.12027918221652E-15));
#44921=DIRECTION('ref_axis',(5.46077161851015E-15,-1.12027918221652E-15,
1.));
#44922=DIRECTION('center_axis',(-3.66113466765132E-16,-1.,-1.12027918221652E-15));
#44923=DIRECTION('ref_axis',(5.46077161851015E-15,-1.12027918221652E-15,
1.));
#44924=DIRECTION('center_axis',(3.66113466765132E-16,1.,1.12027918221652E-15));
#44925=DIRECTION('ref_axis',(5.46077161851015E-15,-1.12027918221652E-15,
1.));
#44926=DIRECTION('center_axis',(-3.66113466765132E-16,-1.,-1.12027918221652E-15));
#44927=DIRECTION('ref_axis',(5.46077161851015E-15,-1.12027918221652E-15,
1.));
#44928=DIRECTION('center_axis',(3.66113466765132E-16,1.,1.12027918221652E-15));
#44929=DIRECTION('ref_axis',(5.46077161851015E-15,-1.12027918221652E-15,
1.));
#44930=DIRECTION('center_axis',(-3.66113466765132E-16,-1.,-1.12027918221652E-15));
#44931=DIRECTION('ref_axis',(5.46077161851015E-15,-1.12027918221652E-15,
1.));
#44932=DIRECTION('center_axis',(3.66113466765132E-16,1.,1.12027918221652E-15));
#44933=DIRECTION('ref_axis',(5.46077161851015E-15,-1.12027918221652E-15,
1.));
#44934=DIRECTION('center_axis',(-3.66113466765132E-16,-1.,-1.12027918221652E-15));
#44935=DIRECTION('ref_axis',(5.46077161851015E-15,-1.12027918221652E-15,
1.));
#44936=DIRECTION('center_axis',(3.66113466765132E-16,1.,1.12027918221652E-15));
#44937=DIRECTION('ref_axis',(5.46077161851015E-15,-1.12027918221652E-15,
1.));
#44938=DIRECTION('center_axis',(-3.66113466765132E-16,-1.,-1.12027918221652E-15));
#44939=DIRECTION('ref_axis',(5.46077161851015E-15,-1.12027918221652E-15,
1.));
#44940=DIRECTION('center_axis',(3.66113466765132E-16,1.,1.12027918221652E-15));
#44941=DIRECTION('ref_axis',(5.46077161851015E-15,-1.12027918221652E-15,
1.));
#44942=DIRECTION('center_axis',(-3.66113466765132E-16,-1.,-1.12027918221652E-15));
#44943=DIRECTION('ref_axis',(5.46077161851015E-15,-1.12027918221652E-15,
1.));
#44944=DIRECTION('center_axis',(3.66113466765132E-16,1.,1.12027918221652E-15));
#44945=DIRECTION('ref_axis',(5.46077161851015E-15,-1.12027918221652E-15,
1.));
#44946=DIRECTION('center_axis',(-3.66113466765132E-16,-1.,-1.12027918221652E-15));
#44947=DIRECTION('ref_axis',(5.46077161851015E-15,-1.12027918221652E-15,
1.));
#44948=DIRECTION('center_axis',(3.66113466765132E-16,1.,1.12027918221652E-15));
#44949=DIRECTION('ref_axis',(5.46077161851015E-15,-1.12027918221652E-15,
1.));
#44950=DIRECTION('center_axis',(-3.66113466765132E-16,-1.,-1.12027918221652E-15));
#44951=DIRECTION('ref_axis',(5.46077161851015E-15,-1.12027918221652E-15,
1.));
#44952=DIRECTION('center_axis',(3.66113466765132E-16,1.,1.12027918221652E-15));
#44953=DIRECTION('ref_axis',(-5.78239614844548E-15,1.12027918221652E-15,
-1.));
#44954=DIRECTION('center_axis',(-3.66113466765132E-16,-1.,-1.12027918221652E-15));
#44955=DIRECTION('ref_axis',(5.46077161851015E-15,-1.12027918221652E-15,
1.));
#44956=DIRECTION('center_axis',(3.66113466765132E-16,1.,1.12027918221652E-15));
#44957=DIRECTION('ref_axis',(5.46077161851015E-15,-1.12027918221652E-15,
1.));
#44958=DIRECTION('center_axis',(-3.66113466765132E-16,-1.,-1.12027918221652E-15));
#44959=DIRECTION('ref_axis',(5.46077161851015E-15,-1.12027918221652E-15,
1.));
#44960=DIRECTION('center_axis',(3.66113466765132E-16,1.,1.12027918221652E-15));
#44961=DIRECTION('ref_axis',(5.46077161851015E-15,-1.12027918221652E-15,
1.));
#44962=DIRECTION('center_axis',(-3.66113466765132E-16,-1.,-1.12027918221652E-15));
#44963=DIRECTION('ref_axis',(5.46077161851015E-15,-1.12027918221652E-15,
1.));
#44964=DIRECTION('center_axis',(3.66113466765132E-16,1.,1.12027918221652E-15));
#44965=DIRECTION('ref_axis',(5.46077161851015E-15,-1.12027918221652E-15,
1.));
#44966=DIRECTION('center_axis',(-3.66113466765132E-16,-1.,-1.12027918221652E-15));
#44967=DIRECTION('ref_axis',(5.46077161851015E-15,-1.12027918221652E-15,
1.));
#44968=DIRECTION('center_axis',(3.66113466765132E-16,1.,1.12027918221652E-15));
#44969=DIRECTION('ref_axis',(5.46077161851015E-15,-1.12027918221652E-15,
1.));
#44970=DIRECTION('center_axis',(-3.66113466765132E-16,-1.,-1.12027918221652E-15));
#44971=DIRECTION('ref_axis',(5.46077161851015E-15,-1.12027918221652E-15,
1.));
#44972=DIRECTION('center_axis',(3.66113466765132E-16,1.,1.12027918221652E-15));
#44973=DIRECTION('ref_axis',(5.46077161851015E-15,-1.12027918221652E-15,
1.));
#44974=DIRECTION('center_axis',(-3.66113466765132E-16,-1.,-1.12027918221652E-15));
#44975=DIRECTION('ref_axis',(5.46077161851015E-15,-1.12027918221652E-15,
1.));
#44976=DIRECTION('center_axis',(3.66113466765132E-16,1.,1.12027918221652E-15));
#44977=DIRECTION('ref_axis',(5.46077161851015E-15,-1.12027918221652E-15,
1.));
#44978=DIRECTION('center_axis',(-3.66113466765132E-16,-1.,-1.12027918221652E-15));
#44979=DIRECTION('ref_axis',(5.46077161851015E-15,-1.12027918221652E-15,
1.));
#44980=DIRECTION('center_axis',(3.66113466765132E-16,1.,1.12027918221652E-15));
#44981=DIRECTION('ref_axis',(5.46077161851015E-15,-1.12027918221652E-15,
1.));
#44982=DIRECTION('center_axis',(-3.66113466765132E-16,-1.,-1.12027918221652E-15));
#44983=DIRECTION('ref_axis',(5.46077161851015E-15,-1.12027918221652E-15,
1.));
#44984=DIRECTION('center_axis',(3.66113466765132E-16,1.,1.12027918221652E-15));
#44985=DIRECTION('ref_axis',(5.46077161851015E-15,-1.12027918221652E-15,
1.));
#44986=DIRECTION('center_axis',(-3.66113466765132E-16,-1.,-1.12027918221652E-15));
#44987=DIRECTION('ref_axis',(5.46077161851015E-15,-1.12027918221652E-15,
1.));
#44988=DIRECTION('center_axis',(3.66113466765132E-16,1.,1.12027918221652E-15));
#44989=DIRECTION('ref_axis',(5.46077161851015E-15,-1.12027918221652E-15,
1.));
#44990=DIRECTION('center_axis',(-3.66113466765132E-16,-1.,-1.12027918221652E-15));
#44991=DIRECTION('ref_axis',(5.46077161851015E-15,-1.12027918221652E-15,
1.));
#44992=DIRECTION('center_axis',(3.66113466765132E-16,1.,1.12027918221652E-15));
#44993=DIRECTION('ref_axis',(5.46077161851015E-15,-1.12027918221652E-15,
1.));
#44994=DIRECTION('center_axis',(-3.66113466765132E-16,-1.,-1.12027918221652E-15));
#44995=DIRECTION('ref_axis',(5.46077161851015E-15,-1.12027918221652E-15,
1.));
#44996=DIRECTION('center_axis',(3.66113466765132E-16,1.,1.12027918221652E-15));
#44997=DIRECTION('ref_axis',(5.46077161851015E-15,-1.12027918221652E-15,
1.));
#44998=DIRECTION('center_axis',(-3.66113466765132E-16,-1.,-1.12027918221652E-15));
#44999=DIRECTION('ref_axis',(5.46077161851015E-15,-1.12027918221652E-15,
1.));
#45000=DIRECTION('center_axis',(3.66113466765132E-16,1.,1.12027918221652E-15));
#45001=DIRECTION('ref_axis',(5.46077161851015E-15,-1.12027918221652E-15,
1.));
#45002=DIRECTION('center_axis',(-3.66113466765132E-16,-1.,-1.12027918221652E-15));
#45003=DIRECTION('ref_axis',(5.46077161851015E-15,-1.12027918221652E-15,
1.));
#45004=DIRECTION('center_axis',(3.66113466765132E-16,1.,1.12027918221652E-15));
#45005=DIRECTION('ref_axis',(5.46077161851015E-15,-1.12027918221652E-15,
1.));
#45006=DIRECTION('center_axis',(-3.66113466765132E-16,-1.,-1.12027918221652E-15));
#45007=DIRECTION('ref_axis',(5.46077161851015E-15,-1.12027918221652E-15,
1.));
#45008=DIRECTION('center_axis',(3.66113466765132E-16,1.,1.12027918221652E-15));
#45009=DIRECTION('ref_axis',(5.46077161851015E-15,-1.12027918221652E-15,
1.));
#45010=DIRECTION('center_axis',(-3.66113466765132E-16,-1.,-1.12027918221652E-15));
#45011=DIRECTION('ref_axis',(5.46077161851015E-15,-1.12027918221652E-15,
1.));
#45012=DIRECTION('center_axis',(3.66113466765132E-16,1.,1.12027918221652E-15));
#45013=DIRECTION('ref_axis',(5.46077161851015E-15,-1.12027918221652E-15,
1.));
#45014=DIRECTION('center_axis',(-3.66113466765132E-16,-1.,-1.12027918221652E-15));
#45015=DIRECTION('ref_axis',(5.46077161851015E-15,-1.12027918221652E-15,
1.));
#45016=DIRECTION('center_axis',(3.66113466765132E-16,1.,1.12027918221652E-15));
#45017=DIRECTION('ref_axis',(5.46077161851015E-15,-1.12027918221652E-15,
1.));
#45018=DIRECTION('center_axis',(-3.66113466765132E-16,-1.,-1.12027918221652E-15));
#45019=DIRECTION('ref_axis',(5.46077161851015E-15,-1.12027918221652E-15,
1.));
#45020=DIRECTION('center_axis',(3.66113466765132E-16,1.,1.12027918221652E-15));
#45021=DIRECTION('ref_axis',(5.46077161851015E-15,-1.12027918221652E-15,
1.));
#45022=DIRECTION('center_axis',(-3.66113466765132E-16,-1.,-1.12027918221652E-15));
#45023=DIRECTION('ref_axis',(5.46077161851015E-15,-1.12027918221652E-15,
1.));
#45024=DIRECTION('center_axis',(3.66113466765132E-16,1.,1.12027918221652E-15));
#45025=DIRECTION('ref_axis',(5.46077161851015E-15,-1.12027918221652E-15,
1.));
#45026=DIRECTION('center_axis',(-3.66113466765132E-16,-1.,-1.12027918221652E-15));
#45027=DIRECTION('ref_axis',(5.46077161851015E-15,-1.12027918221652E-15,
1.));
#45028=DIRECTION('center_axis',(3.66113466765132E-16,1.,1.12027918221652E-15));
#45029=DIRECTION('ref_axis',(5.46077161851015E-15,-1.12027918221652E-15,
1.));
#45030=DIRECTION('center_axis',(-3.66113466765132E-16,-1.,-1.12027918221652E-15));
#45031=DIRECTION('ref_axis',(5.46077161851015E-15,-1.12027918221652E-15,
1.));
#45032=DIRECTION('center_axis',(3.66113466765132E-16,1.,1.12027918221652E-15));
#45033=DIRECTION('ref_axis',(5.46077161851015E-15,-1.12027918221652E-15,
1.));
#45034=DIRECTION('center_axis',(-3.66113466765132E-16,-1.,-1.12027918221652E-15));
#45035=DIRECTION('ref_axis',(5.46077161851015E-15,-1.12027918221652E-15,
1.));
#45036=DIRECTION('center_axis',(3.66113466765132E-16,1.,1.12027918221652E-15));
#45037=DIRECTION('ref_axis',(5.46077161851015E-15,-1.12027918221652E-15,
1.));
#45038=DIRECTION('center_axis',(-3.66113466765132E-16,-1.,-1.12027918221652E-15));
#45039=DIRECTION('ref_axis',(5.46077161851015E-15,-1.12027918221652E-15,
1.));
#45040=DIRECTION('center_axis',(3.66113466765132E-16,1.,1.12027918221652E-15));
#45041=DIRECTION('ref_axis',(5.46077161851015E-15,-1.12027918221652E-15,
1.));
#45042=DIRECTION('center_axis',(-3.66113466765132E-16,-1.,-1.12027918221652E-15));
#45043=DIRECTION('ref_axis',(5.46077161851015E-15,-1.12027918221652E-15,
1.));
#45044=DIRECTION('center_axis',(3.66113466765132E-16,1.,1.12027918221652E-15));
#45045=DIRECTION('ref_axis',(5.46077161851015E-15,-1.12027918221652E-15,
1.));
#45046=DIRECTION('center_axis',(-3.66113466765132E-16,-1.,-1.12027918221652E-15));
#45047=DIRECTION('ref_axis',(5.46077161851015E-15,-1.12027918221652E-15,
1.));
#45048=DIRECTION('center_axis',(3.66113466765132E-16,1.,1.12027918221652E-15));
#45049=DIRECTION('ref_axis',(5.46077161851015E-15,-1.12027918221652E-15,
1.));
#45050=DIRECTION('center_axis',(-3.66113466765132E-16,-1.,-1.12027918221652E-15));
#45051=DIRECTION('ref_axis',(5.46077161851015E-15,-1.12027918221652E-15,
1.));
#45052=DIRECTION('center_axis',(3.66113466765132E-16,1.,1.12027918221652E-15));
#45053=DIRECTION('ref_axis',(5.46077161851015E-15,-1.12027918221652E-15,
1.));
#45054=DIRECTION('center_axis',(-3.66113466765132E-16,-1.,-1.12027918221652E-15));
#45055=DIRECTION('ref_axis',(5.46077161851015E-15,-1.12027918221652E-15,
1.));
#45056=DIRECTION('center_axis',(3.66113466765132E-16,1.,1.12027918221652E-15));
#45057=DIRECTION('ref_axis',(5.46077161851015E-15,-1.12027918221652E-15,
1.));
#45058=DIRECTION('center_axis',(-3.66113466765132E-16,-1.,-1.12027918221652E-15));
#45059=DIRECTION('ref_axis',(5.46077161851015E-15,-1.12027918221652E-15,
1.));
#45060=DIRECTION('center_axis',(3.66113466765132E-16,1.,1.12027918221652E-15));
#45061=DIRECTION('ref_axis',(5.46077161851015E-15,-1.12027918221652E-15,
1.));
#45062=DIRECTION('center_axis',(-3.66113466765132E-16,-1.,-1.12027918221652E-15));
#45063=DIRECTION('ref_axis',(5.46077161851015E-15,-1.12027918221652E-15,
1.));
#45064=DIRECTION('center_axis',(3.66113466765132E-16,1.,1.12027918221652E-15));
#45065=DIRECTION('ref_axis',(5.46077161851015E-15,-1.12027918221652E-15,
1.));
#45066=DIRECTION('center_axis',(-3.66113466765132E-16,-1.,-1.12027918221652E-15));
#45067=DIRECTION('ref_axis',(5.46077161851015E-15,-1.12027918221652E-15,
1.));
#45068=DIRECTION('center_axis',(3.66113466765132E-16,1.,1.12027918221652E-15));
#45069=DIRECTION('ref_axis',(5.46077161851015E-15,-1.12027918221652E-15,
1.));
#45070=DIRECTION('center_axis',(-3.66113466765132E-16,-1.,-1.12027918221652E-15));
#45071=DIRECTION('ref_axis',(5.46077161851015E-15,-1.12027918221652E-15,
1.));
#45072=DIRECTION('center_axis',(3.66113466765132E-16,1.,1.12027918221652E-15));
#45073=DIRECTION('ref_axis',(5.46077161851015E-15,-1.12027918221652E-15,
1.));
#45074=DIRECTION('center_axis',(-3.66113466765132E-16,-1.,-1.12027918221652E-15));
#45075=DIRECTION('ref_axis',(5.46077161851015E-15,-1.12027918221652E-15,
1.));
#45076=DIRECTION('center_axis',(3.66113466765132E-16,1.,1.12027918221652E-15));
#45077=DIRECTION('ref_axis',(5.46077161851015E-15,-1.12027918221652E-15,
1.));
#45078=DIRECTION('center_axis',(-3.66113466765132E-16,-1.,-1.12027918221652E-15));
#45079=DIRECTION('ref_axis',(5.46077161851015E-15,-1.12027918221652E-15,
1.));
#45080=DIRECTION('center_axis',(3.66113466765132E-16,1.,1.12027918221652E-15));
#45081=DIRECTION('ref_axis',(5.46077161851015E-15,-1.12027918221652E-15,
1.));
#45082=DIRECTION('center_axis',(-3.66113466765132E-16,-1.,-1.12027918221652E-15));
#45083=DIRECTION('ref_axis',(5.46077161851015E-15,-1.12027918221652E-15,
1.));
#45084=DIRECTION('center_axis',(3.66113466765132E-16,1.,1.12027918221652E-15));
#45085=DIRECTION('ref_axis',(5.46077161851015E-15,-1.12027918221652E-15,
1.));
#45086=DIRECTION('center_axis',(-3.66113466765132E-16,-1.,-1.12027918221652E-15));
#45087=DIRECTION('ref_axis',(5.46077161851015E-15,-1.12027918221652E-15,
1.));
#45088=DIRECTION('center_axis',(3.66113466765132E-16,1.,1.12027918221652E-15));
#45089=DIRECTION('ref_axis',(5.46077161851015E-15,-1.12027918221652E-15,
1.));
#45090=DIRECTION('center_axis',(-3.66113466765132E-16,-1.,-1.12027918221652E-15));
#45091=DIRECTION('ref_axis',(5.46077161851015E-15,-1.12027918221652E-15,
1.));
#45092=DIRECTION('center_axis',(3.66113466765132E-16,1.,1.12027918221652E-15));
#45093=DIRECTION('ref_axis',(-0.99665523930918,2.73338486732788E-16,0.0817210741336742));
#45094=DIRECTION('',(3.66113466765132E-16,1.,1.12027918221652E-15));
#45095=DIRECTION('center_axis',(-3.66113466765132E-16,-1.,-1.12027918221652E-15));
#45096=DIRECTION('ref_axis',(-0.99665523930918,2.73338486732788E-16,0.0817210741336742));
#45097=DIRECTION('',(3.66113466765132E-16,1.,1.12027918221652E-15));
#45098=DIRECTION('center_axis',(3.66113466765132E-16,1.,1.12027918221652E-15));
#45099=DIRECTION('ref_axis',(-0.526253893797564,1.14527282192027E-15,-0.850327489419754));
#45100=DIRECTION('center_axis',(-3.66113466765132E-16,-1.,-1.12027918221652E-15));
#45101=DIRECTION('ref_axis',(-0.526253893797564,1.14527282192027E-15,-0.850327489419754));
#45102=DIRECTION('',(-3.66113466765132E-16,-1.,-1.12027918221652E-15));
#45103=DIRECTION('center_axis',(3.66113466765132E-16,1.,1.12027918221652E-15));
#45104=DIRECTION('ref_axis',(-0.214373809744306,-1.01574944914611E-15,0.976751692957689));
#45105=DIRECTION('center_axis',(-3.66113466765132E-16,-1.,-1.12027918221652E-15));
#45106=DIRECTION('ref_axis',(-0.214373809744306,-1.01574944914611E-15,0.976751692957689));
#45107=DIRECTION('center_axis',(3.66113466765132E-16,1.,1.12027918221652E-15));
#45108=DIRECTION('ref_axis',(5.46077161851015E-15,-1.12027918221652E-15,
1.));
#45109=DIRECTION('center_axis',(-3.66113466765132E-16,-1.,-1.12027918221652E-15));
#45110=DIRECTION('ref_axis',(5.46077161851015E-15,-1.12027918221652E-15,
1.));
#45111=DIRECTION('center_axis',(-3.66113466765132E-16,-1.,-1.12027918221652E-15));
#45112=DIRECTION('ref_axis',(5.46077161851015E-15,-1.12027918221652E-15,
1.));
#56404=CARTESIAN_POINT('',(0.,0.,0.));
#56405=CARTESIAN_POINT('Origin',(263.115917770968,8.52799273121002,445.000000551893));
#56406=CARTESIAN_POINT('',(263.115917770968,10.52799273121,473.000000551893));
#56407=CARTESIAN_POINT('Origin',(263.115917770968,10.52799273121,445.000000551893));
#56408=CARTESIAN_POINT('',(263.115917770968,8.52799273120999,475.000000551893));
#56409=CARTESIAN_POINT('Origin',(263.115917770968,8.52799273120999,473.000000551893));
#56410=CARTESIAN_POINT('',(263.115917770968,8.52799273121006,415.000000551893));
#56411=CARTESIAN_POINT('Origin',(263.115917770968,8.52799273121002,445.000000551893));
#56412=CARTESIAN_POINT('Origin',(263.115917770968,8.52799273121002,445.000000551893));
#56413=CARTESIAN_POINT('Origin',(263.115917770968,0.527992731210016,445.000000551893));
#56414=CARTESIAN_POINT('',(263.115917770968,2.52799273121005,415.000000551893));
#56415=CARTESIAN_POINT('',(263.115917770968,0.52799273121005,415.000000551893));
#56416=CARTESIAN_POINT('Origin',(263.115917770968,2.52799273121002,445.000000551893));
#56417=CARTESIAN_POINT('Origin',(263.115917770968,10.52799273121,445.000000551893));
#56418=CARTESIAN_POINT('',(276.863644855836,10.52799273121,439.000000551893));
#56419=CARTESIAN_POINT('',(282.115917770968,10.52799273121,439.000000551893));
#56420=CARTESIAN_POINT('',(272.615917770968,10.52799273121,439.000000551893));
#56421=CARTESIAN_POINT('',(282.115917770968,10.52799273121,451.000000551893));
#56422=CARTESIAN_POINT('',(282.115917770968,10.52799273121,448.000000551893));
#56423=CARTESIAN_POINT('',(276.863644855836,10.52799273121,451.000000551893));
#56424=CARTESIAN_POINT('',(269.989781313402,10.52799273121,451.000000551893));
#56425=CARTESIAN_POINT('Origin',(263.115917770968,10.52799273121,445.000000551893));
#56426=CARTESIAN_POINT('Origin',(263.115917770968,2.52799273121002,445.000000551893));
#56427=CARTESIAN_POINT('',(263.115917770968,0.527992731210052,413.000000551893));
#56428=CARTESIAN_POINT('Origin',(263.115917770968,0.527992731210016,445.000000551893));
#56429=CARTESIAN_POINT('Origin',(263.115917770968,2.52799273121005,413.000000551893));
#56430=CARTESIAN_POINT('Origin',(263.115917770968,0.527992731210016,445.000000551893));
#56431=CARTESIAN_POINT('',(199.31403287824,0.52799273121003,454.464116154264));
#56432=CARTESIAN_POINT('',(205.064770108999,0.527992731210025,455.562765644546));
#56433=CARTESIAN_POINT('Origin',(207.471787643001,0.527992731210056,427.363480684421));
#56434=CARTESIAN_POINT('',(205.441455406363,0.527992731210025,457.456490516082));
#56435=CARTESIAN_POINT('Origin',(263.115917770968,0.527992731210016,445.000000551893));
#56436=CARTESIAN_POINT('',(200.54890193992,0.527992731210021,460.672222155654));
#56437=CARTESIAN_POINT('Origin',(218.456648799204,0.52799273120999,482.58810699052));
#56438=CARTESIAN_POINT('',(201.095181820417,0.527992731210021,462.710966424822));
#56439=CARTESIAN_POINT('Origin',(263.115917770968,0.527992731210016,445.000000551893));
#56440=CARTESIAN_POINT('',(206.940123231516,0.527992731210016,463.049594983223));
#56441=CARTESIAN_POINT('Origin',(205.645803107665,0.527992731210047,434.777379981771));
#56442=CARTESIAN_POINT('',(207.560766630536,0.527992731210014,464.877951478433));
#56443=CARTESIAN_POINT('Origin',(263.115917770968,0.527992731210016,445.000000551893));
#56444=CARTESIAN_POINT('',(203.129806843349,0.527992731210012,468.704778462252));
#56445=CARTESIAN_POINT('Origin',(223.744947442398,0.527992731209983,488.095739855457));
#56446=CARTESIAN_POINT('',(203.937522750105,0.52799273121001,470.654777158886));
#56447=CARTESIAN_POINT('Origin',(263.115917770968,0.527992731210016,445.000000551893));
#56448=CARTESIAN_POINT('',(209.776659773475,0.527992731210007,470.227590756887));
#56449=CARTESIAN_POINT('Origin',(204.803148167944,0.527992731210039,442.366191151322));
#56450=CARTESIAN_POINT('',(210.630641893519,0.527992731210005,471.959295189222));
#56451=CARTESIAN_POINT('Origin',(263.115917770968,0.527992731210016,445.000000551893));
#56452=CARTESIAN_POINT('',(206.737090736042,0.527992731210001,476.331739446597));
#56453=CARTESIAN_POINT('Origin',(229.706894303609,0.527992731209974,492.865992672514));
#56454=CARTESIAN_POINT('',(207.792422425951,0.527992731209999,478.159627552356));
#56455=CARTESIAN_POINT('Origin',(263.115917770968,0.527992731210016,445.000000551893));
#56456=CARTESIAN_POINT('',(213.525845808207,0.527992731209999,476.973935467734));
#56457=CARTESIAN_POINT('Origin',(204.958240883485,0.527992731210034,450.000067529947));
#56458=CARTESIAN_POINT('',(214.598554778434,0.527992731209996,478.579357894238));
#56459=CARTESIAN_POINT('Origin',(263.115917770968,0.527992731210016,445.000000551893));
#56460=CARTESIAN_POINT('',(211.309031990467,0.527992731209992,483.422605691655));
#56461=CARTESIAN_POINT('Origin',(236.240478819077,0.527992731209967,496.817245093427));
#56462=CARTESIAN_POINT('',(212.59392244572,0.52799273120999,485.097107534263));
#56463=CARTESIAN_POINT('Origin',(263.115917770968,0.527992731210016,445.000000551893));
#56464=CARTESIAN_POINT('',(218.123531723188,0.52799273120999,483.173197287322));
#56465=CARTESIAN_POINT('Origin',(206.108427574925,0.527992731210025,457.548391376297));
#56466=CARTESIAN_POINT('',(219.396613195705,0.527992731209987,484.62486848517));
#56467=CARTESIAN_POINT('Origin',(263.115917770968,0.527992731210016,445.000000551893));
#56468=CARTESIAN_POINT('',(216.767403424178,0.527992731209983,489.856050510013));
#56469=CARTESIAN_POINT('Origin',(243.233909546292,0.527992731209963,499.881890093779));
#56470=CARTESIAN_POINT('',(218.259867812848,0.527992731209981,491.348514898684));
#56471=CARTESIAN_POINT('Origin',(263.115917770968,0.527992731210016,445.000000551893));
#56472=CARTESIAN_POINT('',(223.491049837692,0.527992731209981,488.719305127157));
#56473=CARTESIAN_POINT('Origin',(208.234028229082,0.527992731210014,464.88200877657));
#56474=CARTESIAN_POINT('',(224.94272103554,0.527992731209981,489.992386599674));
#56475=CARTESIAN_POINT('Origin',(263.115917770968,0.527992731210016,445.000000551893));
#56476=CARTESIAN_POINT('',(223.018810788598,0.527992731209974,495.521995877141));
#56477=CARTESIAN_POINT('Origin',(250.567526946565,0.527992731209956,502.007490747936));
#56478=CARTESIAN_POINT('',(224.693312631207,0.527992731209972,496.806886332395));
#56479=CARTESIAN_POINT('Origin',(263.115917770968,0.527992731210016,445.000000551893));
#56480=CARTESIAN_POINT('',(229.536560428624,0.527992731209974,493.517363544428));
#56481=CARTESIAN_POINT('Origin',(211.298673229435,0.527992731210005,471.875439503784));
#56482=CARTESIAN_POINT('',(231.141982855127,0.527992731209972,494.590072514654));
#56483=CARTESIAN_POINT('Origin',(263.115917770968,0.527992731210016,445.000000551893));
#56484=CARTESIAN_POINT('',(229.956290770506,0.527992731209967,500.323495896911));
#56485=CARTESIAN_POINT('Origin',(258.115850792915,0.527992731209952,503.157677439376));
#56486=CARTESIAN_POINT('',(231.784178876265,0.527992731209965,501.378827586819));
#56487=CARTESIAN_POINT('Origin',(263.115917770968,0.527992731210016,445.000000551893));
#56488=CARTESIAN_POINT('',(236.15662313364,0.527992731209967,497.485276429342));
#56489=CARTESIAN_POINT('Origin',(215.249925650348,0.527992731209996,478.409024019253));
#56490=CARTESIAN_POINT('',(237.888327565975,0.527992731209965,498.339258549387));
#56491=CARTESIAN_POINT('Origin',(263.115917770968,0.527992731210016,445.000000551893));
#56492=CARTESIAN_POINT('',(237.461141163976,0.527992731209959,504.178395572756));
#56493=CARTESIAN_POINT('Origin',(265.74972717154,0.52799273120995,503.312770154917));
#56494=CARTESIAN_POINT('',(239.41113986061,0.527992731209959,504.986111479512));
#56495=CARTESIAN_POINT('Origin',(263.115917770968,0.527992731210016,445.000000551893));
#56496=CARTESIAN_POINT('',(243.237966844429,0.527992731209961,500.555151692326));
#56497=CARTESIAN_POINT('Origin',(220.020178467405,0.527992731209987,484.370970880464));
#56498=CARTESIAN_POINT('',(245.066323339639,0.527992731209961,501.175795091346));
#56499=CARTESIAN_POINT('Origin',(263.115917770968,0.527992731210016,445.000000551893));
#56500=CARTESIAN_POINT('',(245.40495189804,0.527992731209954,507.020736502444));
#56501=CARTESIAN_POINT('Origin',(273.338538341091,0.527992731209947,502.470115215196));
#56502=CARTESIAN_POINT('',(247.443696167208,0.527992731209952,507.567016382941));
#56503=CARTESIAN_POINT('Origin',(263.115917770968,0.527992731210016,445.000000551893));
#56504=CARTESIAN_POINT('',(250.65942780678,0.527992731209956,502.674462916499));
#56505=CARTESIAN_POINT('Origin',(225.527811332342,0.527992731209981,489.659269523657));
#56506=CARTESIAN_POINT('',(252.553152678316,0.527992731209954,503.051148213862));
#56507=CARTESIAN_POINT('Origin',(263.115917770968,0.527992731210016,445.000000551893));
#56508=CARTESIAN_POINT('',(253.651802168598,0.527992731209947,508.801885444622));
#56509=CARTESIAN_POINT('Origin',(280.752437638441,0.527992731209947,500.64413067986));
#56510=CARTESIAN_POINT('',(255.744408530607,0.527992731209947,509.077382298647));
#56511=CARTESIAN_POINT('Origin',(263.115917770968,0.527992731210016,445.000000551893));
#56512=CARTESIAN_POINT('',(258.29402276601,0.527992731209952,503.806948099231));
#56513=CARTESIAN_POINT('Origin',(231.678587119835,0.527992731209972,494.183435692855));
#56514=CARTESIAN_POINT('',(260.22071385628,0.527992731209952,503.933230105063));
#56515=CARTESIAN_POINT('Origin',(263.115917770968,0.527992731210016,445.000000551893));
#56516=CARTESIAN_POINT('',(262.06058608106,0.527992731209945,509.49136644706));
#56517=CARTESIAN_POINT('Origin',(287.864571191092,0.527992731209947,497.866059650567));
#56518=CARTESIAN_POINT('',(264.171249460877,0.527992731209943,509.49136644706));
#56519=CARTESIAN_POINT('Origin',(263.115917770968,0.527992731210016,445.000000551893));
#56520=CARTESIAN_POINT('',(266.011121685657,0.52799273120995,503.933230105063));
#56521=CARTESIAN_POINT('Origin',(238.367264350845,0.527992731209965,497.866059650567));
#56522=CARTESIAN_POINT('',(267.937812775927,0.52799273120995,503.806948099231));
#56523=CARTESIAN_POINT('Origin',(263.115917770968,0.527992731210016,445.000000551893));
#56524=CARTESIAN_POINT('',(270.48742701133,0.527992731209941,509.077382298647));
#56525=CARTESIAN_POINT('Origin',(294.553248422101,0.52799273120995,494.183435692855));
#56526=CARTESIAN_POINT('',(272.580033373339,0.527992731209941,508.801885444621));
#56527=CARTESIAN_POINT('Origin',(263.115917770968,0.527992731210016,445.000000551893));
#56528=CARTESIAN_POINT('',(273.678682863621,0.527992731209947,503.051148213862));
#56529=CARTESIAN_POINT('Origin',(245.479397903496,0.527992731209961,500.64413067986));
#56530=CARTESIAN_POINT('',(275.572407735157,0.527992731209947,502.674462916499));
#56531=CARTESIAN_POINT('Origin',(263.115917770968,0.527992731210016,445.000000551893));
#56532=CARTESIAN_POINT('',(278.788139374729,0.527992731209941,507.567016382941));
#56533=CARTESIAN_POINT('Origin',(300.704024209595,0.527992731209952,489.659269523657));
#56534=CARTESIAN_POINT('',(280.826883643897,0.527992731209941,507.020736502444));
#56535=CARTESIAN_POINT('Origin',(263.115917770968,0.527992731210016,445.000000551893));
#56536=CARTESIAN_POINT('',(281.165512202298,0.527992731209947,501.175795091345));
#56537=CARTESIAN_POINT('Origin',(252.893297200846,0.527992731209956,502.470115215196));
#56538=CARTESIAN_POINT('',(282.993868697508,0.527992731209947,500.555151692326));
#56539=CARTESIAN_POINT('Origin',(263.115917770968,0.527992731210016,445.000000551893));
#56540=CARTESIAN_POINT('',(286.820695681327,0.527992731209941,504.986111479512));
#56541=CARTESIAN_POINT('Origin',(306.211657074532,0.527992731209956,484.370970880463));
#56542=CARTESIAN_POINT('',(288.770694377961,0.527992731209941,504.178395572756));
#56543=CARTESIAN_POINT('Origin',(263.115917770968,0.527992731210016,445.000000551893));
#56544=CARTESIAN_POINT('',(288.343507975962,0.527992731209947,498.339258549386));
#56545=CARTESIAN_POINT('Origin',(260.482108370397,0.527992731209952,503.312770154917));
#56546=CARTESIAN_POINT('',(290.075212408297,0.527992731209947,497.485276429342));
#56547=CARTESIAN_POINT('Origin',(263.115917770968,0.527992731210016,445.000000551893));
#56548=CARTESIAN_POINT('',(294.447656665672,0.527992731209941,501.378827586819));
#56549=CARTESIAN_POINT('Origin',(310.981909891589,0.527992731209961,478.409024019252));
#56550=CARTESIAN_POINT('',(296.275544771431,0.527992731209943,500.32349589691));
#56551=CARTESIAN_POINT('Origin',(263.115917770968,0.527992731210016,445.000000551893));
#56552=CARTESIAN_POINT('',(295.089852686809,0.52799273120995,494.590072514654));
#56553=CARTESIAN_POINT('Origin',(268.115984749022,0.52799273120995,503.157677439376));
#56554=CARTESIAN_POINT('',(296.695275113313,0.52799273120995,493.517363544428));
#56555=CARTESIAN_POINT('Origin',(263.115917770968,0.527992731210016,445.000000551893));
#56556=CARTESIAN_POINT('',(301.53852291073,0.527992731209945,496.806886332394));
#56557=CARTESIAN_POINT('Origin',(314.933162312502,0.527992731209967,471.875439503784));
#56558=CARTESIAN_POINT('',(303.213024753338,0.527992731209945,495.521995877141));
#56559=CARTESIAN_POINT('Origin',(263.115917770968,0.527992731210016,445.000000551893));
#56560=CARTESIAN_POINT('',(301.289114506397,0.527992731209952,489.992386599673));
#56561=CARTESIAN_POINT('Origin',(275.664308595372,0.527992731209947,502.007490747936));
#56562=CARTESIAN_POINT('',(302.740785704245,0.527992731209952,488.719305127157));
#56563=CARTESIAN_POINT('Origin',(263.115917770968,0.527992731210016,445.000000551893));
#56564=CARTESIAN_POINT('',(307.971967729088,0.527992731209947,491.348514898683));
#56565=CARTESIAN_POINT('Origin',(317.997807312854,0.527992731209974,464.882008776569));
#56566=CARTESIAN_POINT('',(309.464432117759,0.52799273120995,489.856050510013));
#56567=CARTESIAN_POINT('Origin',(263.115917770968,0.527992731210016,445.000000551893));
#56568=CARTESIAN_POINT('',(306.835222346232,0.527992731209956,484.624868485169));
#56569=CARTESIAN_POINT('Origin',(282.997925995645,0.527992731209947,499.881890093779));
#56570=CARTESIAN_POINT('',(308.108303818749,0.527992731209956,483.173197287322));
#56571=CARTESIAN_POINT('Origin',(263.115917770968,0.527992731210016,445.000000551893));
#56572=CARTESIAN_POINT('',(313.637913096216,0.527992731209952,485.097107534263));
#56573=CARTESIAN_POINT('Origin',(320.123407967011,0.527992731209981,457.548391376296));
#56574=CARTESIAN_POINT('',(314.92280355147,0.527992731209954,483.422605691655));
#56575=CARTESIAN_POINT('Origin',(263.115917770968,0.527992731210016,445.000000551893));
#56576=CARTESIAN_POINT('',(311.633280763503,0.527992731209961,478.579357894237));
#56577=CARTESIAN_POINT('Origin',(289.99135672286,0.527992731209947,496.817245093426));
#56578=CARTESIAN_POINT('',(312.705989733729,0.527992731209963,476.973935467734));
#56579=CARTESIAN_POINT('Origin',(263.115917770968,0.527992731210016,445.000000551893));
#56580=CARTESIAN_POINT('',(318.439413115986,0.527992731209959,478.159627552356));
#56581=CARTESIAN_POINT('Origin',(321.273594658451,0.52799273120999,450.000067529946));
#56582=CARTESIAN_POINT('',(319.494744805894,0.527992731209961,476.331739446597));
#56583=CARTESIAN_POINT('Origin',(263.115917770968,0.527992731210016,445.000000551893));
#56584=CARTESIAN_POINT('',(315.601193648417,0.527992731209967,471.959295189222));
#56585=CARTESIAN_POINT('Origin',(296.524941238328,0.52799273120995,492.865992672513));
#56586=CARTESIAN_POINT('',(316.455175768462,0.527992731209967,470.227590756886));
#56587=CARTESIAN_POINT('Origin',(263.115917770968,0.527992731210016,445.000000551893));
#56588=CARTESIAN_POINT('',(322.294312791831,0.527992731209965,470.654777158885));
#56589=CARTESIAN_POINT('Origin',(321.428687373992,0.527992731209999,442.366191151322));
#56590=CARTESIAN_POINT('',(323.102028698587,0.527992731209967,468.704778462251));
#56591=CARTESIAN_POINT('Origin',(263.115917770968,0.527992731210016,445.000000551893));
#56592=CARTESIAN_POINT('',(318.671068911401,0.527992731209974,464.877951478433));
#56593=CARTESIAN_POINT('Origin',(302.486888099539,0.527992731209954,488.095739855457));
#56594=CARTESIAN_POINT('',(319.291712310421,0.527992731209976,463.049594983222));
#56595=CARTESIAN_POINT('Origin',(263.115917770968,0.527992731210016,445.000000551893));
#56596=CARTESIAN_POINT('',(325.136653721519,0.527992731209974,462.710966424821));
#56597=CARTESIAN_POINT('Origin',(320.586032434271,0.527992731210007,434.77737998177));
#56598=CARTESIAN_POINT('',(325.682933602016,0.527992731209976,460.672222155653));
#56599=CARTESIAN_POINT('Origin',(263.115917770968,0.527992731210016,445.000000551893));
#56600=CARTESIAN_POINT('',(320.790380135574,0.527992731209981,457.456490516081));
#56601=CARTESIAN_POINT('Origin',(307.775186742732,0.527992731209959,482.588106990519));
#56602=CARTESIAN_POINT('',(321.167065432937,0.527992731209983,455.562765644545));
#56603=CARTESIAN_POINT('Origin',(263.115917770968,0.527992731210016,445.000000551893));
#56604=CARTESIAN_POINT('',(326.917802663697,0.527992731209983,454.464116154263));
#56605=CARTESIAN_POINT('Origin',(318.760047898935,0.527992731210016,427.36348068442));
#56606=CARTESIAN_POINT('',(327.193299517722,0.527992731209985,452.371509792254));
#56607=CARTESIAN_POINT('Origin',(263.115917770968,0.527992731210016,445.000000551893));
#56608=CARTESIAN_POINT('',(321.922865318307,0.52799273120999,449.821895556851));
#56609=CARTESIAN_POINT('Origin',(312.29935291193,0.527992731209963,476.437331203026));
#56610=CARTESIAN_POINT('',(322.049147324138,0.527992731209992,447.895204466581));
#56611=CARTESIAN_POINT('Origin',(263.115917770968,0.527992731210016,445.000000551893));
#56612=CARTESIAN_POINT('',(327.607283666135,0.527992731209992,446.055332241801));
#56613=CARTESIAN_POINT('Origin',(315.981976869642,0.527992731210025,420.251347131769));
#56614=CARTESIAN_POINT('',(327.607283666135,0.527992731209994,443.944668861984));
#56615=CARTESIAN_POINT('Origin',(263.115917770968,0.527992731210016,445.000000551893));
#56616=CARTESIAN_POINT('',(322.049147324138,0.527992731209999,442.104796637205));
#56617=CARTESIAN_POINT('Origin',(315.981976869642,0.52799273120997,469.748653972016));
#56618=CARTESIAN_POINT('',(321.922865318307,0.527992731210001,440.178105546934));
#56619=CARTESIAN_POINT('Origin',(263.115917770968,0.527992731210016,445.000000551893));
#56620=CARTESIAN_POINT('',(327.193299517722,0.527992731210001,437.628491311531));
#56621=CARTESIAN_POINT('Origin',(312.29935291193,0.527992731210034,413.56266990076));
#56622=CARTESIAN_POINT('',(326.917802663696,0.527992731210003,435.535884949522));
#56623=CARTESIAN_POINT('Origin',(263.115917770968,0.527992731210016,445.000000551893));
#56624=CARTESIAN_POINT('',(321.167065432937,0.527992731210007,434.43723545924));
#56625=CARTESIAN_POINT('Origin',(318.760047898935,0.527992731209976,462.636520419365));
#56626=CARTESIAN_POINT('',(320.790380135574,0.52799273121001,432.543510587704));
#56627=CARTESIAN_POINT('Origin',(263.115917770968,0.527992731210016,445.000000551893));
#56628=CARTESIAN_POINT('',(325.682933602016,0.527992731210012,429.327778948132));
#56629=CARTESIAN_POINT('Origin',(307.775186742732,0.527992731210043,407.411894113266));
#56630=CARTESIAN_POINT('',(325.136653721519,0.527992731210014,427.289034678965));
#56631=CARTESIAN_POINT('Origin',(263.115917770968,0.527992731210016,445.000000551893));
#56632=CARTESIAN_POINT('',(319.29171231042,0.527992731210016,426.950406120563));
#56633=CARTESIAN_POINT('Origin',(320.586032434271,0.527992731209983,455.222621122015));
#56634=CARTESIAN_POINT('',(318.671068911401,0.527992731210016,425.122049625353));
#56635=CARTESIAN_POINT('Origin',(263.115917770968,0.527992731210016,445.000000551893));
#56636=CARTESIAN_POINT('',(323.102028698587,0.527992731210021,421.295222641534));
#56637=CARTESIAN_POINT('Origin',(302.486888099538,0.527992731210052,401.904261248329));
#56638=CARTESIAN_POINT('',(322.294312791831,0.527992731210025,419.345223944901));
#56639=CARTESIAN_POINT('Origin',(263.115917770968,0.527992731210016,445.000000551893));
#56640=CARTESIAN_POINT('',(316.455175768461,0.527992731210025,419.772410346899));
#56641=CARTESIAN_POINT('Origin',(321.428687373992,0.527992731209992,447.633809952464));
#56642=CARTESIAN_POINT('',(315.601193648417,0.527992731210025,418.040705914564));
#56643=CARTESIAN_POINT('Origin',(263.115917770968,0.527992731210016,445.000000551893));
#56644=CARTESIAN_POINT('',(319.494744805894,0.52799273121003,413.668261657189));
#56645=CARTESIAN_POINT('Origin',(296.524941238327,0.527992731210056,397.134008431272));
#56646=CARTESIAN_POINT('',(318.439413115985,0.527992731210034,411.84037355143));
#56647=CARTESIAN_POINT('Origin',(263.115917770968,0.527992731210016,445.000000551893));
#56648=CARTESIAN_POINT('',(312.705989733729,0.527992731210034,413.026065636052));
#56649=CARTESIAN_POINT('Origin',(321.273594658451,0.527992731210001,439.999933573839));
#56650=CARTESIAN_POINT('',(311.633280763503,0.527992731210034,411.420643209548));
#56651=CARTESIAN_POINT('Origin',(263.115917770968,0.527992731210016,445.000000551893));
#56652=CARTESIAN_POINT('',(314.92280355147,0.527992731210039,406.577395412131));
#56653=CARTESIAN_POINT('Origin',(289.991356722859,0.527992731210065,393.18275601036));
#56654=CARTESIAN_POINT('',(313.637913096216,0.527992731210043,404.902893569523));
#56655=CARTESIAN_POINT('Origin',(263.115917770968,0.527992731210016,445.000000551893));
#56656=CARTESIAN_POINT('',(308.108303818748,0.527992731210043,406.826803816464));
#56657=CARTESIAN_POINT('Origin',(320.123407967011,0.52799273121001,432.451609727489));
#56658=CARTESIAN_POINT('',(306.835222346232,0.527992731210043,405.375132618617));
#56659=CARTESIAN_POINT('Origin',(263.115917770968,0.527992731210016,445.000000551893));
#56660=CARTESIAN_POINT('',(309.464432117758,0.527992731210047,400.143950593773));
#56661=CARTESIAN_POINT('Origin',(282.997925995644,0.52799273121007,390.118111010007));
#56662=CARTESIAN_POINT('',(307.971967729088,0.527992731210052,398.651486205102));
#56663=CARTESIAN_POINT('Origin',(263.115917770968,0.527992731210016,445.000000551893));
#56664=CARTESIAN_POINT('',(302.740785704244,0.527992731210052,401.280695976629));
#56665=CARTESIAN_POINT('Origin',(317.997807312854,0.527992731210016,425.117992327216));
#56666=CARTESIAN_POINT('',(301.289114506397,0.527992731210052,400.007614504112));
#56667=CARTESIAN_POINT('Origin',(263.115917770968,0.527992731210016,445.000000551893));
#56668=CARTESIAN_POINT('',(303.213024753338,0.527992731210056,394.478005226645));
#56669=CARTESIAN_POINT('Origin',(275.664308595371,0.527992731210074,387.99251035585));
#56670=CARTESIAN_POINT('',(301.53852291073,0.527992731210061,393.193114771391));
#56671=CARTESIAN_POINT('Origin',(263.115917770968,0.527992731210016,445.000000551893));
#56672=CARTESIAN_POINT('',(296.695275113313,0.527992731210056,396.482637559358));
#56673=CARTESIAN_POINT('Origin',(314.933162312501,0.52799273121003,418.124561600002));
#56674=CARTESIAN_POINT('',(295.089852686809,0.527992731210061,395.409928589132));
#56675=CARTESIAN_POINT('Origin',(263.115917770968,0.527992731210016,445.000000551893));
#56676=CARTESIAN_POINT('',(296.275544771431,0.527992731210065,389.676505206875));
#56677=CARTESIAN_POINT('Origin',(268.115984749021,0.527992731210079,386.84232366441));
#56678=CARTESIAN_POINT('',(294.447656665672,0.52799273121007,388.621173516967));
#56679=CARTESIAN_POINT('Origin',(263.115917770968,0.527992731210016,445.000000551893));
#56680=CARTESIAN_POINT('',(290.075212408297,0.527992731210065,392.514724674444));
#56681=CARTESIAN_POINT('Origin',(310.981909891589,0.527992731210034,411.590977084533));
#56682=CARTESIAN_POINT('',(288.343507975962,0.527992731210065,391.6607425544));
#56683=CARTESIAN_POINT('Origin',(263.115917770968,0.527992731210016,445.000000551893));
#56684=CARTESIAN_POINT('',(288.77069437796,0.527992731210074,385.82160553103));
#56685=CARTESIAN_POINT('Origin',(260.482108370397,0.527992731210083,386.687230948869));
#56686=CARTESIAN_POINT('',(286.820695681326,0.527992731210074,385.013889624274));
#56687=CARTESIAN_POINT('Origin',(263.115917770968,0.527992731210016,445.000000551893));
#56688=CARTESIAN_POINT('',(282.993868697508,0.52799273121007,389.44484941146));
#56689=CARTESIAN_POINT('Origin',(306.211657074532,0.527992731210043,405.629030223323));
#56690=CARTESIAN_POINT('',(281.165512202297,0.527992731210074,388.824206012441));
#56691=CARTESIAN_POINT('Origin',(263.115917770968,0.527992731210016,445.000000551893));
#56692=CARTESIAN_POINT('',(280.826883643896,0.527992731210079,382.979264601342));
#56693=CARTESIAN_POINT('Origin',(252.893297200846,0.527992731210083,387.52988588859));
#56694=CARTESIAN_POINT('',(278.788139374728,0.527992731210079,382.432984720845));
#56695=CARTESIAN_POINT('Origin',(263.115917770968,0.527992731210016,445.000000551893));
#56696=CARTESIAN_POINT('',(275.572407735156,0.527992731210079,387.325538187287));
#56697=CARTESIAN_POINT('Origin',(300.704024209595,0.527992731210052,400.340731580129));
#56698=CARTESIAN_POINT('',(273.67868286362,0.527992731210079,386.948852889924));
#56699=CARTESIAN_POINT('Origin',(263.115917770968,0.527992731210016,445.000000551893));
#56700=CARTESIAN_POINT('',(272.580033373339,0.527992731210083,381.198115659165));
#56701=CARTESIAN_POINT('Origin',(245.479397903495,0.527992731210083,389.355870423926));
#56702=CARTESIAN_POINT('',(270.487427011329,0.527992731210087,380.922618805139));
#56703=CARTESIAN_POINT('Origin',(263.115917770968,0.527992731210016,445.000000551893));
#56704=CARTESIAN_POINT('',(267.937812775926,0.527992731210079,386.193053004555));
#56705=CARTESIAN_POINT('Origin',(294.553248422101,0.527992731210061,395.816565410931));
#56706=CARTESIAN_POINT('',(266.011121685656,0.527992731210083,386.066770998723));
#56707=CARTESIAN_POINT('Origin',(263.115917770968,0.527992731210016,445.000000551893));
#56708=CARTESIAN_POINT('',(264.171249460876,0.527992731210087,380.508634656726));
#56709=CARTESIAN_POINT('Origin',(238.367264350844,0.527992731210083,392.133941453219));
#56710=CARTESIAN_POINT('',(262.060586081059,0.527992731210087,380.508634656726));
#56711=CARTESIAN_POINT('Origin',(263.115917770968,0.527992731210016,445.000000551893));
#56712=CARTESIAN_POINT('',(260.22071385628,0.527992731210083,386.066770998723));
#56713=CARTESIAN_POINT('Origin',(287.864571191091,0.527992731210065,392.133941453219));
#56714=CARTESIAN_POINT('',(258.294022766009,0.527992731210083,386.193053004555));
#56715=CARTESIAN_POINT('Origin',(263.115917770968,0.527992731210016,445.000000551893));
#56716=CARTESIAN_POINT('',(255.744408530606,0.527992731210092,380.922618805139));
#56717=CARTESIAN_POINT('Origin',(231.678587119835,0.527992731210083,395.816565410931));
#56718=CARTESIAN_POINT('',(253.651802168597,0.527992731210092,381.198115659165));
#56719=CARTESIAN_POINT('Origin',(263.115917770968,0.527992731210016,445.000000551893));
#56720=CARTESIAN_POINT('',(252.553152678315,0.527992731210087,386.948852889924));
#56721=CARTESIAN_POINT('Origin',(280.75243763844,0.527992731210074,389.355870423926));
#56722=CARTESIAN_POINT('',(250.659427806779,0.527992731210087,387.325538187287));
#56723=CARTESIAN_POINT('Origin',(263.115917770968,0.527992731210016,445.000000551893));
#56724=CARTESIAN_POINT('',(247.443696167207,0.527992731210092,382.432984720845));
#56725=CARTESIAN_POINT('Origin',(225.527811332341,0.527992731210079,400.340731580129));
#56726=CARTESIAN_POINT('',(245.40495189804,0.527992731210092,382.979264601342));
#56727=CARTESIAN_POINT('Origin',(263.115917770968,0.527992731210016,445.000000551893));
#56728=CARTESIAN_POINT('',(245.066323339638,0.527992731210087,388.824206012441));
#56729=CARTESIAN_POINT('Origin',(273.33853834109,0.527992731210079,387.52988588859));
#56730=CARTESIAN_POINT('',(243.237966844428,0.527992731210087,389.44484941146));
#56731=CARTESIAN_POINT('Origin',(263.115917770968,0.527992731210016,445.000000551893));
#56732=CARTESIAN_POINT('',(239.411139860609,0.527992731210092,385.013889624274));
#56733=CARTESIAN_POINT('Origin',(220.020178467404,0.527992731210074,405.629030223323));
#56734=CARTESIAN_POINT('',(237.461141163976,0.527992731210092,385.82160553103));
#56735=CARTESIAN_POINT('Origin',(263.115917770968,0.527992731210016,445.000000551893));
#56736=CARTESIAN_POINT('',(237.888327565974,0.527992731210087,391.6607425544));
#56737=CARTESIAN_POINT('Origin',(265.749727171539,0.527992731210079,386.687230948869));
#56738=CARTESIAN_POINT('',(236.156623133639,0.527992731210083,392.514724674444));
#56739=CARTESIAN_POINT('Origin',(263.115917770968,0.527992731210016,445.000000551893));
#56740=CARTESIAN_POINT('',(231.784178876264,0.527992731210092,388.621173516967));
#56741=CARTESIAN_POINT('Origin',(215.249925650347,0.52799273121007,411.590977084534));
#56742=CARTESIAN_POINT('',(229.956290770505,0.527992731210092,389.676505206876));
#56743=CARTESIAN_POINT('Origin',(263.115917770968,0.527992731210016,445.000000551893));
#56744=CARTESIAN_POINT('',(231.141982855127,0.527992731210083,395.409928589132));
#56745=CARTESIAN_POINT('Origin',(258.115850792914,0.527992731210083,386.84232366441));
#56746=CARTESIAN_POINT('',(229.536560428623,0.527992731210083,396.482637559359));
#56747=CARTESIAN_POINT('Origin',(263.115917770968,0.527992731210016,445.000000551893));
#56748=CARTESIAN_POINT('',(224.693312631206,0.527992731210087,393.193114771392));
#56749=CARTESIAN_POINT('Origin',(211.298673229435,0.527992731210065,418.124561600002));
#56750=CARTESIAN_POINT('',(223.018810788598,0.527992731210087,394.478005226645));
#56751=CARTESIAN_POINT('Origin',(263.115917770968,0.527992731210016,445.000000551893));
#56752=CARTESIAN_POINT('',(224.942721035539,0.527992731210079,400.007614504113));
#56753=CARTESIAN_POINT('Origin',(250.567526946565,0.527992731210083,387.99251035585));
#56754=CARTESIAN_POINT('',(223.491049837692,0.527992731210079,401.280695976629));
#56755=CARTESIAN_POINT('Origin',(263.115917770968,0.527992731210016,445.000000551893));
#56756=CARTESIAN_POINT('',(218.259867812848,0.527992731210083,398.651486205103));
#56757=CARTESIAN_POINT('Origin',(208.234028229082,0.527992731210061,425.117992327217));
#56758=CARTESIAN_POINT('',(216.767403424177,0.527992731210083,400.143950593773));
#56759=CARTESIAN_POINT('Origin',(263.115917770968,0.527992731210016,445.000000551893));
#56760=CARTESIAN_POINT('',(219.396613195704,0.527992731210079,405.375132618617));
#56761=CARTESIAN_POINT('Origin',(243.233909546291,0.527992731210083,390.118111010007));
#56762=CARTESIAN_POINT('',(218.123531723188,0.527992731210074,406.826803816464));
#56763=CARTESIAN_POINT('Origin',(263.115917770968,0.527992731210016,445.000000551893));
#56764=CARTESIAN_POINT('',(212.59392244572,0.527992731210079,404.902893569523));
#56765=CARTESIAN_POINT('Origin',(206.108427574925,0.527992731210052,432.45160972749));
#56766=CARTESIAN_POINT('',(211.309031990466,0.527992731210079,406.577395412131));
#56767=CARTESIAN_POINT('Origin',(263.115917770968,0.527992731210016,445.000000551893));
#56768=CARTESIAN_POINT('',(214.598554778433,0.52799273121007,411.420643209549));
#56769=CARTESIAN_POINT('Origin',(236.240478819077,0.527992731210083,393.18275601036));
#56770=CARTESIAN_POINT('',(213.525845808207,0.52799273121007,413.026065636052));
#56771=CARTESIAN_POINT('Origin',(263.115917770968,0.527992731210016,445.000000551893));
#56772=CARTESIAN_POINT('',(207.79242242595,0.527992731210074,411.840373551431));
#56773=CARTESIAN_POINT('Origin',(204.958240883485,0.527992731210043,439.99993357384));
#56774=CARTESIAN_POINT('',(206.737090736042,0.527992731210074,413.668261657189));
#56775=CARTESIAN_POINT('Origin',(263.115917770968,0.527992731210016,445.000000551893));
#56776=CARTESIAN_POINT('',(210.630641893519,0.527992731210065,418.040705914564));
#56777=CARTESIAN_POINT('Origin',(229.706894303608,0.527992731210083,397.134008431273));
#56778=CARTESIAN_POINT('',(209.776659773475,0.527992731210065,419.7724103469));
#56779=CARTESIAN_POINT('Origin',(263.115917770968,0.527992731210016,445.000000551893));
#56780=CARTESIAN_POINT('',(203.937522750105,0.527992731210065,419.345223944901));
#56781=CARTESIAN_POINT('Origin',(204.803148167944,0.527992731210034,447.633809952465));
#56782=CARTESIAN_POINT('',(203.129806843349,0.527992731210065,421.295222641535));
#56783=CARTESIAN_POINT('Origin',(263.115917770968,0.527992731210016,445.000000551893));
#56784=CARTESIAN_POINT('',(207.560766630535,0.527992731210061,425.122049625353));
#56785=CARTESIAN_POINT('Origin',(223.744947442398,0.527992731210079,401.904261248329));
#56786=CARTESIAN_POINT('',(206.940123231516,0.527992731210056,426.950406120564));
#56787=CARTESIAN_POINT('Origin',(263.115917770968,0.527992731210016,445.000000551893));
#56788=CARTESIAN_POINT('',(201.095181820417,0.527992731210061,427.289034678965));
#56789=CARTESIAN_POINT('Origin',(205.645803107665,0.527992731210025,455.222621122016));
#56790=CARTESIAN_POINT('',(200.54890193992,0.527992731210056,429.327778948133));
#56791=CARTESIAN_POINT('Origin',(263.115917770968,0.527992731210016,445.000000551893));
#56792=CARTESIAN_POINT('',(205.441455406362,0.527992731210052,432.543510587705));
#56793=CARTESIAN_POINT('Origin',(218.456648799204,0.527992731210074,407.411894113266));
#56794=CARTESIAN_POINT('',(205.064770108999,0.527992731210047,434.437235459241));
#56795=CARTESIAN_POINT('Origin',(263.115917770968,0.527992731210016,445.000000551893));
#56796=CARTESIAN_POINT('',(199.31403287824,0.527992731210052,435.535884949523));
#56797=CARTESIAN_POINT('Origin',(207.471787643001,0.527992731210016,462.636520419366));
#56798=CARTESIAN_POINT('',(199.038536024214,0.527992731210047,437.628491311532));
#56799=CARTESIAN_POINT('Origin',(263.115917770968,0.527992731210016,445.000000551893));
#56800=CARTESIAN_POINT('',(204.30897022363,0.527992731210043,440.178105546935));
#56801=CARTESIAN_POINT('Origin',(213.932482630006,0.52799273121007,413.56266990076));
#56802=CARTESIAN_POINT('',(204.182688217798,0.527992731210043,442.104796637205));
#56803=CARTESIAN_POINT('Origin',(263.115917770968,0.527992731210016,445.000000551893));
#56804=CARTESIAN_POINT('',(198.624551875801,0.527992731210043,443.944668861985));
#56805=CARTESIAN_POINT('Origin',(210.249858672294,0.527992731210007,469.748653972017));
#56806=CARTESIAN_POINT('',(198.624551875801,0.527992731210039,446.055332241802));
#56807=CARTESIAN_POINT('Origin',(263.115917770968,0.527992731210016,445.000000551893));
#56808=CARTESIAN_POINT('',(204.182688217798,0.527992731210034,447.895204466582));
#56809=CARTESIAN_POINT('Origin',(210.249858672294,0.527992731210065,420.25134713177));
#56810=CARTESIAN_POINT('',(204.30897022363,0.527992731210034,449.821895556852));
#56811=CARTESIAN_POINT('Origin',(263.115917770968,0.527992731210016,445.000000551893));
#56812=CARTESIAN_POINT('',(199.038536024214,0.52799273121003,452.371509792255));
#56813=CARTESIAN_POINT('Origin',(213.932482630006,0.527992731209999,476.437331203026));
#56814=CARTESIAN_POINT('Origin',(263.115917770968,0.527992731210016,445.000000551893));
#56815=CARTESIAN_POINT('Origin',(282.115917770968,0.527992731210016,439.000000551893));
#56816=CARTESIAN_POINT('',(282.115917770968,-19.47200726879,451.000000551893));
#56817=CARTESIAN_POINT('',(282.115917770968,-19.47200726879,439.000000551893));
#56818=CARTESIAN_POINT('',(282.115917770968,-19.47200726879,442.000000551893));
#56819=CARTESIAN_POINT('',(282.115917770968,0.527992731210003,451.000000551893));
#56820=CARTESIAN_POINT('',(282.115917770968,0.527992731210016,439.000000551893));
#56821=CARTESIAN_POINT('Origin',(274.115917770968,0.527992731210021,439.000000551893));
#56822=CARTESIAN_POINT('',(276.863644855836,-19.47200726879,439.000000551893));
#56823=CARTESIAN_POINT('',(268.615917770968,-19.47200726879,439.000000551893));
#56824=CARTESIAN_POINT('',(276.863644855836,0.527992731210016,439.000000551893));
#56825=CARTESIAN_POINT('Origin',(263.115917770968,0.527992731210016,445.000000551893));
#56826=CARTESIAN_POINT('',(276.863644855836,-19.47200726879,451.000000551893));
#56827=CARTESIAN_POINT('Origin',(263.115917770968,-19.47200726879,445.000000551893));
#56828=CARTESIAN_POINT('',(276.863644855836,0.527992731210005,451.000000551893));
#56829=CARTESIAN_POINT('Origin',(282.115917770968,0.527992731210003,451.000000551893));
#56830=CARTESIAN_POINT('',(272.615917770968,-19.47200726879,451.000000551893));
#56831=CARTESIAN_POINT('Origin',(263.115917770968,-19.47200726879,445.000000551893));
#56832=CARTESIAN_POINT('',(205.064770108999,-19.47200726879,455.562765644546));
#56833=CARTESIAN_POINT('',(205.064770108999,-19.47200726879,455.562765644546));
#56834=CARTESIAN_POINT('',(205.441455406362,-19.47200726879,457.456490516082));
#56835=CARTESIAN_POINT('Origin',(263.115917770968,-19.47200726879,445.000000551893));
#56836=CARTESIAN_POINT('',(205.441455406362,-19.47200726879,457.456490516082));
#56837=CARTESIAN_POINT('Origin',(218.456648799204,-19.47200726879,482.58810699052));
#56838=CARTESIAN_POINT('',(200.54890193992,-19.47200726879,460.672222155654));
#56839=CARTESIAN_POINT('Origin',(218.456648799204,-19.47200726879,482.58810699052));
#56840=CARTESIAN_POINT('',(200.54890193992,-19.47200726879,460.672222155654));
#56841=CARTESIAN_POINT('Origin',(207.471787643001,-19.4720072687899,427.363480684421));
#56842=CARTESIAN_POINT('',(199.31403287824,-19.47200726879,454.464116154264));
#56843=CARTESIAN_POINT('',(199.31403287824,-19.47200726879,454.464116154264));
#56844=CARTESIAN_POINT('Origin',(207.471787643001,-19.4720072687899,427.363480684421));
#56845=CARTESIAN_POINT('Origin',(263.115917770968,-19.47200726879,445.000000551893));
#56846=CARTESIAN_POINT('',(206.940123231516,-19.47200726879,463.049594983223));
#56847=CARTESIAN_POINT('',(206.940123231516,-19.47200726879,463.049594983223));
#56848=CARTESIAN_POINT('',(207.560766630536,-19.47200726879,464.877951478433));
#56849=CARTESIAN_POINT('Origin',(263.115917770968,-19.47200726879,445.000000551893));
#56850=CARTESIAN_POINT('',(207.560766630536,-19.47200726879,464.877951478433));
#56851=CARTESIAN_POINT('Origin',(223.744947442398,-19.47200726879,488.095739855457));
#56852=CARTESIAN_POINT('',(203.129806843349,-19.47200726879,468.704778462252));
#56853=CARTESIAN_POINT('Origin',(223.744947442398,-19.47200726879,488.095739855457));
#56854=CARTESIAN_POINT('',(203.129806843349,-19.47200726879,468.704778462252));
#56855=CARTESIAN_POINT('Origin',(205.645803107665,-19.47200726879,434.777379981771));
#56856=CARTESIAN_POINT('',(201.095181820417,-19.47200726879,462.710966424822));
#56857=CARTESIAN_POINT('',(201.095181820417,-19.47200726879,462.710966424822));
#56858=CARTESIAN_POINT('Origin',(205.645803107665,-19.47200726879,434.777379981771));
#56859=CARTESIAN_POINT('Origin',(263.115917770968,-19.47200726879,445.000000551893));
#56860=CARTESIAN_POINT('',(209.776659773475,-19.47200726879,470.227590756887));
#56861=CARTESIAN_POINT('',(209.776659773475,-19.47200726879,470.227590756887));
#56862=CARTESIAN_POINT('',(210.630641893519,-19.47200726879,471.959295189222));
#56863=CARTESIAN_POINT('Origin',(263.115917770968,-19.47200726879,445.000000551893));
#56864=CARTESIAN_POINT('',(210.630641893519,-19.47200726879,471.959295189222));
#56865=CARTESIAN_POINT('Origin',(229.706894303609,-19.47200726879,492.865992672514));
#56866=CARTESIAN_POINT('',(206.737090736042,-19.47200726879,476.331739446597));
#56867=CARTESIAN_POINT('Origin',(229.706894303609,-19.47200726879,492.865992672514));
#56868=CARTESIAN_POINT('',(206.737090736042,-19.47200726879,476.331739446597));
#56869=CARTESIAN_POINT('Origin',(204.803148167944,-19.47200726879,442.366191151322));
#56870=CARTESIAN_POINT('',(203.937522750105,-19.47200726879,470.654777158886));
#56871=CARTESIAN_POINT('',(203.937522750105,-19.47200726879,470.654777158886));
#56872=CARTESIAN_POINT('Origin',(204.803148167944,-19.47200726879,442.366191151322));
#56873=CARTESIAN_POINT('Origin',(263.115917770968,-19.47200726879,445.000000551893));
#56874=CARTESIAN_POINT('',(213.525845808207,-19.47200726879,476.973935467734));
#56875=CARTESIAN_POINT('',(213.525845808207,-19.47200726879,476.973935467734));
#56876=CARTESIAN_POINT('',(214.598554778434,-19.47200726879,478.579357894238));
#56877=CARTESIAN_POINT('Origin',(263.115917770968,-19.47200726879,445.000000551893));
#56878=CARTESIAN_POINT('',(214.598554778434,-19.47200726879,478.579357894238));
#56879=CARTESIAN_POINT('Origin',(236.240478819077,-19.47200726879,496.817245093427));
#56880=CARTESIAN_POINT('',(211.309031990467,-19.47200726879,483.422605691655));
#56881=CARTESIAN_POINT('Origin',(236.240478819077,-19.47200726879,496.817245093427));
#56882=CARTESIAN_POINT('',(211.309031990467,-19.47200726879,483.422605691655));
#56883=CARTESIAN_POINT('Origin',(204.958240883485,-19.47200726879,450.000067529947));
#56884=CARTESIAN_POINT('',(207.792422425951,-19.47200726879,478.159627552356));
#56885=CARTESIAN_POINT('',(207.792422425951,-19.47200726879,478.159627552356));
#56886=CARTESIAN_POINT('Origin',(204.958240883485,-19.47200726879,450.000067529947));
#56887=CARTESIAN_POINT('Origin',(263.115917770968,-19.47200726879,445.000000551893));
#56888=CARTESIAN_POINT('',(218.123531723188,-19.47200726879,483.173197287322));
#56889=CARTESIAN_POINT('',(218.123531723188,-19.47200726879,483.173197287322));
#56890=CARTESIAN_POINT('',(219.396613195705,-19.47200726879,484.624868485169));
#56891=CARTESIAN_POINT('Origin',(263.115917770968,-19.47200726879,445.000000551893));
#56892=CARTESIAN_POINT('',(219.396613195705,-19.47200726879,484.624868485169));
#56893=CARTESIAN_POINT('Origin',(243.233909546292,-19.47200726879,499.881890093779));
#56894=CARTESIAN_POINT('',(216.767403424178,-19.47200726879,489.856050510013));
#56895=CARTESIAN_POINT('Origin',(243.233909546292,-19.47200726879,499.881890093779));
#56896=CARTESIAN_POINT('',(216.767403424178,-19.47200726879,489.856050510013));
#56897=CARTESIAN_POINT('Origin',(206.108427574925,-19.47200726879,457.548391376297));
#56898=CARTESIAN_POINT('',(212.59392244572,-19.47200726879,485.097107534263));
#56899=CARTESIAN_POINT('',(212.59392244572,-19.47200726879,485.097107534263));
#56900=CARTESIAN_POINT('Origin',(206.108427574925,-19.47200726879,457.548391376297));
#56901=CARTESIAN_POINT('Origin',(263.115917770968,-19.47200726879,445.000000551893));
#56902=CARTESIAN_POINT('',(223.491049837692,-19.47200726879,488.719305127157));
#56903=CARTESIAN_POINT('',(223.491049837692,-19.47200726879,488.719305127157));
#56904=CARTESIAN_POINT('',(224.94272103554,-19.47200726879,489.992386599674));
#56905=CARTESIAN_POINT('Origin',(263.115917770968,-19.47200726879,445.000000551893));
#56906=CARTESIAN_POINT('',(224.94272103554,-19.47200726879,489.992386599674));
#56907=CARTESIAN_POINT('Origin',(250.567526946565,-19.47200726879,502.007490747936));
#56908=CARTESIAN_POINT('',(223.018810788598,-19.47200726879,495.521995877141));
#56909=CARTESIAN_POINT('Origin',(250.567526946565,-19.47200726879,502.007490747936));
#56910=CARTESIAN_POINT('',(223.018810788598,-19.47200726879,495.521995877141));
#56911=CARTESIAN_POINT('Origin',(208.234028229082,-19.47200726879,464.88200877657));
#56912=CARTESIAN_POINT('',(218.259867812848,-19.47200726879,491.348514898684));
#56913=CARTESIAN_POINT('',(218.259867812848,-19.47200726879,491.348514898684));
#56914=CARTESIAN_POINT('Origin',(208.234028229082,-19.47200726879,464.88200877657));
#56915=CARTESIAN_POINT('Origin',(263.115917770968,-19.47200726879,445.000000551893));
#56916=CARTESIAN_POINT('',(229.536560428624,-19.47200726879,493.517363544428));
#56917=CARTESIAN_POINT('',(229.536560428624,-19.47200726879,493.517363544428));
#56918=CARTESIAN_POINT('',(231.141982855127,-19.47200726879,494.590072514654));
#56919=CARTESIAN_POINT('Origin',(263.115917770968,-19.47200726879,445.000000551893));
#56920=CARTESIAN_POINT('',(231.141982855127,-19.47200726879,494.590072514654));
#56921=CARTESIAN_POINT('Origin',(258.115850792915,-19.47200726879,503.157677439376));
#56922=CARTESIAN_POINT('',(229.956290770506,-19.47200726879,500.323495896911));
#56923=CARTESIAN_POINT('Origin',(258.115850792915,-19.47200726879,503.157677439376));
#56924=CARTESIAN_POINT('',(229.956290770506,-19.47200726879,500.323495896911));
#56925=CARTESIAN_POINT('Origin',(211.298673229435,-19.47200726879,471.875439503784));
#56926=CARTESIAN_POINT('',(224.693312631207,-19.47200726879,496.806886332395));
#56927=CARTESIAN_POINT('',(224.693312631207,-19.47200726879,496.806886332395));
#56928=CARTESIAN_POINT('Origin',(211.298673229435,-19.47200726879,471.875439503784));
#56929=CARTESIAN_POINT('Origin',(263.115917770968,-19.47200726879,445.000000551893));
#56930=CARTESIAN_POINT('',(236.15662313364,-19.47200726879,497.485276429342));
#56931=CARTESIAN_POINT('',(236.15662313364,-19.47200726879,497.485276429342));
#56932=CARTESIAN_POINT('',(237.888327565975,-19.47200726879,498.339258549387));
#56933=CARTESIAN_POINT('Origin',(263.115917770968,-19.47200726879,445.000000551893));
#56934=CARTESIAN_POINT('',(237.888327565975,-19.47200726879,498.339258549387));
#56935=CARTESIAN_POINT('Origin',(265.74972717154,-19.4720072687901,503.312770154917));
#56936=CARTESIAN_POINT('',(237.461141163976,-19.47200726879,504.178395572756));
#56937=CARTESIAN_POINT('Origin',(265.74972717154,-19.4720072687901,503.312770154917));
#56938=CARTESIAN_POINT('',(237.461141163976,-19.47200726879,504.178395572756));
#56939=CARTESIAN_POINT('Origin',(215.249925650348,-19.47200726879,478.409024019253));
#56940=CARTESIAN_POINT('',(231.784178876265,-19.47200726879,501.378827586819));
#56941=CARTESIAN_POINT('',(231.784178876265,-19.47200726879,501.378827586819));
#56942=CARTESIAN_POINT('Origin',(215.249925650348,-19.47200726879,478.409024019253));
#56943=CARTESIAN_POINT('Origin',(263.115917770968,-19.47200726879,445.000000551893));
#56944=CARTESIAN_POINT('',(243.237966844429,-19.47200726879,500.555151692326));
#56945=CARTESIAN_POINT('',(243.237966844429,-19.47200726879,500.555151692326));
#56946=CARTESIAN_POINT('',(245.066323339639,-19.47200726879,501.175795091346));
#56947=CARTESIAN_POINT('Origin',(263.115917770968,-19.47200726879,445.000000551893));
#56948=CARTESIAN_POINT('',(245.066323339639,-19.47200726879,501.175795091346));
#56949=CARTESIAN_POINT('Origin',(273.338538341091,-19.4720072687901,502.470115215196));
#56950=CARTESIAN_POINT('',(245.40495189804,-19.47200726879,507.020736502444));
#56951=CARTESIAN_POINT('Origin',(273.338538341091,-19.4720072687901,502.470115215196));
#56952=CARTESIAN_POINT('',(245.40495189804,-19.47200726879,507.020736502444));
#56953=CARTESIAN_POINT('Origin',(220.020178467404,-19.47200726879,484.370970880464));
#56954=CARTESIAN_POINT('',(239.41113986061,-19.47200726879,504.986111479512));
#56955=CARTESIAN_POINT('',(239.41113986061,-19.47200726879,504.986111479512));
#56956=CARTESIAN_POINT('Origin',(220.020178467404,-19.47200726879,484.370970880464));
#56957=CARTESIAN_POINT('Origin',(263.115917770968,-19.47200726879,445.000000551893));
#56958=CARTESIAN_POINT('',(250.65942780678,-19.47200726879,502.674462916499));
#56959=CARTESIAN_POINT('',(250.65942780678,-19.47200726879,502.674462916499));
#56960=CARTESIAN_POINT('',(252.553152678316,-19.47200726879,503.051148213862));
#56961=CARTESIAN_POINT('Origin',(263.115917770968,-19.47200726879,445.000000551893));
#56962=CARTESIAN_POINT('',(252.553152678316,-19.47200726879,503.051148213862));
#56963=CARTESIAN_POINT('Origin',(280.752437638441,-19.4720072687901,500.64413067986));
#56964=CARTESIAN_POINT('',(253.651802168598,-19.4720072687901,508.801885444622));
#56965=CARTESIAN_POINT('Origin',(280.752437638441,-19.4720072687901,500.64413067986));
#56966=CARTESIAN_POINT('',(253.651802168598,-19.4720072687901,508.801885444622));
#56967=CARTESIAN_POINT('Origin',(225.527811332342,-19.47200726879,489.659269523657));
#56968=CARTESIAN_POINT('',(247.443696167208,-19.47200726879,507.567016382941));
#56969=CARTESIAN_POINT('',(247.443696167208,-19.47200726879,507.567016382941));
#56970=CARTESIAN_POINT('Origin',(225.527811332342,-19.47200726879,489.659269523657));
#56971=CARTESIAN_POINT('Origin',(263.115917770968,-19.47200726879,445.000000551893));
#56972=CARTESIAN_POINT('',(258.29402276601,-19.47200726879,503.806948099231));
#56973=CARTESIAN_POINT('',(258.29402276601,-19.47200726879,503.806948099231));
#56974=CARTESIAN_POINT('',(260.22071385628,-19.47200726879,503.933230105063));
#56975=CARTESIAN_POINT('Origin',(263.115917770968,-19.47200726879,445.000000551893));
#56976=CARTESIAN_POINT('',(260.22071385628,-19.47200726879,503.933230105063));
#56977=CARTESIAN_POINT('Origin',(287.864571191092,-19.4720072687901,497.866059650567));
#56978=CARTESIAN_POINT('',(262.06058608106,-19.4720072687901,509.49136644706));
#56979=CARTESIAN_POINT('Origin',(287.864571191092,-19.4720072687901,497.866059650567));
#56980=CARTESIAN_POINT('',(262.06058608106,-19.4720072687901,509.49136644706));
#56981=CARTESIAN_POINT('Origin',(231.678587119835,-19.47200726879,494.183435692855));
#56982=CARTESIAN_POINT('',(255.744408530607,-19.4720072687901,509.077382298647));
#56983=CARTESIAN_POINT('',(255.744408530607,-19.4720072687901,509.077382298647));
#56984=CARTESIAN_POINT('Origin',(231.678587119835,-19.47200726879,494.183435692855));
#56985=CARTESIAN_POINT('Origin',(263.115917770968,-19.47200726879,445.000000551893));
#56986=CARTESIAN_POINT('',(266.011121685657,-19.4720072687901,503.933230105063));
#56987=CARTESIAN_POINT('',(266.011121685657,-19.4720072687901,503.933230105063));
#56988=CARTESIAN_POINT('',(267.937812775927,-19.4720072687901,503.806948099231));
#56989=CARTESIAN_POINT('Origin',(263.115917770968,-19.47200726879,445.000000551893));
#56990=CARTESIAN_POINT('',(267.937812775927,-19.4720072687901,503.806948099231));
#56991=CARTESIAN_POINT('Origin',(294.553248422101,-19.4720072687901,494.183435692855));
#56992=CARTESIAN_POINT('',(270.48742701133,-19.4720072687901,509.077382298647));
#56993=CARTESIAN_POINT('Origin',(294.553248422101,-19.4720072687901,494.183435692855));
#56994=CARTESIAN_POINT('',(270.48742701133,-19.4720072687901,509.077382298647));
#56995=CARTESIAN_POINT('Origin',(238.367264350845,-19.47200726879,497.866059650567));
#56996=CARTESIAN_POINT('',(264.171249460877,-19.4720072687901,509.49136644706));
#56997=CARTESIAN_POINT('',(264.171249460877,-19.4720072687901,509.49136644706));
#56998=CARTESIAN_POINT('Origin',(238.367264350845,-19.47200726879,497.866059650567));
#56999=CARTESIAN_POINT('Origin',(263.115917770968,-19.47200726879,445.000000551893));
#57000=CARTESIAN_POINT('',(273.678682863621,-19.4720072687901,503.051148213862));
#57001=CARTESIAN_POINT('',(273.678682863621,-19.4720072687901,503.051148213862));
#57002=CARTESIAN_POINT('',(275.572407735157,-19.4720072687901,502.674462916499));
#57003=CARTESIAN_POINT('Origin',(263.115917770968,-19.47200726879,445.000000551893));
#57004=CARTESIAN_POINT('',(275.572407735157,-19.4720072687901,502.674462916499));
#57005=CARTESIAN_POINT('Origin',(300.704024209595,-19.47200726879,489.659269523657));
#57006=CARTESIAN_POINT('',(278.788139374729,-19.4720072687901,507.567016382941));
#57007=CARTESIAN_POINT('Origin',(300.704024209595,-19.47200726879,489.659269523657));
#57008=CARTESIAN_POINT('',(278.788139374729,-19.4720072687901,507.567016382941));
#57009=CARTESIAN_POINT('Origin',(245.479397903496,-19.47200726879,500.64413067986));
#57010=CARTESIAN_POINT('',(272.580033373339,-19.4720072687901,508.801885444621));
#57011=CARTESIAN_POINT('',(272.580033373339,-19.4720072687901,508.801885444621));
#57012=CARTESIAN_POINT('Origin',(245.479397903496,-19.47200726879,500.64413067986));
#57013=CARTESIAN_POINT('Origin',(263.115917770968,-19.47200726879,445.000000551893));
#57014=CARTESIAN_POINT('',(281.165512202298,-19.4720072687901,501.175795091345));
#57015=CARTESIAN_POINT('',(281.165512202298,-19.4720072687901,501.175795091345));
#57016=CARTESIAN_POINT('',(282.993868697508,-19.4720072687901,500.555151692326));
#57017=CARTESIAN_POINT('Origin',(263.115917770968,-19.47200726879,445.000000551893));
#57018=CARTESIAN_POINT('',(282.993868697508,-19.4720072687901,500.555151692326));
#57019=CARTESIAN_POINT('Origin',(306.211657074532,-19.47200726879,484.370970880463));
#57020=CARTESIAN_POINT('',(286.820695681327,-19.4720072687901,504.986111479512));
#57021=CARTESIAN_POINT('Origin',(306.211657074532,-19.47200726879,484.370970880463));
#57022=CARTESIAN_POINT('',(286.820695681327,-19.4720072687901,504.986111479512));
#57023=CARTESIAN_POINT('Origin',(252.893297200846,-19.47200726879,502.470115215196));
#57024=CARTESIAN_POINT('',(280.826883643897,-19.4720072687901,507.020736502444));
#57025=CARTESIAN_POINT('',(280.826883643897,-19.4720072687901,507.020736502444));
#57026=CARTESIAN_POINT('Origin',(252.893297200846,-19.47200726879,502.470115215196));
#57027=CARTESIAN_POINT('Origin',(263.115917770968,-19.47200726879,445.000000551893));
#57028=CARTESIAN_POINT('',(288.343507975962,-19.4720072687901,498.339258549386));
#57029=CARTESIAN_POINT('',(288.343507975962,-19.4720072687901,498.339258549386));
#57030=CARTESIAN_POINT('',(290.075212408297,-19.4720072687901,497.485276429342));
#57031=CARTESIAN_POINT('Origin',(263.115917770968,-19.47200726879,445.000000551893));
#57032=CARTESIAN_POINT('',(290.075212408297,-19.4720072687901,497.485276429342));
#57033=CARTESIAN_POINT('Origin',(310.981909891589,-19.47200726879,478.409024019252));
#57034=CARTESIAN_POINT('',(294.447656665672,-19.4720072687901,501.378827586819));
#57035=CARTESIAN_POINT('Origin',(310.981909891589,-19.47200726879,478.409024019252));
#57036=CARTESIAN_POINT('',(294.447656665672,-19.4720072687901,501.378827586819));
#57037=CARTESIAN_POINT('Origin',(260.482108370397,-19.47200726879,503.312770154917));
#57038=CARTESIAN_POINT('',(288.770694377961,-19.4720072687901,504.178395572756));
#57039=CARTESIAN_POINT('',(288.770694377961,-19.4720072687901,504.178395572756));
#57040=CARTESIAN_POINT('Origin',(260.482108370397,-19.47200726879,503.312770154917));
#57041=CARTESIAN_POINT('Origin',(263.115917770968,-19.47200726879,445.000000551893));
#57042=CARTESIAN_POINT('',(295.089852686809,-19.4720072687901,494.590072514654));
#57043=CARTESIAN_POINT('',(295.089852686809,-19.4720072687901,494.590072514654));
#57044=CARTESIAN_POINT('',(296.695275113313,-19.4720072687901,493.517363544428));
#57045=CARTESIAN_POINT('Origin',(263.115917770968,-19.47200726879,445.000000551893));
#57046=CARTESIAN_POINT('',(296.695275113313,-19.4720072687901,493.517363544428));
#57047=CARTESIAN_POINT('Origin',(314.933162312502,-19.47200726879,471.875439503784));
#57048=CARTESIAN_POINT('',(301.53852291073,-19.4720072687901,496.806886332394));
#57049=CARTESIAN_POINT('Origin',(314.933162312502,-19.47200726879,471.875439503784));
#57050=CARTESIAN_POINT('',(301.53852291073,-19.4720072687901,496.806886332394));
#57051=CARTESIAN_POINT('Origin',(268.115984749022,-19.4720072687901,503.157677439376));
#57052=CARTESIAN_POINT('',(296.275544771431,-19.4720072687901,500.32349589691));
#57053=CARTESIAN_POINT('',(296.275544771431,-19.4720072687901,500.32349589691));
#57054=CARTESIAN_POINT('Origin',(268.115984749022,-19.4720072687901,503.157677439376));
#57055=CARTESIAN_POINT('Origin',(263.115917770968,-19.47200726879,445.000000551893));
#57056=CARTESIAN_POINT('',(301.289114506397,-19.47200726879,489.992386599673));
#57057=CARTESIAN_POINT('',(301.289114506397,-19.47200726879,489.992386599673));
#57058=CARTESIAN_POINT('',(302.740785704245,-19.47200726879,488.719305127157));
#57059=CARTESIAN_POINT('Origin',(263.115917770968,-19.47200726879,445.000000551893));
#57060=CARTESIAN_POINT('',(302.740785704245,-19.47200726879,488.719305127157));
#57061=CARTESIAN_POINT('Origin',(317.997807312854,-19.47200726879,464.882008776569));
#57062=CARTESIAN_POINT('',(307.971967729088,-19.4720072687901,491.348514898683));
#57063=CARTESIAN_POINT('Origin',(317.997807312854,-19.47200726879,464.882008776569));
#57064=CARTESIAN_POINT('',(307.971967729088,-19.4720072687901,491.348514898683));
#57065=CARTESIAN_POINT('Origin',(275.664308595372,-19.4720072687901,502.007490747936));
#57066=CARTESIAN_POINT('',(303.213024753338,-19.4720072687901,495.521995877141));
#57067=CARTESIAN_POINT('',(303.213024753338,-19.4720072687901,495.521995877141));
#57068=CARTESIAN_POINT('Origin',(275.664308595372,-19.4720072687901,502.007490747936));
#57069=CARTESIAN_POINT('Origin',(263.115917770968,-19.47200726879,445.000000551893));
#57070=CARTESIAN_POINT('',(306.835222346232,-19.47200726879,484.624868485169));
#57071=CARTESIAN_POINT('',(306.835222346232,-19.47200726879,484.624868485169));
#57072=CARTESIAN_POINT('',(308.108303818749,-19.47200726879,483.173197287322));
#57073=CARTESIAN_POINT('Origin',(263.115917770968,-19.47200726879,445.000000551893));
#57074=CARTESIAN_POINT('',(308.108303818749,-19.47200726879,483.173197287322));
#57075=CARTESIAN_POINT('Origin',(320.123407967011,-19.47200726879,457.548391376296));
#57076=CARTESIAN_POINT('',(313.637913096216,-19.47200726879,485.097107534263));
#57077=CARTESIAN_POINT('Origin',(320.123407967011,-19.47200726879,457.548391376296));
#57078=CARTESIAN_POINT('',(313.637913096216,-19.47200726879,485.097107534263));
#57079=CARTESIAN_POINT('Origin',(282.997925995645,-19.4720072687901,499.881890093779));
#57080=CARTESIAN_POINT('',(309.464432117759,-19.4720072687901,489.856050510013));
#57081=CARTESIAN_POINT('',(309.464432117759,-19.4720072687901,489.856050510013));
#57082=CARTESIAN_POINT('Origin',(282.997925995645,-19.4720072687901,499.881890093779));
#57083=CARTESIAN_POINT('Origin',(263.115917770968,-19.47200726879,445.000000551893));
#57084=CARTESIAN_POINT('',(311.633280763503,-19.47200726879,478.579357894237));
#57085=CARTESIAN_POINT('',(311.633280763503,-19.47200726879,478.579357894237));
#57086=CARTESIAN_POINT('',(312.705989733729,-19.47200726879,476.973935467734));
#57087=CARTESIAN_POINT('Origin',(263.115917770968,-19.47200726879,445.000000551893));
#57088=CARTESIAN_POINT('',(312.705989733729,-19.47200726879,476.973935467734));
#57089=CARTESIAN_POINT('Origin',(321.273594658451,-19.47200726879,450.000067529946));
#57090=CARTESIAN_POINT('',(318.439413115986,-19.47200726879,478.159627552356));
#57091=CARTESIAN_POINT('Origin',(321.273594658451,-19.47200726879,450.000067529946));
#57092=CARTESIAN_POINT('',(318.439413115986,-19.47200726879,478.159627552356));
#57093=CARTESIAN_POINT('Origin',(289.99135672286,-19.4720072687901,496.817245093426));
#57094=CARTESIAN_POINT('',(314.92280355147,-19.47200726879,483.422605691655));
#57095=CARTESIAN_POINT('',(314.92280355147,-19.47200726879,483.422605691655));
#57096=CARTESIAN_POINT('Origin',(289.99135672286,-19.4720072687901,496.817245093426));
#57097=CARTESIAN_POINT('Origin',(263.115917770968,-19.47200726879,445.000000551893));
#57098=CARTESIAN_POINT('',(315.601193648417,-19.47200726879,471.959295189222));
#57099=CARTESIAN_POINT('',(315.601193648417,-19.47200726879,471.959295189222));
#57100=CARTESIAN_POINT('',(316.455175768462,-19.47200726879,470.227590756886));
#57101=CARTESIAN_POINT('Origin',(263.115917770968,-19.47200726879,445.000000551893));
#57102=CARTESIAN_POINT('',(316.455175768462,-19.47200726879,470.227590756886));
#57103=CARTESIAN_POINT('Origin',(321.428687373992,-19.47200726879,442.366191151322));
#57104=CARTESIAN_POINT('',(322.294312791831,-19.47200726879,470.654777158885));
#57105=CARTESIAN_POINT('Origin',(321.428687373992,-19.47200726879,442.366191151322));
#57106=CARTESIAN_POINT('',(322.294312791831,-19.47200726879,470.654777158885));
#57107=CARTESIAN_POINT('Origin',(296.524941238328,-19.4720072687901,492.865992672513));
#57108=CARTESIAN_POINT('',(319.494744805894,-19.47200726879,476.331739446597));
#57109=CARTESIAN_POINT('',(319.494744805894,-19.47200726879,476.331739446597));
#57110=CARTESIAN_POINT('Origin',(296.524941238328,-19.4720072687901,492.865992672513));
#57111=CARTESIAN_POINT('Origin',(263.115917770968,-19.47200726879,445.000000551893));
#57112=CARTESIAN_POINT('',(318.671068911401,-19.47200726879,464.877951478433));
#57113=CARTESIAN_POINT('',(318.671068911401,-19.47200726879,464.877951478433));
#57114=CARTESIAN_POINT('',(319.291712310421,-19.47200726879,463.049594983222));
#57115=CARTESIAN_POINT('Origin',(263.115917770968,-19.47200726879,445.000000551893));
#57116=CARTESIAN_POINT('',(319.291712310421,-19.47200726879,463.049594983222));
#57117=CARTESIAN_POINT('Origin',(320.586032434271,-19.47200726879,434.77737998177));
#57118=CARTESIAN_POINT('',(325.136653721519,-19.47200726879,462.710966424821));
#57119=CARTESIAN_POINT('Origin',(320.586032434271,-19.47200726879,434.77737998177));
#57120=CARTESIAN_POINT('',(325.136653721519,-19.47200726879,462.710966424821));
#57121=CARTESIAN_POINT('Origin',(302.486888099539,-19.47200726879,488.095739855457));
#57122=CARTESIAN_POINT('',(323.102028698587,-19.47200726879,468.704778462251));
#57123=CARTESIAN_POINT('',(323.102028698587,-19.47200726879,468.704778462251));
#57124=CARTESIAN_POINT('Origin',(302.486888099539,-19.47200726879,488.095739855457));
#57125=CARTESIAN_POINT('Origin',(263.115917770968,-19.47200726879,445.000000551893));
#57126=CARTESIAN_POINT('',(320.790380135574,-19.47200726879,457.456490516081));
#57127=CARTESIAN_POINT('',(320.790380135574,-19.47200726879,457.456490516081));
#57128=CARTESIAN_POINT('',(321.167065432937,-19.47200726879,455.562765644545));
#57129=CARTESIAN_POINT('Origin',(263.115917770968,-19.47200726879,445.000000551893));
#57130=CARTESIAN_POINT('',(321.167065432937,-19.47200726879,455.562765644545));
#57131=CARTESIAN_POINT('Origin',(318.760047898935,-19.47200726879,427.36348068442));
#57132=CARTESIAN_POINT('',(326.917802663697,-19.47200726879,454.464116154263));
#57133=CARTESIAN_POINT('Origin',(318.760047898935,-19.47200726879,427.36348068442));
#57134=CARTESIAN_POINT('',(326.917802663697,-19.47200726879,454.464116154263));
#57135=CARTESIAN_POINT('Origin',(307.775186742732,-19.47200726879,482.588106990519));
#57136=CARTESIAN_POINT('',(325.682933602016,-19.47200726879,460.672222155653));
#57137=CARTESIAN_POINT('',(325.682933602016,-19.47200726879,460.672222155653));
#57138=CARTESIAN_POINT('Origin',(307.775186742732,-19.47200726879,482.588106990519));
#57139=CARTESIAN_POINT('Origin',(263.115917770968,-19.47200726879,445.000000551893));
#57140=CARTESIAN_POINT('',(321.922865318307,-19.47200726879,449.821895556851));
#57141=CARTESIAN_POINT('',(321.922865318307,-19.47200726879,449.821895556851));
#57142=CARTESIAN_POINT('',(322.049147324138,-19.47200726879,447.895204466581));
#57143=CARTESIAN_POINT('Origin',(263.115917770968,-19.47200726879,445.000000551893));
#57144=CARTESIAN_POINT('',(322.049147324138,-19.47200726879,447.895204466581));
#57145=CARTESIAN_POINT('Origin',(315.981976869642,-19.47200726879,420.251347131769));
#57146=CARTESIAN_POINT('',(327.607283666135,-19.47200726879,446.055332241801));
#57147=CARTESIAN_POINT('Origin',(315.981976869642,-19.47200726879,420.251347131769));
#57148=CARTESIAN_POINT('',(327.607283666135,-19.47200726879,446.055332241801));
#57149=CARTESIAN_POINT('Origin',(312.29935291193,-19.47200726879,476.437331203026));
#57150=CARTESIAN_POINT('',(327.193299517722,-19.47200726879,452.371509792254));
#57151=CARTESIAN_POINT('',(327.193299517722,-19.47200726879,452.371509792254));
#57152=CARTESIAN_POINT('Origin',(312.29935291193,-19.47200726879,476.437331203026));
#57153=CARTESIAN_POINT('Origin',(263.115917770968,-19.47200726879,445.000000551893));
#57154=CARTESIAN_POINT('',(322.049147324138,-19.47200726879,442.104796637205));
#57155=CARTESIAN_POINT('',(322.049147324138,-19.47200726879,442.104796637205));
#57156=CARTESIAN_POINT('',(321.922865318306,-19.47200726879,440.178105546934));
#57157=CARTESIAN_POINT('Origin',(263.115917770968,-19.47200726879,445.000000551893));
#57158=CARTESIAN_POINT('',(321.922865318306,-19.47200726879,440.178105546934));
#57159=CARTESIAN_POINT('Origin',(312.29935291193,-19.47200726879,413.56266990076));
#57160=CARTESIAN_POINT('',(327.193299517722,-19.47200726879,437.628491311531));
#57161=CARTESIAN_POINT('Origin',(312.29935291193,-19.47200726879,413.56266990076));
#57162=CARTESIAN_POINT('',(327.193299517722,-19.47200726879,437.628491311531));
#57163=CARTESIAN_POINT('Origin',(315.981976869642,-19.47200726879,469.748653972016));
#57164=CARTESIAN_POINT('',(327.607283666135,-19.47200726879,443.944668861984));
#57165=CARTESIAN_POINT('',(327.607283666135,-19.47200726879,443.944668861984));
#57166=CARTESIAN_POINT('Origin',(315.981976869642,-19.47200726879,469.748653972016));
#57167=CARTESIAN_POINT('Origin',(263.115917770968,-19.47200726879,445.000000551893));
#57168=CARTESIAN_POINT('',(321.167065432937,-19.47200726879,434.43723545924));
#57169=CARTESIAN_POINT('',(321.167065432937,-19.47200726879,434.43723545924));
#57170=CARTESIAN_POINT('',(320.790380135574,-19.47200726879,432.543510587704));
#57171=CARTESIAN_POINT('Origin',(263.115917770968,-19.47200726879,445.000000551893));
#57172=CARTESIAN_POINT('',(320.790380135574,-19.47200726879,432.543510587704));
#57173=CARTESIAN_POINT('Origin',(307.775186742732,-19.47200726879,407.411894113266));
#57174=CARTESIAN_POINT('',(325.682933602016,-19.47200726879,429.327778948132));
#57175=CARTESIAN_POINT('Origin',(307.775186742732,-19.47200726879,407.411894113266));
#57176=CARTESIAN_POINT('',(325.682933602016,-19.47200726879,429.327778948132));
#57177=CARTESIAN_POINT('Origin',(318.760047898935,-19.47200726879,462.636520419365));
#57178=CARTESIAN_POINT('',(326.917802663696,-19.47200726879,435.535884949522));
#57179=CARTESIAN_POINT('',(326.917802663696,-19.47200726879,435.535884949522));
#57180=CARTESIAN_POINT('Origin',(318.760047898935,-19.47200726879,462.636520419365));
#57181=CARTESIAN_POINT('Origin',(263.115917770968,-19.47200726879,445.000000551893));
#57182=CARTESIAN_POINT('',(319.29171231042,-19.47200726879,426.950406120563));
#57183=CARTESIAN_POINT('',(319.29171231042,-19.47200726879,426.950406120563));
#57184=CARTESIAN_POINT('',(318.671068911401,-19.47200726879,425.122049625353));
#57185=CARTESIAN_POINT('Origin',(263.115917770968,-19.47200726879,445.000000551893));
#57186=CARTESIAN_POINT('',(318.671068911401,-19.47200726879,425.122049625353));
#57187=CARTESIAN_POINT('Origin',(302.486888099538,-19.47200726879,401.904261248329));
#57188=CARTESIAN_POINT('',(323.102028698587,-19.47200726879,421.295222641534));
#57189=CARTESIAN_POINT('Origin',(302.486888099538,-19.47200726879,401.904261248329));
#57190=CARTESIAN_POINT('',(323.102028698587,-19.47200726879,421.295222641534));
#57191=CARTESIAN_POINT('Origin',(320.586032434271,-19.47200726879,455.222621122015));
#57192=CARTESIAN_POINT('',(325.136653721519,-19.47200726879,427.289034678965));
#57193=CARTESIAN_POINT('',(325.136653721519,-19.47200726879,427.289034678965));
#57194=CARTESIAN_POINT('Origin',(320.586032434271,-19.47200726879,455.222621122015));
#57195=CARTESIAN_POINT('Origin',(263.115917770968,-19.47200726879,445.000000551893));
#57196=CARTESIAN_POINT('',(316.455175768461,-19.47200726879,419.772410346899));
#57197=CARTESIAN_POINT('',(316.455175768461,-19.47200726879,419.772410346899));
#57198=CARTESIAN_POINT('',(315.601193648417,-19.47200726879,418.040705914564));
#57199=CARTESIAN_POINT('Origin',(263.115917770968,-19.47200726879,445.000000551893));
#57200=CARTESIAN_POINT('',(315.601193648417,-19.47200726879,418.040705914564));
#57201=CARTESIAN_POINT('Origin',(296.524941238327,-19.4720072687899,397.134008431272));
#57202=CARTESIAN_POINT('',(319.494744805894,-19.47200726879,413.668261657189));
#57203=CARTESIAN_POINT('Origin',(296.524941238327,-19.4720072687899,397.134008431272));
#57204=CARTESIAN_POINT('',(319.494744805894,-19.47200726879,413.668261657189));
#57205=CARTESIAN_POINT('Origin',(321.428687373992,-19.47200726879,447.633809952464));
#57206=CARTESIAN_POINT('',(322.294312791831,-19.47200726879,419.345223944901));
#57207=CARTESIAN_POINT('',(322.294312791831,-19.47200726879,419.345223944901));
#57208=CARTESIAN_POINT('Origin',(321.428687373992,-19.47200726879,447.633809952464));
#57209=CARTESIAN_POINT('Origin',(263.115917770968,-19.47200726879,445.000000551893));
#57210=CARTESIAN_POINT('',(312.705989733729,-19.47200726879,413.026065636052));
#57211=CARTESIAN_POINT('',(312.705989733729,-19.47200726879,413.026065636052));
#57212=CARTESIAN_POINT('',(311.633280763503,-19.47200726879,411.420643209548));
#57213=CARTESIAN_POINT('Origin',(263.115917770968,-19.47200726879,445.000000551893));
#57214=CARTESIAN_POINT('',(311.633280763503,-19.47200726879,411.420643209548));
#57215=CARTESIAN_POINT('Origin',(289.991356722859,-19.4720072687899,393.18275601036));
#57216=CARTESIAN_POINT('',(314.92280355147,-19.47200726879,406.577395412131));
#57217=CARTESIAN_POINT('Origin',(289.991356722859,-19.4720072687899,393.18275601036));
#57218=CARTESIAN_POINT('',(314.92280355147,-19.47200726879,406.577395412131));
#57219=CARTESIAN_POINT('Origin',(321.273594658451,-19.47200726879,439.999933573839));
#57220=CARTESIAN_POINT('',(318.439413115985,-19.47200726879,411.84037355143));
#57221=CARTESIAN_POINT('',(318.439413115985,-19.47200726879,411.84037355143));
#57222=CARTESIAN_POINT('Origin',(321.273594658451,-19.47200726879,439.999933573839));
#57223=CARTESIAN_POINT('Origin',(263.115917770968,-19.47200726879,445.000000551893));
#57224=CARTESIAN_POINT('',(308.108303818748,-19.47200726879,406.826803816464));
#57225=CARTESIAN_POINT('',(308.108303818748,-19.47200726879,406.826803816464));
#57226=CARTESIAN_POINT('',(306.835222346232,-19.47200726879,405.375132618617));
#57227=CARTESIAN_POINT('Origin',(263.115917770968,-19.47200726879,445.000000551893));
#57228=CARTESIAN_POINT('',(306.835222346232,-19.47200726879,405.375132618617));
#57229=CARTESIAN_POINT('Origin',(282.997925995644,-19.4720072687899,390.118111010007));
#57230=CARTESIAN_POINT('',(309.464432117758,-19.47200726879,400.143950593773));
#57231=CARTESIAN_POINT('Origin',(282.997925995644,-19.4720072687899,390.118111010007));
#57232=CARTESIAN_POINT('',(309.464432117758,-19.47200726879,400.143950593773));
#57233=CARTESIAN_POINT('Origin',(320.123407967011,-19.47200726879,432.451609727489));
#57234=CARTESIAN_POINT('',(313.637913096216,-19.47200726879,404.902893569523));
#57235=CARTESIAN_POINT('',(313.637913096216,-19.47200726879,404.902893569523));
#57236=CARTESIAN_POINT('Origin',(320.123407967011,-19.47200726879,432.451609727489));
#57237=CARTESIAN_POINT('Origin',(263.115917770968,-19.47200726879,445.000000551893));
#57238=CARTESIAN_POINT('',(302.740785704244,-19.4720072687899,401.280695976629));
#57239=CARTESIAN_POINT('',(302.740785704244,-19.4720072687899,401.280695976629));
#57240=CARTESIAN_POINT('',(301.289114506397,-19.4720072687899,400.007614504112));
#57241=CARTESIAN_POINT('Origin',(263.115917770968,-19.47200726879,445.000000551893));
#57242=CARTESIAN_POINT('',(301.289114506397,-19.4720072687899,400.007614504112));
#57243=CARTESIAN_POINT('Origin',(275.664308595371,-19.4720072687899,387.99251035585));
#57244=CARTESIAN_POINT('',(303.213024753338,-19.4720072687899,394.478005226645));
#57245=CARTESIAN_POINT('Origin',(275.664308595371,-19.4720072687899,387.99251035585));
#57246=CARTESIAN_POINT('',(303.213024753338,-19.4720072687899,394.478005226645));
#57247=CARTESIAN_POINT('Origin',(317.997807312854,-19.47200726879,425.117992327216));
#57248=CARTESIAN_POINT('',(307.971967729088,-19.4720072687899,398.651486205102));
#57249=CARTESIAN_POINT('',(307.971967729088,-19.4720072687899,398.651486205102));
#57250=CARTESIAN_POINT('Origin',(317.997807312854,-19.47200726879,425.117992327216));
#57251=CARTESIAN_POINT('Origin',(263.115917770968,-19.47200726879,445.000000551893));
#57252=CARTESIAN_POINT('',(296.695275113313,-19.4720072687899,396.482637559358));
#57253=CARTESIAN_POINT('',(296.695275113313,-19.4720072687899,396.482637559358));
#57254=CARTESIAN_POINT('',(295.089852686809,-19.4720072687899,395.409928589132));
#57255=CARTESIAN_POINT('Origin',(263.115917770968,-19.47200726879,445.000000551893));
#57256=CARTESIAN_POINT('',(295.089852686809,-19.4720072687899,395.409928589132));
#57257=CARTESIAN_POINT('Origin',(268.115984749021,-19.4720072687899,386.84232366441));
#57258=CARTESIAN_POINT('',(296.275544771431,-19.4720072687899,389.676505206875));
#57259=CARTESIAN_POINT('Origin',(268.115984749021,-19.4720072687899,386.84232366441));
#57260=CARTESIAN_POINT('',(296.275544771431,-19.4720072687899,389.676505206875));
#57261=CARTESIAN_POINT('Origin',(314.933162312501,-19.47200726879,418.124561600002));
#57262=CARTESIAN_POINT('',(301.53852291073,-19.4720072687899,393.193114771391));
#57263=CARTESIAN_POINT('',(301.53852291073,-19.4720072687899,393.193114771391));
#57264=CARTESIAN_POINT('Origin',(314.933162312501,-19.47200726879,418.124561600002));
#57265=CARTESIAN_POINT('Origin',(263.115917770968,-19.47200726879,445.000000551893));
#57266=CARTESIAN_POINT('',(290.075212408297,-19.4720072687899,392.514724674444));
#57267=CARTESIAN_POINT('',(290.075212408297,-19.4720072687899,392.514724674444));
#57268=CARTESIAN_POINT('',(288.343507975962,-19.4720072687899,391.6607425544));
#57269=CARTESIAN_POINT('Origin',(263.115917770968,-19.47200726879,445.000000551893));
#57270=CARTESIAN_POINT('',(288.343507975962,-19.4720072687899,391.6607425544));
#57271=CARTESIAN_POINT('Origin',(260.482108370397,-19.4720072687899,386.687230948869));
#57272=CARTESIAN_POINT('',(288.77069437796,-19.4720072687899,385.82160553103));
#57273=CARTESIAN_POINT('Origin',(260.482108370397,-19.4720072687899,386.687230948869));
#57274=CARTESIAN_POINT('',(288.77069437796,-19.4720072687899,385.82160553103));
#57275=CARTESIAN_POINT('Origin',(310.981909891589,-19.47200726879,411.590977084533));
#57276=CARTESIAN_POINT('',(294.447656665672,-19.4720072687899,388.621173516967));
#57277=CARTESIAN_POINT('',(294.447656665672,-19.4720072687899,388.621173516967));
#57278=CARTESIAN_POINT('Origin',(310.981909891589,-19.47200726879,411.590977084533));
#57279=CARTESIAN_POINT('Origin',(263.115917770968,-19.47200726879,445.000000551893));
#57280=CARTESIAN_POINT('',(282.993868697508,-19.4720072687899,389.44484941146));
#57281=CARTESIAN_POINT('',(282.993868697508,-19.4720072687899,389.44484941146));
#57282=CARTESIAN_POINT('',(281.165512202297,-19.4720072687899,388.82420601244));
#57283=CARTESIAN_POINT('Origin',(263.115917770968,-19.47200726879,445.000000551893));
#57284=CARTESIAN_POINT('',(281.165512202297,-19.4720072687899,388.82420601244));
#57285=CARTESIAN_POINT('Origin',(252.893297200845,-19.4720072687899,387.52988588859));
#57286=CARTESIAN_POINT('',(280.826883643896,-19.4720072687899,382.979264601342));
#57287=CARTESIAN_POINT('Origin',(252.893297200845,-19.4720072687899,387.52988588859));
#57288=CARTESIAN_POINT('',(280.826883643896,-19.4720072687899,382.979264601342));
#57289=CARTESIAN_POINT('Origin',(306.211657074532,-19.47200726879,405.629030223323));
#57290=CARTESIAN_POINT('',(286.820695681326,-19.4720072687899,385.013889624274));
#57291=CARTESIAN_POINT('',(286.820695681326,-19.4720072687899,385.013889624274));
#57292=CARTESIAN_POINT('Origin',(306.211657074532,-19.47200726879,405.629030223323));
#57293=CARTESIAN_POINT('Origin',(263.115917770968,-19.47200726879,445.000000551893));
#57294=CARTESIAN_POINT('',(275.572407735156,-19.4720072687899,387.325538187287));
#57295=CARTESIAN_POINT('',(275.572407735156,-19.4720072687899,387.325538187287));
#57296=CARTESIAN_POINT('',(273.67868286362,-19.4720072687899,386.948852889924));
#57297=CARTESIAN_POINT('Origin',(263.115917770968,-19.47200726879,445.000000551893));
#57298=CARTESIAN_POINT('',(273.67868286362,-19.4720072687899,386.948852889924));
#57299=CARTESIAN_POINT('Origin',(245.479397903495,-19.4720072687899,389.355870423926));
#57300=CARTESIAN_POINT('',(272.580033373339,-19.4720072687899,381.198115659165));
#57301=CARTESIAN_POINT('Origin',(245.479397903495,-19.4720072687899,389.355870423926));
#57302=CARTESIAN_POINT('',(272.580033373339,-19.4720072687899,381.198115659165));
#57303=CARTESIAN_POINT('Origin',(300.704024209595,-19.4720072687899,400.340731580129));
#57304=CARTESIAN_POINT('',(278.788139374728,-19.4720072687899,382.432984720845));
#57305=CARTESIAN_POINT('',(278.788139374728,-19.4720072687899,382.432984720845));
#57306=CARTESIAN_POINT('Origin',(300.704024209595,-19.4720072687899,400.340731580129));
#57307=CARTESIAN_POINT('Origin',(263.115917770968,-19.47200726879,445.000000551893));
#57308=CARTESIAN_POINT('',(267.937812775926,-19.4720072687899,386.193053004555));
#57309=CARTESIAN_POINT('',(267.937812775926,-19.4720072687899,386.193053004555));
#57310=CARTESIAN_POINT('',(266.011121685656,-19.4720072687899,386.066770998723));
#57311=CARTESIAN_POINT('Origin',(263.115917770968,-19.47200726879,445.000000551893));
#57312=CARTESIAN_POINT('',(266.011121685656,-19.4720072687899,386.066770998723));
#57313=CARTESIAN_POINT('Origin',(238.367264350844,-19.4720072687899,392.133941453219));
#57314=CARTESIAN_POINT('',(264.171249460876,-19.4720072687899,380.508634656726));
#57315=CARTESIAN_POINT('Origin',(238.367264350844,-19.4720072687899,392.133941453219));
#57316=CARTESIAN_POINT('',(264.171249460876,-19.4720072687899,380.508634656726));
#57317=CARTESIAN_POINT('Origin',(294.553248422101,-19.4720072687899,395.816565410931));
#57318=CARTESIAN_POINT('',(270.487427011329,-19.4720072687899,380.922618805139));
#57319=CARTESIAN_POINT('',(270.487427011329,-19.4720072687899,380.922618805139));
#57320=CARTESIAN_POINT('Origin',(294.553248422101,-19.4720072687899,395.816565410931));
#57321=CARTESIAN_POINT('Origin',(263.115917770968,-19.47200726879,445.000000551893));
#57322=CARTESIAN_POINT('',(260.22071385628,-19.4720072687899,386.066770998723));
#57323=CARTESIAN_POINT('',(260.22071385628,-19.4720072687899,386.066770998723));
#57324=CARTESIAN_POINT('',(258.294022766009,-19.4720072687899,386.193053004555));
#57325=CARTESIAN_POINT('Origin',(263.115917770968,-19.47200726879,445.000000551893));
#57326=CARTESIAN_POINT('',(258.294022766009,-19.4720072687899,386.193053004555));
#57327=CARTESIAN_POINT('Origin',(231.678587119835,-19.4720072687899,395.816565410931));
#57328=CARTESIAN_POINT('',(255.744408530606,-19.4720072687899,380.922618805139));
#57329=CARTESIAN_POINT('Origin',(231.678587119835,-19.4720072687899,395.816565410931));
#57330=CARTESIAN_POINT('',(255.744408530606,-19.4720072687899,380.922618805139));
#57331=CARTESIAN_POINT('Origin',(287.864571191091,-19.4720072687899,392.133941453219));
#57332=CARTESIAN_POINT('',(262.060586081059,-19.4720072687899,380.508634656726));
#57333=CARTESIAN_POINT('',(262.060586081059,-19.4720072687899,380.508634656726));
#57334=CARTESIAN_POINT('Origin',(287.864571191091,-19.4720072687899,392.133941453219));
#57335=CARTESIAN_POINT('Origin',(263.115917770968,-19.47200726879,445.000000551893));
#57336=CARTESIAN_POINT('',(252.553152678315,-19.4720072687899,386.948852889924));
#57337=CARTESIAN_POINT('',(252.553152678315,-19.4720072687899,386.948852889924));
#57338=CARTESIAN_POINT('',(250.659427806779,-19.4720072687899,387.325538187287));
#57339=CARTESIAN_POINT('Origin',(263.115917770968,-19.47200726879,445.000000551893));
#57340=CARTESIAN_POINT('',(250.659427806779,-19.4720072687899,387.325538187287));
#57341=CARTESIAN_POINT('Origin',(225.527811332341,-19.4720072687899,400.340731580129));
#57342=CARTESIAN_POINT('',(247.443696167207,-19.4720072687899,382.432984720845));
#57343=CARTESIAN_POINT('Origin',(225.527811332341,-19.4720072687899,400.340731580129));
#57344=CARTESIAN_POINT('',(247.443696167207,-19.4720072687899,382.432984720845));
#57345=CARTESIAN_POINT('Origin',(280.75243763844,-19.4720072687899,389.355870423926));
#57346=CARTESIAN_POINT('',(253.651802168597,-19.4720072687899,381.198115659165));
#57347=CARTESIAN_POINT('',(253.651802168597,-19.4720072687899,381.198115659165));
#57348=CARTESIAN_POINT('Origin',(280.75243763844,-19.4720072687899,389.355870423926));
#57349=CARTESIAN_POINT('Origin',(263.115917770968,-19.47200726879,445.000000551893));
#57350=CARTESIAN_POINT('',(245.066323339638,-19.4720072687899,388.824206012441));
#57351=CARTESIAN_POINT('',(245.066323339638,-19.4720072687899,388.824206012441));
#57352=CARTESIAN_POINT('',(243.237966844428,-19.4720072687899,389.44484941146));
#57353=CARTESIAN_POINT('Origin',(263.115917770968,-19.47200726879,445.000000551893));
#57354=CARTESIAN_POINT('',(243.237966844428,-19.4720072687899,389.44484941146));
#57355=CARTESIAN_POINT('Origin',(220.020178467404,-19.4720072687899,405.629030223323));
#57356=CARTESIAN_POINT('',(239.411139860609,-19.4720072687899,385.013889624274));
#57357=CARTESIAN_POINT('Origin',(220.020178467404,-19.4720072687899,405.629030223323));
#57358=CARTESIAN_POINT('',(239.411139860609,-19.4720072687899,385.013889624274));
#57359=CARTESIAN_POINT('Origin',(273.33853834109,-19.4720072687899,387.52988588859));
#57360=CARTESIAN_POINT('',(245.40495189804,-19.4720072687899,382.979264601342));
#57361=CARTESIAN_POINT('',(245.40495189804,-19.4720072687899,382.979264601342));
#57362=CARTESIAN_POINT('Origin',(273.33853834109,-19.4720072687899,387.52988588859));
#57363=CARTESIAN_POINT('Origin',(263.115917770968,-19.47200726879,445.000000551893));
#57364=CARTESIAN_POINT('',(237.888327565974,-19.4720072687899,391.6607425544));
#57365=CARTESIAN_POINT('',(237.888327565974,-19.4720072687899,391.6607425544));
#57366=CARTESIAN_POINT('',(236.156623133639,-19.4720072687899,392.514724674444));
#57367=CARTESIAN_POINT('Origin',(263.115917770968,-19.47200726879,445.000000551893));
#57368=CARTESIAN_POINT('',(236.156623133639,-19.4720072687899,392.514724674444));
#57369=CARTESIAN_POINT('Origin',(215.249925650347,-19.4720072687899,411.590977084534));
#57370=CARTESIAN_POINT('',(231.784178876264,-19.4720072687899,388.621173516967));
#57371=CARTESIAN_POINT('Origin',(215.249925650347,-19.4720072687899,411.590977084534));
#57372=CARTESIAN_POINT('',(231.784178876264,-19.4720072687899,388.621173516967));
#57373=CARTESIAN_POINT('Origin',(265.749727171539,-19.4720072687899,386.687230948869));
#57374=CARTESIAN_POINT('',(237.461141163976,-19.4720072687899,385.82160553103));
#57375=CARTESIAN_POINT('',(237.461141163976,-19.4720072687899,385.82160553103));
#57376=CARTESIAN_POINT('Origin',(265.749727171539,-19.4720072687899,386.687230948869));
#57377=CARTESIAN_POINT('Origin',(263.115917770968,-19.47200726879,445.000000551893));
#57378=CARTESIAN_POINT('',(231.141982855127,-19.4720072687899,395.409928589132));
#57379=CARTESIAN_POINT('',(231.141982855127,-19.4720072687899,395.409928589132));
#57380=CARTESIAN_POINT('',(229.536560428623,-19.4720072687899,396.482637559359));
#57381=CARTESIAN_POINT('Origin',(263.115917770968,-19.47200726879,445.000000551893));
#57382=CARTESIAN_POINT('',(229.536560428623,-19.4720072687899,396.482637559359));
#57383=CARTESIAN_POINT('Origin',(211.298673229435,-19.4720072687899,418.124561600002));
#57384=CARTESIAN_POINT('',(224.693312631206,-19.4720072687899,393.193114771392));
#57385=CARTESIAN_POINT('Origin',(211.298673229435,-19.4720072687899,418.124561600002));
#57386=CARTESIAN_POINT('',(224.693312631206,-19.4720072687899,393.193114771392));
#57387=CARTESIAN_POINT('Origin',(258.115850792914,-19.4720072687899,386.84232366441));
#57388=CARTESIAN_POINT('',(229.956290770505,-19.4720072687899,389.676505206876));
#57389=CARTESIAN_POINT('',(229.956290770505,-19.4720072687899,389.676505206876));
#57390=CARTESIAN_POINT('Origin',(258.115850792914,-19.4720072687899,386.84232366441));
#57391=CARTESIAN_POINT('Origin',(263.115917770968,-19.47200726879,445.000000551893));
#57392=CARTESIAN_POINT('',(224.942721035539,-19.4720072687899,400.007614504113));
#57393=CARTESIAN_POINT('',(224.942721035539,-19.4720072687899,400.007614504113));
#57394=CARTESIAN_POINT('',(223.491049837692,-19.4720072687899,401.280695976629));
#57395=CARTESIAN_POINT('Origin',(263.115917770968,-19.47200726879,445.000000551893));
#57396=CARTESIAN_POINT('',(223.491049837692,-19.4720072687899,401.280695976629));
#57397=CARTESIAN_POINT('Origin',(208.234028229082,-19.4720072687899,425.117992327217));
#57398=CARTESIAN_POINT('',(218.259867812848,-19.4720072687899,398.651486205103));
#57399=CARTESIAN_POINT('Origin',(208.234028229082,-19.4720072687899,425.117992327217));
#57400=CARTESIAN_POINT('',(218.259867812848,-19.4720072687899,398.651486205103));
#57401=CARTESIAN_POINT('Origin',(250.567526946564,-19.4720072687899,387.99251035585));
#57402=CARTESIAN_POINT('',(223.018810788598,-19.4720072687899,394.478005226645));
#57403=CARTESIAN_POINT('',(223.018810788598,-19.4720072687899,394.478005226645));
#57404=CARTESIAN_POINT('Origin',(250.567526946564,-19.4720072687899,387.99251035585));
#57405=CARTESIAN_POINT('Origin',(263.115917770968,-19.47200726879,445.000000551893));
#57406=CARTESIAN_POINT('',(219.396613195704,-19.4720072687899,405.375132618617));
#57407=CARTESIAN_POINT('',(219.396613195704,-19.4720072687899,405.375132618617));
#57408=CARTESIAN_POINT('',(218.123531723188,-19.4720072687899,406.826803816464));
#57409=CARTESIAN_POINT('Origin',(263.115917770968,-19.47200726879,445.000000551893));
#57410=CARTESIAN_POINT('',(218.123531723188,-19.4720072687899,406.826803816464));
#57411=CARTESIAN_POINT('Origin',(206.108427574925,-19.4720072687899,432.45160972749));
#57412=CARTESIAN_POINT('',(212.59392244572,-19.4720072687899,404.902893569523));
#57413=CARTESIAN_POINT('Origin',(206.108427574925,-19.4720072687899,432.45160972749));
#57414=CARTESIAN_POINT('',(212.59392244572,-19.4720072687899,404.902893569523));
#57415=CARTESIAN_POINT('Origin',(243.233909546291,-19.4720072687899,390.118111010007));
#57416=CARTESIAN_POINT('',(216.767403424177,-19.4720072687899,400.143950593773));
#57417=CARTESIAN_POINT('',(216.767403424177,-19.4720072687899,400.143950593773));
#57418=CARTESIAN_POINT('Origin',(243.233909546291,-19.4720072687899,390.118111010007));
#57419=CARTESIAN_POINT('Origin',(263.115917770968,-19.47200726879,445.000000551893));
#57420=CARTESIAN_POINT('',(214.598554778433,-19.4720072687899,411.420643209549));
#57421=CARTESIAN_POINT('',(214.598554778433,-19.4720072687899,411.420643209549));
#57422=CARTESIAN_POINT('',(213.525845808207,-19.4720072687899,413.026065636052));
#57423=CARTESIAN_POINT('Origin',(263.115917770968,-19.47200726879,445.000000551893));
#57424=CARTESIAN_POINT('',(213.525845808207,-19.4720072687899,413.026065636052));
#57425=CARTESIAN_POINT('Origin',(204.958240883485,-19.47200726879,439.99993357384));
#57426=CARTESIAN_POINT('',(207.79242242595,-19.4720072687899,411.840373551431));
#57427=CARTESIAN_POINT('Origin',(204.958240883485,-19.47200726879,439.99993357384));
#57428=CARTESIAN_POINT('',(207.79242242595,-19.4720072687899,411.840373551431));
#57429=CARTESIAN_POINT('Origin',(236.240478819077,-19.4720072687899,393.18275601036));
#57430=CARTESIAN_POINT('',(211.309031990466,-19.4720072687899,406.577395412131));
#57431=CARTESIAN_POINT('',(211.309031990466,-19.4720072687899,406.577395412131));
#57432=CARTESIAN_POINT('Origin',(236.240478819077,-19.4720072687899,393.18275601036));
#57433=CARTESIAN_POINT('Origin',(263.115917770968,-19.47200726879,445.000000551893));
#57434=CARTESIAN_POINT('',(210.630641893519,-19.4720072687899,418.040705914564));
#57435=CARTESIAN_POINT('',(210.630641893519,-19.4720072687899,418.040705914564));
#57436=CARTESIAN_POINT('',(209.776659773475,-19.4720072687899,419.7724103469));
#57437=CARTESIAN_POINT('Origin',(263.115917770968,-19.47200726879,445.000000551893));
#57438=CARTESIAN_POINT('',(209.776659773475,-19.4720072687899,419.7724103469));
#57439=CARTESIAN_POINT('Origin',(204.803148167944,-19.47200726879,447.633809952465));
#57440=CARTESIAN_POINT('',(203.937522750105,-19.4720072687899,419.345223944901));
#57441=CARTESIAN_POINT('Origin',(204.803148167944,-19.47200726879,447.633809952465));
#57442=CARTESIAN_POINT('',(203.937522750105,-19.4720072687899,419.345223944901));
#57443=CARTESIAN_POINT('Origin',(229.706894303608,-19.4720072687899,397.134008431273));
#57444=CARTESIAN_POINT('',(206.737090736042,-19.4720072687899,413.668261657189));
#57445=CARTESIAN_POINT('',(206.737090736042,-19.4720072687899,413.668261657189));
#57446=CARTESIAN_POINT('Origin',(229.706894303608,-19.4720072687899,397.134008431273));
#57447=CARTESIAN_POINT('Origin',(263.115917770968,-19.47200726879,445.000000551893));
#57448=CARTESIAN_POINT('',(207.560766630535,-19.4720072687899,425.122049625353));
#57449=CARTESIAN_POINT('',(207.560766630535,-19.4720072687899,425.122049625353));
#57450=CARTESIAN_POINT('',(206.940123231516,-19.4720072687899,426.950406120564));
#57451=CARTESIAN_POINT('Origin',(263.115917770968,-19.47200726879,445.000000551893));
#57452=CARTESIAN_POINT('',(206.940123231516,-19.4720072687899,426.950406120564));
#57453=CARTESIAN_POINT('Origin',(205.645803107665,-19.47200726879,455.222621122016));
#57454=CARTESIAN_POINT('',(201.095181820417,-19.4720072687899,427.289034678965));
#57455=CARTESIAN_POINT('Origin',(205.645803107665,-19.47200726879,455.222621122016));
#57456=CARTESIAN_POINT('',(201.095181820417,-19.4720072687899,427.289034678965));
#57457=CARTESIAN_POINT('Origin',(223.744947442398,-19.4720072687899,401.904261248329));
#57458=CARTESIAN_POINT('',(203.129806843349,-19.4720072687899,421.295222641535));
#57459=CARTESIAN_POINT('',(203.129806843349,-19.4720072687899,421.295222641535));
#57460=CARTESIAN_POINT('Origin',(223.744947442398,-19.4720072687899,401.904261248329));
#57461=CARTESIAN_POINT('Origin',(263.115917770968,-19.47200726879,445.000000551893));
#57462=CARTESIAN_POINT('',(205.441455406362,-19.4720072687899,432.543510587705));
#57463=CARTESIAN_POINT('',(205.441455406362,-19.4720072687899,432.543510587705));
#57464=CARTESIAN_POINT('',(205.064770108999,-19.47200726879,434.437235459241));
#57465=CARTESIAN_POINT('Origin',(263.115917770968,-19.47200726879,445.000000551893));
#57466=CARTESIAN_POINT('',(205.064770108999,-19.47200726879,434.437235459241));
#57467=CARTESIAN_POINT('Origin',(207.471787643001,-19.47200726879,462.636520419366));
#57468=CARTESIAN_POINT('',(199.31403287824,-19.47200726879,435.535884949523));
#57469=CARTESIAN_POINT('Origin',(207.471787643001,-19.47200726879,462.636520419366));
#57470=CARTESIAN_POINT('',(199.31403287824,-19.47200726879,435.535884949522));
#57471=CARTESIAN_POINT('Origin',(218.456648799204,-19.4720072687899,407.411894113266));
#57472=CARTESIAN_POINT('',(200.54890193992,-19.4720072687899,429.327778948133));
#57473=CARTESIAN_POINT('',(200.54890193992,-19.4720072687899,429.327778948133));
#57474=CARTESIAN_POINT('Origin',(218.456648799204,-19.4720072687899,407.411894113266));
#57475=CARTESIAN_POINT('Origin',(263.115917770968,-19.47200726879,445.000000551893));
#57476=CARTESIAN_POINT('',(204.30897022363,-19.47200726879,440.178105546935));
#57477=CARTESIAN_POINT('',(204.30897022363,-19.47200726879,440.178105546935));
#57478=CARTESIAN_POINT('',(204.182688217798,-19.47200726879,442.104796637205));
#57479=CARTESIAN_POINT('Origin',(263.115917770968,-19.47200726879,445.000000551893));
#57480=CARTESIAN_POINT('',(204.182688217798,-19.47200726879,442.104796637205));
#57481=CARTESIAN_POINT('Origin',(210.249858672294,-19.47200726879,469.748653972017));
#57482=CARTESIAN_POINT('',(198.624551875801,-19.47200726879,443.944668861985));
#57483=CARTESIAN_POINT('Origin',(210.249858672294,-19.47200726879,469.748653972017));
#57484=CARTESIAN_POINT('',(198.624551875801,-19.47200726879,443.944668861985));
#57485=CARTESIAN_POINT('Origin',(213.932482630006,-19.4720072687899,413.56266990076));
#57486=CARTESIAN_POINT('',(199.038536024214,-19.47200726879,437.628491311532));
#57487=CARTESIAN_POINT('',(199.038536024214,-19.47200726879,437.628491311532));
#57488=CARTESIAN_POINT('Origin',(213.932482630006,-19.4720072687899,413.56266990076));
#57489=CARTESIAN_POINT('Origin',(263.115917770968,-19.47200726879,445.000000551893));
#57490=CARTESIAN_POINT('',(198.624551875801,-19.47200726879,446.055332241802));
#57491=CARTESIAN_POINT('Origin',(263.115917770968,-19.47200726879,445.000000551893));
#57492=CARTESIAN_POINT('',(198.624551875801,-19.47200726879,446.055332241802));
#57493=CARTESIAN_POINT('Origin',(263.115917770968,-19.47200726879,445.000000551893));
#57494=CARTESIAN_POINT('Origin',(263.115917770968,-19.47200726879,445.000000551893));
#57495=CARTESIAN_POINT('Origin',(263.115917770968,-19.47200726879,445.000000551893));
#57496=CARTESIAN_POINT('Origin',(263.115917770968,-19.47200726879,445.000000551893));
#57497=CARTESIAN_POINT('Origin',(263.115917770968,-19.47200726879,445.000000551893));
#57498=CARTESIAN_POINT('Origin',(263.115917770968,-19.47200726879,445.000000551893));
#57499=CARTESIAN_POINT('Origin',(263.115917770968,-19.47200726879,445.000000551893));
#57500=CARTESIAN_POINT('Origin',(263.115917770968,-19.47200726879,445.000000551893));
#57501=CARTESIAN_POINT('Origin',(263.115917770968,-19.47200726879,445.000000551893));
#57502=CARTESIAN_POINT('Origin',(263.115917770968,-19.47200726879,445.000000551893));
#57503=CARTESIAN_POINT('Origin',(263.115917770968,-19.47200726879,445.000000551893));
#57504=CARTESIAN_POINT('Origin',(263.115917770968,-19.47200726879,445.000000551893));
#57505=CARTESIAN_POINT('Origin',(263.115917770968,-19.47200726879,445.000000551893));
#57506=CARTESIAN_POINT('Origin',(263.115917770968,-19.47200726879,445.000000551893));
#57507=CARTESIAN_POINT('Origin',(263.115917770968,-19.47200726879,445.000000551893));
#57508=CARTESIAN_POINT('Origin',(263.115917770968,-19.47200726879,445.000000551893));
#57509=CARTESIAN_POINT('Origin',(263.115917770968,-19.47200726879,445.000000551893));
#57510=CARTESIAN_POINT('Origin',(263.115917770968,-19.47200726879,445.000000551893));
#57511=CARTESIAN_POINT('Origin',(263.115917770968,-19.47200726879,445.000000551893));
#57512=CARTESIAN_POINT('Origin',(263.115917770968,-19.47200726879,445.000000551893));
#57513=CARTESIAN_POINT('Origin',(263.115917770968,-19.47200726879,445.000000551893));
#57514=CARTESIAN_POINT('Origin',(263.115917770968,-19.47200726879,445.000000551893));
#57515=CARTESIAN_POINT('Origin',(263.115917770968,-19.47200726879,445.000000551893));
#57516=CARTESIAN_POINT('Origin',(263.115917770968,-19.47200726879,445.000000551893));
#57517=CARTESIAN_POINT('Origin',(263.115917770968,-19.47200726879,445.000000551893));
#57518=CARTESIAN_POINT('Origin',(263.115917770968,-19.47200726879,445.000000551893));
#57519=CARTESIAN_POINT('Origin',(263.115917770968,-19.47200726879,445.000000551893));
#57520=CARTESIAN_POINT('Origin',(263.115917770968,-19.47200726879,445.000000551893));
#57521=CARTESIAN_POINT('Origin',(263.115917770968,-19.47200726879,445.000000551893));
#57522=CARTESIAN_POINT('Origin',(263.115917770968,-19.47200726879,445.000000551893));
#57523=CARTESIAN_POINT('Origin',(263.115917770968,-19.47200726879,445.000000551893));
#57524=CARTESIAN_POINT('Origin',(263.115917770968,-19.47200726879,445.000000551893));
#57525=CARTESIAN_POINT('Origin',(263.115917770968,-19.47200726879,445.000000551893));
#57526=CARTESIAN_POINT('Origin',(263.115917770968,-19.47200726879,445.000000551893));
#57527=CARTESIAN_POINT('Origin',(263.115917770968,-19.47200726879,445.000000551893));
#57528=CARTESIAN_POINT('Origin',(263.115917770968,-19.47200726879,445.000000551893));
#57529=CARTESIAN_POINT('Origin',(263.115917770968,-19.47200726879,445.000000551893));
#57530=CARTESIAN_POINT('Origin',(263.115917770968,-19.47200726879,445.000000551893));
#57531=CARTESIAN_POINT('Origin',(263.115917770968,-19.47200726879,445.000000551893));
#57532=CARTESIAN_POINT('Origin',(263.115917770968,-19.47200726879,445.000000551893));
#57533=CARTESIAN_POINT('Origin',(263.115917770968,-19.47200726879,445.000000551893));
#57534=CARTESIAN_POINT('Origin',(263.115917770968,-19.47200726879,445.000000551893));
#57535=CARTESIAN_POINT('Origin',(263.115917770968,-19.47200726879,445.000000551893));
#57536=CARTESIAN_POINT('Origin',(263.115917770968,-19.47200726879,445.000000551893));
#57537=CARTESIAN_POINT('Origin',(263.115917770968,-19.47200726879,445.000000551893));
#57538=CARTESIAN_POINT('Origin',(263.115917770968,-19.47200726879,445.000000551893));
#57539=CARTESIAN_POINT('Origin',(263.115917770968,-19.47200726879,445.000000551893));
#57540=CARTESIAN_POINT('Origin',(263.115917770968,-19.47200726879,445.000000551893));
#57541=CARTESIAN_POINT('Origin',(263.115917770968,-19.47200726879,445.000000551893));
#57542=CARTESIAN_POINT('Origin',(263.115917770968,-19.47200726879,445.000000551893));
#57543=CARTESIAN_POINT('Origin',(263.115917770968,-19.47200726879,445.000000551893));
#57544=CARTESIAN_POINT('Origin',(263.115917770968,-19.47200726879,445.000000551893));
#57545=CARTESIAN_POINT('Origin',(263.115917770968,-19.47200726879,445.000000551893));
#57546=CARTESIAN_POINT('Origin',(263.115917770968,-19.47200726879,445.000000551893));
#57547=CARTESIAN_POINT('Origin',(263.115917770968,-19.47200726879,445.000000551893));
#57548=CARTESIAN_POINT('Origin',(263.115917770968,-19.47200726879,445.000000551893));
#57549=CARTESIAN_POINT('Origin',(263.115917770968,-19.47200726879,445.000000551893));
#57550=CARTESIAN_POINT('Origin',(263.115917770968,-19.47200726879,445.000000551893));
#57551=CARTESIAN_POINT('Origin',(263.115917770968,-19.47200726879,445.000000551893));
#57552=CARTESIAN_POINT('Origin',(263.115917770968,-19.47200726879,445.000000551893));
#57553=CARTESIAN_POINT('Origin',(263.115917770968,-19.47200726879,445.000000551893));
#57554=CARTESIAN_POINT('Origin',(263.115917770968,-19.47200726879,445.000000551893));
#57555=CARTESIAN_POINT('Origin',(263.115917770968,-19.47200726879,445.000000551893));
#57556=CARTESIAN_POINT('Origin',(263.115917770968,-19.47200726879,445.000000551893));
#57557=CARTESIAN_POINT('Origin',(263.115917770968,-19.47200726879,445.000000551893));
#57558=CARTESIAN_POINT('Origin',(263.115917770968,-19.47200726879,445.000000551893));
#57559=CARTESIAN_POINT('Origin',(263.115917770968,-19.47200726879,445.000000551893));
#57560=CARTESIAN_POINT('Origin',(263.115917770968,-19.47200726879,445.000000551893));
#57561=CARTESIAN_POINT('Origin',(263.115917770968,-19.47200726879,445.000000551893));
#57562=CARTESIAN_POINT('Origin',(263.115917770968,-19.47200726879,445.000000551893));
#57563=CARTESIAN_POINT('Origin',(263.115917770968,-19.47200726879,445.000000551893));
#57564=CARTESIAN_POINT('Origin',(263.115917770968,-19.47200726879,445.000000551893));
#57565=CARTESIAN_POINT('Origin',(263.115917770968,-19.47200726879,445.000000551893));
#57566=CARTESIAN_POINT('Origin',(263.115917770968,-19.47200726879,445.000000551893));
#57567=CARTESIAN_POINT('Origin',(263.115917770968,-19.47200726879,445.000000551893));
#57568=CARTESIAN_POINT('Origin',(263.115917770968,-19.47200726879,445.000000551893));
#57569=CARTESIAN_POINT('Origin',(263.115917770968,-19.47200726879,445.000000551893));
#57570=CARTESIAN_POINT('Origin',(263.115917770968,-19.47200726879,445.000000551893));
#57571=CARTESIAN_POINT('Origin',(263.115917770968,-19.47200726879,445.000000551893));
#57572=CARTESIAN_POINT('Origin',(263.115917770968,-19.47200726879,445.000000551893));
#57573=CARTESIAN_POINT('Origin',(263.115917770968,-19.47200726879,445.000000551893));
#57574=CARTESIAN_POINT('Origin',(263.115917770968,-19.47200726879,445.000000551893));
#57575=CARTESIAN_POINT('Origin',(263.115917770968,-19.47200726879,445.000000551893));
#57576=CARTESIAN_POINT('Origin',(263.115917770968,-19.47200726879,445.000000551893));
#57577=CARTESIAN_POINT('Origin',(263.115917770968,-19.47200726879,445.000000551893));
#57578=CARTESIAN_POINT('Origin',(263.115917770968,-19.47200726879,445.000000551893));
#57579=CARTESIAN_POINT('Origin',(263.115917770968,-19.47200726879,445.000000551893));
#57580=CARTESIAN_POINT('Origin',(263.115917770968,-19.47200726879,445.000000551893));
#57581=CARTESIAN_POINT('Origin',(263.115917770968,-19.47200726879,445.000000551893));
#57582=CARTESIAN_POINT('Origin',(263.115917770968,-19.47200726879,445.000000551893));
#57583=CARTESIAN_POINT('Origin',(263.115917770968,-19.47200726879,445.000000551893));
#57584=CARTESIAN_POINT('Origin',(263.115917770968,-19.47200726879,445.000000551893));
#57585=CARTESIAN_POINT('Origin',(263.115917770968,-19.47200726879,445.000000551893));
#57586=CARTESIAN_POINT('',(204.182688217798,-19.47200726879,447.895204466582));
#57587=CARTESIAN_POINT('',(204.182688217798,-19.47200726879,447.895204466582));
#57588=CARTESIAN_POINT('',(204.30897022363,-19.47200726879,449.821895556852));
#57589=CARTESIAN_POINT('Origin',(263.115917770968,-19.47200726879,445.000000551893));
#57590=CARTESIAN_POINT('',(204.30897022363,-19.47200726879,449.821895556852));
#57591=CARTESIAN_POINT('Origin',(213.932482630006,-19.47200726879,476.437331203026));
#57592=CARTESIAN_POINT('',(199.038536024214,-19.47200726879,452.371509792255));
#57593=CARTESIAN_POINT('Origin',(213.932482630006,-19.47200726879,476.437331203026));
#57594=CARTESIAN_POINT('',(199.038536024214,-19.47200726879,452.371509792255));
#57595=CARTESIAN_POINT('Origin',(210.249858672294,-19.4720072687899,420.25134713177));
#57596=CARTESIAN_POINT('Origin',(210.249858672294,-19.4720072687899,420.25134713177));
#57597=CARTESIAN_POINT('Origin',(263.115917770968,-19.47200726879,445.000000551893));
#57598=CARTESIAN_POINT('Origin',(263.115917770968,-19.47200726879,445.000000551893));
#57599=CARTESIAN_POINT('Origin',(263.115917770968,-19.47200726879,445.000000551893));
#61775=UNCERTAINTY_MEASURE_WITH_UNIT(LENGTH_MEASURE(0.01),#61812,
'DISTANCE_ACCURACY_VALUE',
'Maximum model space distance between geometric entities at asserted c
onnectivities');
#61780=UNCERTAINTY_MEASURE_WITH_UNIT(LENGTH_MEASURE(0.01),#61812,
'DISTANCE_ACCURACY_VALUE',
'Maximum model space distance between geometric entities at asserted c
onnectivities');
#61806=(
GEOMETRIC_REPRESENTATION_CONTEXT(3)
GLOBAL_UNCERTAINTY_ASSIGNED_CONTEXT((#61775))
GLOBAL_UNIT_ASSIGNED_CONTEXT((#61812,#61814,#61815))
REPRESENTATION_CONTEXT('','3D')
);
#61811=(
GEOMETRIC_REPRESENTATION_CONTEXT(3)
GLOBAL_UNCERTAINTY_ASSIGNED_CONTEXT((#61780))
GLOBAL_UNIT_ASSIGNED_CONTEXT((#61812,#61814,#61815))
REPRESENTATION_CONTEXT('','3D')
);
#61812=(
LENGTH_UNIT()
NAMED_UNIT(*)
SI_UNIT(.MILLI.,.METRE.)
);
#61814=(
NAMED_UNIT(*)
PLANE_ANGLE_UNIT()
SI_UNIT($,.RADIAN.)
);
#61815=(
NAMED_UNIT(*)
SI_UNIT($,.STERADIAN.)
SOLID_ANGLE_UNIT()
);
#61841=SHAPE_DEFINITION_REPRESENTATION(#61903,#61993);
#61903=PRODUCT_DEFINITION_SHAPE('',$,#62024);
#61993=SHAPE_REPRESENTATION('',(#36148),#61806);
#61998=PRODUCT_DEFINITION_CONTEXT('part definition',#62090,'design');
#62024=PRODUCT_DEFINITION('Large Spur Gear','Large Spur Gear',#62054,#61998);
#62054=PRODUCT_DEFINITION_FORMATION('',$,#62117);
#62090=APPLICATION_CONTEXT('Managed model based 3d engineering');
#62091=PRODUCT_CONTEXT('part definition',#62090,'mechanical');
#62117=PRODUCT('Large Spur Gear','Large Spur Gear',$,(#62091));
#62143=COLOUR_RGB('Sky Blue',0.24,0.69,0.87);
#62144=FILL_AREA_STYLE_COLOUR('',#62143);
#62145=FILL_AREA_STYLE('',(#62144));
#62146=SURFACE_STYLE_FILL_AREA(#62145);
#62147=SURFACE_SIDE_STYLE('',(#62146));
#62148=SURFACE_STYLE_USAGE(.BOTH.,#62147);
#62149=PRESENTATION_STYLE_ASSIGNMENT((#62148));
ENDSEC;
END-ISO-10303-21;
